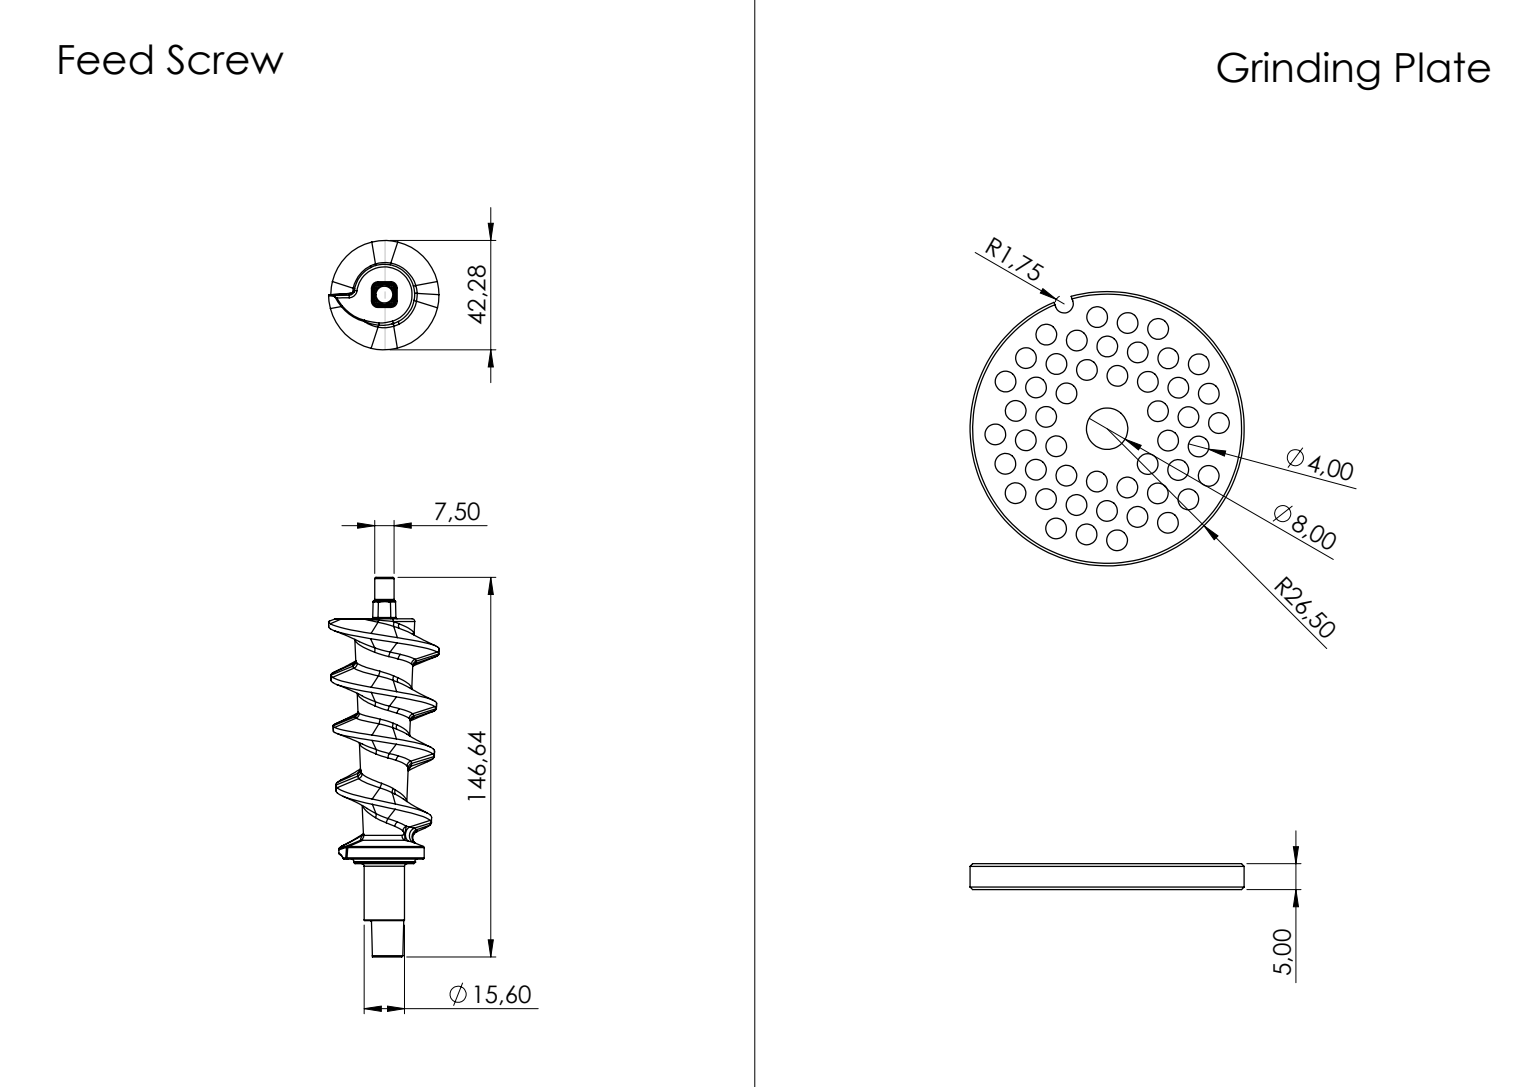
ISO-10303-21;
HEADER;
FILE_DESCRIPTION (('STEP AP214'),
    '1' );
FILE_NAME ('Grinding Plate.step',
    '2026-10-06T09:49:54',
    ( '' ),
    ( '' ),
    'SwSTEP 2.0',
    'SolidWorks 2020',
    '' );
FILE_SCHEMA (( 'AUTOMOTIVE_DESIGN' ));
ENDSEC;

DATA;
#6=DIRECTION ( 'NONE',  ( -0.6736849260863841948, 0.000000000000000000, 0.7390186874254148774 ) ) ;
#19=DIRECTION ( 'NONE',  ( 0.9858563016923833633, 0.000000000000000000, 0.1675928173085483863 ) ) ;
#20=ORIENTED_EDGE ( 'NONE', *, *, #50403, .T. ) ;
#27=ORIENTED_EDGE ( 'NONE', *, *, #23843, .F. ) ;
#32=EDGE_CURVE ( 'NONE', #37900, #21516, #96808, .T. ) ;
#63=CYLINDRICAL_SURFACE ( 'NONE', #4748, 2.000000000000003553 ) ;
#99=DIRECTION ( 'NONE',  ( 0.9858563016923833633, 0.000000000000000000, 0.1675928173085483863 ) ) ;
#119=DIRECTION ( 'NONE',  ( -5.980589973904019347E-17, 1.000000000000000000, -1.736889445713099699E-16 ) ) ;
#130=DIRECTION ( 'NONE',  ( -0.6736849260863839728, 0.000000000000000000, 0.7390186874254150995 ) ) ;
#163=CARTESIAN_POINT ( 'NONE',  ( -6.501609782144661231, 1517.151704408390060, 200.8207946853451631 ) ) ;
#210=FACE_BOUND ( 'NONE', #98928, .T. ) ;
#217=EDGE_LOOP ( 'NONE', ( #25668, #43396, #24555, #73471 ) ) ;
#228=DIRECTION ( 'NONE',  ( -0.6736849260863839728, 0.000000000000000000, 0.7390186874254150995 ) ) ;
#238=EDGE_CURVE ( 'NONE', #55027, #57510, #22026, .T. ) ;
#241=CARTESIAN_POINT ( 'NONE',  ( -9.862951377749247683, 1522.051704408389924, 228.3939896778649654 ) ) ;
#262=DIRECTION ( 'NONE',  ( 1.755985294532464991E-16, -1.000000000000000000, 1.338183447452830017E-16 ) ) ;
#294=CARTESIAN_POINT ( 'NONE',  ( -19.66678637224480397, 1519.551704408389924, 215.8936635741279986 ) ) ;
#310=CARTESIAN_POINT ( 'NONE',  ( -19.02974267272306719, 1517.051704408389924, 207.1627782414018100 ) ) ;
#365=VERTEX_POINT ( 'NONE', #20997 ) ;
#367=AXIS2_PLACEMENT_3D ( 'NONE', #81942, #5812, #24233 ) ;
#373=FACE_OUTER_BOUND ( 'NONE', #57009, .T. ) ;
#399=EDGE_CURVE ( 'NONE', #104547, #81525, #8616, .T. ) ;
#413=CARTESIAN_POINT ( 'NONE',  ( -6.954065720117950100, 1517.051704408389924, 183.5505540514350002 ) ) ;
#427=DIRECTION ( 'NONE',  ( -0.6736849260863839728, 0.000000000000000000, 0.7390186874254150995 ) ) ;
#428=DIRECTION ( 'NONE',  ( -1.755985294532469921E-16, 1.000000000000000000, -1.338183447452831989E-16 ) ) ;
#451=EDGE_LOOP ( 'NONE', ( #81291, #94235, #88373, #80457, #8593 ) ) ;
#471=AXIS2_PLACEMENT_3D ( 'NONE', #413, #34530, #58646 ) ;
#507=CARTESIAN_POINT ( 'NONE',  ( -9.786977751178733698, 1521.951704408389787, 191.2793932888540951 ) ) ;
#512=DIRECTION ( 'NONE',  ( -1.964544591288419982E-14, -1.000000000000000000, 8.043425993822650894E-15 ) ) ;
#532=DIRECTION ( 'NONE',  ( 0.9858563016923833633, 0.000000000000000000, 0.1675928173085483863 ) ) ;
#595=ORIENTED_EDGE ( 'NONE', *, *, #3501, .F. ) ;
#597=CARTESIAN_POINT ( 'NONE',  ( -7.271052316819549333, 1522.051704408389924, 225.3404165491008371 ) ) ;
#600=ORIENTED_EDGE ( 'NONE', *, *, #74040, .T. ) ;
#619=ORIENTED_EDGE ( 'NONE', *, *, #18010, .T. ) ;
#620=ADVANCED_FACE ( 'NONE', ( #78041 ), #85891, .F. ) ;
#634=SHAPE_DEFINITION_REPRESENTATION ( #5341, #72299 ) ;
#648=FACE_OUTER_BOUND ( 'NONE', #91311, .T. ) ;
#709=EDGE_CURVE ( 'NONE', #103300, #104414, #52050, .T. ) ;
#711=EDGE_CURVE ( 'NONE', #77569, #52731, #30620, .T. ) ;
#721=DIRECTION ( 'NONE',  ( 5.980589973904019347E-17, -1.000000000000000000, 1.736889445713099699E-16 ) ) ;
#743=DIRECTION ( 'NONE',  ( 1.755985294532469921E-16, -1.000000000000000000, 1.338183447452831989E-16 ) ) ;
#746=VECTOR ( 'NONE', #79973, 1000.000000000000000 ) ;
#771=ADVANCED_FACE ( 'NONE', ( #97611 ), #2481, .F. ) ;
#806=LINE ( 'NONE', #8072, #30643 ) ;
#832=EDGE_CURVE ( 'NONE', #43055, #13291, #18048, .T. ) ;
#860=AXIS2_PLACEMENT_3D ( 'NONE', #53375, #104309, #3530 ) ;
#871=VECTOR ( 'NONE', #57828, 1000.000000000000000 ) ;
#886=FACE_BOUND ( 'NONE', #41380, .T. ) ;
#910=ORIENTED_EDGE ( 'NONE', *, *, #106899, .T. ) ;
#914=CIRCLE ( 'NONE', #22271, 1.999999999999997780 ) ;
#999=ORIENTED_EDGE ( 'NONE', *, *, #53098, .T. ) ;
#1004=VERTEX_POINT ( 'NONE', #56242 ) ;
#1012=DIRECTION ( 'NONE',  ( -5.980589973904019347E-17, 1.000000000000000000, -1.736889445713099699E-16 ) ) ;
#1044=ORIENTED_EDGE ( 'NONE', *, *, #84247, .F. ) ;
#1077=VERTEX_POINT ( 'NONE', #18891 ) ;
#1134=EDGE_LOOP ( 'NONE', ( #19550, #98250, #54353, #73848 ) ) ;
#1145=EDGE_CURVE ( 'NONE', #38215, #32285, #36581, .T. ) ;
#1157=CYLINDRICAL_SURFACE ( 'NONE', #96556, 2.000000000000003553 ) ;
#1167=CARTESIAN_POINT ( 'NONE',  ( 3.897009773650441211, 1519.551704408389924, 231.0205787112126075 ) ) ;
#1269=LINE ( 'NONE', #35408, #31651 ) ;
#1351=DIRECTION ( 'NONE',  ( -1.755985294532469921E-16, 1.000000000000000000, -1.338183447452831989E-16 ) ) ;
#1368=CIRCLE ( 'NONE', #63973, 1.999999999999997780 ) ;
#1416=VECTOR ( 'NONE', #69193, 1000.000000000000000 ) ;
#1425=ORIENTED_EDGE ( 'NONE', *, *, #92483, .T. ) ;
#1443=VECTOR ( 'NONE', #3619, 1000.000000000000000 ) ;
#1447=VECTOR ( 'NONE', #59102, 1000.000000000000000 ) ;
#1455=CIRCLE ( 'NONE', #51483, 1.999999999999997780 ) ;
#1474=DIRECTION ( 'NONE',  ( -0.6736849260863841948, 0.000000000000000000, 0.7390186874254148774 ) ) ;
#1490=VERTEX_POINT ( 'NONE', #17960 ) ;
#1505=DIRECTION ( 'NONE',  ( -0.9455185755993178454, 0.000000000000000000, 0.3255681544571539243 ) ) ;
#1524=DIRECTION ( 'NONE',  ( 0.9455185755993178454, 0.000000000000000000, -0.3255681544571537578 ) ) ;
#1534=DIRECTION ( 'NONE',  ( 0.9858563016923833633, 0.000000000000000000, 0.1675928173085483863 ) ) ;
#1548=DIRECTION ( 'NONE',  ( 0.9455185755993178454, 0.000000000000000000, -0.3255681544571537578 ) ) ;
#1552=DIRECTION ( 'NONE',  ( -1.755985294532469921E-16, 1.000000000000000000, -1.338183447452831989E-16 ) ) ;
#1577=CARTESIAN_POINT ( 'NONE',  ( -11.81780673814840021, 1517.051704408389924, 222.7166774759110126 ) ) ;
#1585=VERTEX_POINT ( 'NONE', #48716 ) ;
#1595=CYLINDRICAL_SURFACE ( 'NONE', #11642, 2.000000000000003553 ) ;
#1596=DIRECTION ( 'NONE',  ( -0.6736849260863841948, 0.000000000000000000, 0.7390186874254148774 ) ) ;
#1633=DIRECTION ( 'NONE',  ( -0.6736849260863841948, 0.000000000000000000, 0.7390186874254148774 ) ) ;
#1642=DIRECTION ( 'NONE',  ( -1.755985294532469921E-16, 1.000000000000000000, -1.338183447452831989E-16 ) ) ;
#1649=EDGE_LOOP ( 'NONE', ( #99391, #52672, #101833, #73552 ) ) ;
#1650=DIRECTION ( 'NONE',  ( 1.755985294532469921E-16, -1.000000000000000000, 1.338183447452831989E-16 ) ) ;
#1667=CIRCLE ( 'NONE', #48101, 1.999999999999998668 ) ;
#1720=CARTESIAN_POINT ( 'NONE',  ( -15.69795926999090163, 1517.151704408390060, 195.4758181584410011 ) ) ;
#1747=EDGE_CURVE ( 'NONE', #43414, #35107, #74345, .T. ) ;
#1792=CARTESIAN_POINT ( 'NONE',  ( -21.63849897568203673, 1519.551704408389924, 215.5584779398195678 ) ) ;
#1822=AXIS2_PLACEMENT_3D ( 'NONE', #75535, #15573, #83352 ) ;
#1827=ORIENTED_EDGE ( 'NONE', *, *, #23117, .T. ) ;
#1848=CIRCLE ( 'NONE', #64422, 1.999999999999998668 ) ;
#1850=DIRECTION ( 'NONE',  ( -0.9455185755993178454, 0.000000000000000000, 0.3255681544571537578 ) ) ;
#1859=DIRECTION ( 'NONE',  ( -1.755985294532469921E-16, 1.000000000000000000, -1.338183447452831989E-16 ) ) ;
#1860=CONICAL_SURFACE ( 'NONE', #23233, 1.000000000000007327, 0.7853981633970000820 ) ;
#1868=AXIS2_PLACEMENT_3D ( 'NONE', #1577, #95621, #69899 ) ;
#1956=CARTESIAN_POINT ( 'NONE',  ( 21.62164173326539895, 1519.551704408389924, 208.0273405521070060 ) ) ;
#1961=CIRCLE ( 'NONE', #12873, 1.999999999999998668 ) ;
#1962=DIRECTION ( 'NONE',  ( -1.755985294532464991E-16, 1.000000000000000000, -1.338183447452830017E-16 ) ) ;
#1983=ORIENTED_EDGE ( 'NONE', *, *, #38974, .T. ) ;
#2000=ORIENTED_EDGE ( 'NONE', *, *, #5665, .F. ) ;
#2045=CIRCLE ( 'NONE', #64625, 2.000000000000003109 ) ;
#2052=ORIENTED_EDGE ( 'NONE', *, *, #13448, .F. ) ;
#2076=DIRECTION ( 'NONE',  ( 1.755985294532469921E-16, -1.000000000000000000, 1.338183447452831989E-16 ) ) ;
#2089=LINE ( 'NONE', #96684, #8615 ) ;
#2115=ORIENTED_EDGE ( 'NONE', *, *, #100899, .T. ) ;
#2153=ORIENTED_EDGE ( 'NONE', *, *, #64701, .T. ) ;
#2167=CIRCLE ( 'NONE', #36115, 1.999999999999998668 ) ;
#2172=ORIENTED_EDGE ( 'NONE', *, *, #97884, .T. ) ;
#2221=ADVANCED_FACE ( 'NONE', ( #43767 ), #11279, .F. ) ;
#2241=DIRECTION ( 'NONE',  ( -5.980589973904019347E-17, 1.000000000000000000, -1.736889445713099699E-16 ) ) ;
#2299=DIRECTION ( 'NONE',  ( -1.755985294532469921E-16, 1.000000000000000000, -1.338183447452831989E-16 ) ) ;
#2301=DIRECTION ( 'NONE',  ( -1.755985294532469921E-16, 1.000000000000000000, -1.338183447452831989E-16 ) ) ;
#2318=ADVANCED_FACE ( 'NONE', ( #87286 ), #107382, .F. ) ;
#2344=EDGE_CURVE ( 'NONE', #57510, #28393, #37987, .T. ) ;
#2356=ORIENTED_EDGE ( 'NONE', *, *, #32389, .T. ) ;
#2362=CARTESIAN_POINT ( 'NONE',  ( 10.47043688597563182, 1522.051704408389924, 197.0050518223378333 ) ) ;
#2378=DIRECTION ( 'NONE',  ( -0.6736849260863839728, 0.000000000000000000, 0.7390186874254150995 ) ) ;
#2384=EDGE_CURVE ( 'NONE', #41410, #69866, #97870, .T. ) ;
#2437=CYLINDRICAL_SURFACE ( 'NONE', #49131, 1.999999999999999556 ) ;
#2454=ORIENTED_EDGE ( 'NONE', *, *, #62551, .F. ) ;
#2468=ORIENTED_EDGE ( 'NONE', *, *, #61058, .F. ) ;
#2475=DIRECTION ( 'NONE',  ( 5.980589973904019347E-17, -1.000000000000000000, 1.736889445713099699E-16 ) ) ;
#2481=CYLINDRICAL_SURFACE ( 'NONE', #3800, 2.000000000000003109 ) ;
#2520=ORIENTED_EDGE ( 'NONE', *, *, #7279, .T. ) ;
#2526=DIRECTION ( 'NONE',  ( -0.6736849260863841948, 0.000000000000000000, 0.7390186874254148774 ) ) ;
#2578=ORIENTED_EDGE ( 'NONE', *, *, #35703, .F. ) ;
#2593=ORIENTED_EDGE ( 'NONE', *, *, #108261, .T. ) ;
#2596=CIRCLE ( 'NONE', #93734, 1.999999999999998668 ) ;
#2628=ORIENTED_EDGE ( 'NONE', *, *, #102846, .F. ) ;
#2629=DIRECTION ( 'NONE',  ( -1.755985294532469921E-16, 1.000000000000000000, -1.338183447452831989E-16 ) ) ;
#2630=DIRECTION ( 'NONE',  ( -5.980589973904019347E-17, 1.000000000000000000, -1.736889445713099699E-16 ) ) ;
#2644=ORIENTED_EDGE ( 'NONE', *, *, #20930, .T. ) ;
#2683=AXIS2_PLACEMENT_3D ( 'NONE', #72839, #63899, #54407 ) ;
#2689=DIRECTION ( 'NONE',  ( -1.755985294532469921E-16, 1.000000000000000000, -1.338183447452831989E-16 ) ) ;
#2707=FACE_OUTER_BOUND ( 'NONE', #62290, .T. ) ;
#2741=CARTESIAN_POINT ( 'NONE',  ( -5.940539704407486354, 1521.951704408389787, 229.2045057395878871 ) ) ;
#2743=ORIENTED_EDGE ( 'NONE', *, *, #15924, .T. ) ;
#2746=EDGE_CURVE ( 'NONE', #82445, #48574, #85257, .T. ) ;
#2764=VECTOR ( 'NONE', #6624, 1000.000000000000000 ) ;
#2798=ORIENTED_EDGE ( 'NONE', *, *, #52789, .T. ) ;
#2799=AXIS2_PLACEMENT_3D ( 'NONE', #81723, #3960, #12877 ) ;
#2807=CARTESIAN_POINT ( 'NONE',  ( 7.271052316819548444, 1522.051704408389924, 192.9032753742981470 ) ) ;
#2884=DIRECTION ( 'NONE',  ( 0.9858563016923833633, 0.000000000000000000, 0.1675928173085483863 ) ) ;
#2950=AXIS2_PLACEMENT_3D ( 'NONE', #40990, #76253, #75169 ) ;
#2955=CARTESIAN_POINT ( 'NONE',  ( -2.621457251404222255, 1519.551704408389924, 228.0616540033011574 ) ) ;
#2971=EDGE_CURVE ( 'NONE', #6947, #108856, #31094, .T. ) ;
#2988=EDGE_CURVE ( 'NONE', #20697, #36071, #48476, .T. ) ;
#3048=CARTESIAN_POINT ( 'NONE',  ( -21.60894078472486868, 1517.051704408389924, 199.6722430288449175 ) ) ;
#3095=CARTESIAN_POINT ( 'NONE',  ( -2.562340869413342048, 1522.051704408389924, 196.2891841806521711 ) ) ;
#3099=CIRCLE ( 'NONE', #17334, 1.999999999999999556 ) ;
#3107=VERTEX_POINT ( 'NONE', #106040 ) ;
#3128=ORIENTED_EDGE ( 'NONE', *, *, #24699, .T. ) ;
#3139=EDGE_CURVE ( 'NONE', #70769, #106306, #40471, .T. ) ;
#3155=CIRCLE ( 'NONE', #72836, 1.999999999999998668 ) ;
#3177=VECTOR ( 'NONE', #85229, 1000.000000000000000 ) ;
#3203=CIRCLE ( 'NONE', #6681, 1.999999999999999556 ) ;
#3222=ORIENTED_EDGE ( 'NONE', *, *, #102846, .T. ) ;
#3264=ORIENTED_EDGE ( 'NONE', *, *, #59650, .F. ) ;
#3450=DIRECTION ( 'NONE',  ( 1.755985294532469921E-16, -1.000000000000000000, 1.338183447452831989E-16 ) ) ;
#3455=DIRECTION ( 'NONE',  ( -0.6736849260863841948, 0.000000000000000000, 0.7390186874254148774 ) ) ;
#3468=AXIS2_PLACEMENT_3D ( 'NONE', #34859, #94767, #69046 ) ;
#3471=CYLINDRICAL_SURFACE ( 'NONE', #29822, 1.999999999999999556 ) ;
#3472=FACE_OUTER_BOUND ( 'NONE', #58106, .T. ) ;
#3501=EDGE_CURVE ( 'NONE', #90277, #63160, #6599, .T. ) ;
#3530=DIRECTION ( 'NONE',  ( -0.6736849260863841948, 0.000000000000000000, 0.7390186874254148774 ) ) ;
#3536=AXIS2_PLACEMENT_3D ( 'NONE', #106492, #105958, #29236 ) ;
#3552=ORIENTED_EDGE ( 'NONE', *, *, #50922, .F. ) ;
#3619=DIRECTION ( 'NONE',  ( -1.755985294532469921E-16, 1.000000000000000000, -1.338183447452831989E-16 ) ) ;
#3648=EDGE_CURVE ( 'NONE', #55027, #58309, #2089, .T. ) ;
#3657=EDGE_CURVE ( 'NONE', #3107, #87558, #71252, .T. ) ;
#3679=EDGE_LOOP ( 'NONE', ( #18940, #40964, #10687, #106527, #99518 ) ) ;
#3683=DIRECTION ( 'NONE',  ( -1.755985294532469921E-16, 1.000000000000000000, -1.338183447452831989E-16 ) ) ;
#3714=DIRECTION ( 'NONE',  ( -5.980589973904019347E-17, 1.000000000000000000, -1.736889445713099699E-16 ) ) ;
#3727=DIRECTION ( 'NONE',  ( -0.6736849260863839728, 0.000000000000000000, 0.7390186874254150995 ) ) ;
#3732=ORIENTED_EDGE ( 'NONE', *, *, #44116, .F. ) ;
#3738=AXIS2_PLACEMENT_3D ( 'NONE', #51329, #16589, #77104 ) ;
#3768=ADVANCED_FACE ( 'NONE', ( #87002 ), #11419, .F. ) ;
#3770=VERTEX_POINT ( 'NONE', #37164 ) ;
#3771=ORIENTED_EDGE ( 'NONE', *, *, #24131, .F. ) ;
#3777=EDGE_CURVE ( 'NONE', #20783, #98304, #62963, .T. ) ;
#3793=ORIENTED_EDGE ( 'NONE', *, *, #92766, .T. ) ;
#3794=ORIENTED_EDGE ( 'NONE', *, *, #5777, .T. ) ;
#3800=AXIS2_PLACEMENT_3D ( 'NONE', #88123, #46679, #72424 ) ;
#3804=DIRECTION ( 'NONE',  ( -0.6736849260863841948, 0.000000000000000000, 0.7390186874254148774 ) ) ;
#3812=ORIENTED_EDGE ( 'NONE', *, *, #98933, .F. ) ;
#3820=CARTESIAN_POINT ( 'NONE',  ( 11.75869035672759999, 1522.051704408389924, 227.2994842695800060 ) ) ;
#3826=ORIENTED_EDGE ( 'NONE', *, *, #68263, .F. ) ;
#3851=CARTESIAN_POINT ( 'NONE',  ( 15.69795926444620271, 1519.551704408389924, 222.7678737639049871 ) ) ;
#3893=CIRCLE ( 'NONE', #64637, 1.999999999999999556 ) ;
#3905=CARTESIAN_POINT ( 'NONE',  ( -9.803834995107230554, 1517.151704408390060, 196.6215198571080123 ) ) ;
#3914=EDGE_CURVE ( 'NONE', #42052, #70558, #6856, .T. ) ;
#3924=CARTESIAN_POINT ( 'NONE',  ( -7.878537825433329367, 1522.051704408389924, 218.1850669711710111 ) ) ;
#3955=VERTEX_POINT ( 'NONE', #1792 ) ;
#3956=AXIS2_PLACEMENT_3D ( 'NONE', #18061, #95892, #34874 ) ;
#3960=DIRECTION ( 'NONE',  ( 1.755985294532464991E-16, -1.000000000000000000, 1.338183447452830017E-16 ) ) ;
#3965=EDGE_LOOP ( 'NONE', ( #93778, #97741 ) ) ;
#3970=CIRCLE ( 'NONE', #14650, 2.000000000000003553 ) ;
#4069=EDGE_LOOP ( 'NONE', ( #72525, #55858, #37367, #105994, #72756 ) ) ;
#4131=CARTESIAN_POINT ( 'NONE',  ( 13.10606020890036838, 1522.051704408389924, 225.8214468947291493 ) ) ;
#4149=DIRECTION ( 'NONE',  ( -5.980589973904019347E-17, 1.000000000000000000, -1.736889445713099699E-16 ) ) ;
#4156=ORIENTED_EDGE ( 'NONE', *, *, #71920, .F. ) ;
#4223=DIRECTION ( 'NONE',  ( 1.755985294532469921E-16, -1.000000000000000000, 1.338183447452831989E-16 ) ) ;
#4248=FACE_OUTER_BOUND ( 'NONE', #102284, .T. ) ;
#4284=CIRCLE ( 'NONE', #32863, 1.999999999999999556 ) ;
#4287=DIRECTION ( 'NONE',  ( 5.980589973904019347E-17, -1.000000000000000000, 1.736889445713099699E-16 ) ) ;
#4305=VERTEX_POINT ( 'NONE', #28905 ) ;
#4328=ADVANCED_FACE ( 'NONE', ( #37307 ), #105058, .F. ) ;
#4340=ORIENTED_EDGE ( 'NONE', *, *, #37161, .T. ) ;
#4344=ORIENTED_EDGE ( 'NONE', *, *, #78141, .T. ) ;
#4386=CARTESIAN_POINT ( 'NONE',  ( -2.694739704345539888, 1517.151704408390060, 212.0779207114006510 ) ) ;
#4407=CARTESIAN_POINT ( 'NONE',  ( 7.271052316819548444, 1517.051704408389924, 192.9032753742981470 ) ) ;
#4486=DIRECTION ( 'NONE',  ( -1.755985294532469921E-16, 1.000000000000000000, -1.338183447452831989E-16 ) ) ;
#4521=DIRECTION ( 'NONE',  ( 5.980589973904019347E-17, -1.000000000000000000, 1.736889445713099699E-16 ) ) ;
#4577=CYLINDRICAL_SURFACE ( 'NONE', #87806, 2.000000000000003109 ) ;
#4600=ORIENTED_EDGE ( 'NONE', *, *, #107012, .F. ) ;
#4662=DIRECTION ( 'NONE',  ( 1.755985294532464991E-16, -1.000000000000000000, 1.338183447452830017E-16 ) ) ;
#4664=ORIENTED_EDGE ( 'NONE', *, *, #17540, .F. ) ;
#4694=CARTESIAN_POINT ( 'NONE',  ( 19.64992912776053657, 1517.051704408389924, 207.6921549199338983 ) ) ;
#4704=ORIENTED_EDGE ( 'NONE', *, *, #86424, .F. ) ;
#4735=DIRECTION ( 'NONE',  ( -0.9455185755993177343, 0.000000000000000000, 0.3255681544571540909 ) ) ;
#4745=CYLINDRICAL_SURFACE ( 'NONE', #5170, 2.000000000000003553 ) ;
#4748=AXIS2_PLACEMENT_3D ( 'NONE', #78412, #102486, #43707 ) ;
#4755=VERTEX_POINT ( 'NONE', #32752 ) ;
#4779=CARTESIAN_POINT ( 'NONE',  ( -9.862951377749247683, 1519.551704408389924, 228.3939896778649654 ) ) ;
#4781=CARTESIAN_POINT ( 'NONE',  ( 17.04532911661897288, 1517.151704408390060, 221.2898363890541589 ) ) ;
#4812=EDGE_CURVE ( 'NONE', #110694, #92620, #72829, .T. ) ;
#4830=ORIENTED_EDGE ( 'NONE', *, *, #2384, .F. ) ;
#4852=CYLINDRICAL_SURFACE ( 'NONE', #83731, 1.999999999999999556 ) ;
#4892=EDGE_LOOP ( 'NONE', ( #85187, #54785, #37181, #64258, #94394 ) ) ;
#4998=DIRECTION ( 'NONE',  ( -1.755985294532469921E-16, 1.000000000000000000, -1.338183447452831989E-16 ) ) ;
#5015=DIRECTION ( 'NONE',  ( 1.755985294532464991E-16, -1.000000000000000000, 1.338183447452830017E-16 ) ) ;
#5024=CARTESIAN_POINT ( 'NONE',  ( -20.98459803374076671, 1522.051704408389924, 201.4854660376508377 ) ) ;
#5026=VECTOR ( 'NONE', #83048, 1000.000000000000114 ) ;
#5071=DIRECTION ( 'NONE',  ( -5.980589973904019347E-17, 1.000000000000000000, -1.736889445713099699E-16 ) ) ;
#5075=EDGE_CURVE ( 'NONE', #8045, #31574, #41588, .T. ) ;
#5096=ORIENTED_EDGE ( 'NONE', *, *, #71920, .T. ) ;
#5103=CIRCLE ( 'NONE', #103491, 1.999999999999997780 ) ;
#5135=EDGE_CURVE ( 'NONE', #85592, #22264, #60356, .T. ) ;
#5144=EDGE_LOOP ( 'NONE', ( #76940, #42317, #64742, #2628, #47320 ) ) ;
#5162=VERTEX_POINT ( 'NONE', #106445 ) ;
#5168=DIRECTION ( 'NONE',  ( -5.980589973904019347E-17, 1.000000000000000000, -1.736889445713099699E-16 ) ) ;
#5170=AXIS2_PLACEMENT_3D ( 'NONE', #62071, #47861, #81434 ) ;
#5175=ADVANCED_FACE ( 'NONE', ( #72852 ), #46562, .F. ) ;
#5179=DIRECTION ( 'NONE',  ( -1.755985294532469921E-16, 1.000000000000000000, -1.338183447452831989E-16 ) ) ;
#5204=AXIS2_PLACEMENT_3D ( 'NONE', #24042, #8355, #68860 ) ;
#5231=DIRECTION ( 'NONE',  ( -1.755985294532469921E-16, 1.000000000000000000, -1.338183447452831989E-16 ) ) ;
#5240=CARTESIAN_POINT ( 'NONE',  ( -19.64992913029231403, 1519.551704408389924, 210.5515370058381279 ) ) ;
#5294=ORIENTED_EDGE ( 'NONE', *, *, #58517, .T. ) ;
#5341=PRODUCT_DEFINITION_SHAPE ( 'NONE', 'NONE',  #93161 ) ;
#5345=DIRECTION ( 'NONE',  ( 1.755985294532469921E-16, -1.000000000000000000, 1.338183447452831989E-16 ) ) ;
#5369=ORIENTED_EDGE ( 'NONE', *, *, #109924, .F. ) ;
#5372=DIRECTION ( 'NONE',  ( -1.755985294532469921E-16, 1.000000000000000000, -1.338183447452831989E-16 ) ) ;
#5486=EDGE_CURVE ( 'NONE', #81391, #100544, #1368, .T. ) ;
#5497=CARTESIAN_POINT ( 'NONE',  ( 5.923682464646780943, 1517.151704408390060, 194.3813127491490036 ) ) ;
#5506=DIRECTION ( 'NONE',  ( -1.755985294532469921E-16, 1.000000000000000000, -1.338183447452831989E-16 ) ) ;
#5562=CYLINDRICAL_SURFACE ( 'NONE', #30522, 2.000000000000003109 ) ;
#5599=CLOSED_SHELL ( 'NONE', ( #96938, #24061, #27007, #21181, #95044, #42222, #31748, #84990, #66105, #15986, #78832, #105611, #9693, #47464, #96441, #57134, #95527, #73378, #69362, #41149, #59645, #20154, #8989, #60806, #56963, #71224, #11391, #50751, #23310, #57672, #99363, #78459, #69555, #48000, #55987, #66999, #61806, #19362, #102319, #70587, #83469, #22197, #76059, #10075, #16727, #19263, #92537, #84237, #101278, #4328, #28941, #65806, #64116, #32565, #58366, #101310, #48745, #27494, #21540, #48765, #2318, #72324, #52788, #93107, #13462, #91394, #72125, #63168, #87992, #41597, #48623, #30912, #13186, #49423, #47605, #30257, #9196, #16734, #20439, #27756, #81449, #110377, #27011, #108348, #63755, #15866, #35213, #36382, #107664, #109982, #87124, #26759, #13816, #5175, #104836, #102164, #76276, #74830, #30311, #52793, #37664, #98830, #102964, #54643, #88843, #84779, #99574, #82543, #2221, #3768, #21272, #66596, #76262, #21664, #19989, #80982, #771, #15078, #88570, #77472, #85641, #58210, #97263, #97920, #32326, #620, #79124, #103589, #66134, #70497, #95510, #74653, #22326, #24667, #80630, #42693, #100116, #12589, #83130, #108285, #28154, #25589, #73272, #42319, #82177 ) ) ;
#5621=ORIENTED_EDGE ( 'NONE', *, *, #12480, .F. ) ;
#5646=FACE_OUTER_BOUND ( 'NONE', #74460, .T. ) ;
#5665=EDGE_CURVE ( 'NONE', #365, #93138, #21166, .T. ) ;
#5668=DIRECTION ( 'NONE',  ( -5.980589973904019347E-17, 1.000000000000000000, -1.736889445713099699E-16 ) ) ;
#5701=VECTOR ( 'NONE', #54056, 1000.000000000000000 ) ;
#5712=CARTESIAN_POINT ( 'NONE',  ( 18.31941652029302858, 1519.551704408389924, 203.8280657238408651 ) ) ;
#5718=CIRCLE ( 'NONE', #61218, 2.000000000000003553 ) ;
#5777=EDGE_CURVE ( 'NONE', #86539, #59011, #70285, .T. ) ;
#5812=DIRECTION ( 'NONE',  ( 1.755985294532469921E-16, -1.000000000000000000, 1.338183447452831989E-16 ) ) ;
#5815=AXIS2_PLACEMENT_3D ( 'NONE', #89895, #106692, #108911 ) ;
#5836=FACE_BOUND ( 'NONE', #97963, .T. ) ;
#5911=ORIENTED_EDGE ( 'NONE', *, *, #92691, .F. ) ;
#5918=( BOUNDED_CURVE ( )  B_SPLINE_CURVE ( 2, ( #99780, #55622, #89198 ),
 .UNSPECIFIED., .F., .T. ) 
 B_SPLINE_CURVE_WITH_KNOTS ( ( 3, 3 ),
 ( 0.1572692979053489926, 0.2337410564013850112 ),
 .UNSPECIFIED. ) 
 CURVE ( )  GEOMETRIC_REPRESENTATION_ITEM ( )  RATIONAL_B_SPLINE_CURVE ( ( 1.002044729868130091, 1.002448067003099963, 1.002760198777220113 ) ) 
 REPRESENTATION_ITEM ( '' )  );
#5929=CARTESIAN_POINT ( 'NONE',  ( 15.69795926444620271, 1519.551704408389924, 222.7678737639049871 ) ) ;
#5995=DIRECTION ( 'NONE',  ( -5.980589973904019347E-17, 1.000000000000000000, -1.736889445713099699E-16 ) ) ;
#5998=EDGE_LOOP ( 'NONE', ( #90814, #20701, #47201, #91238, #70087 ) ) ;
#6024=CYLINDRICAL_SURFACE ( 'NONE', #32104, 2.000000000000003553 ) ;
#6074=CARTESIAN_POINT ( 'NONE',  ( 5.864566082395450408, 1517.051704408389924, 226.1537825710409777 ) ) ;
#6086=CIRCLE ( 'NONE', #13177, 1.999999999999999556 ) ;
#6097=LINE ( 'NONE', #49227, #50092 ) ;
#6177=LINE ( 'NONE', #74511, #23361 ) ;
#6235=ORIENTED_EDGE ( 'NONE', *, *, #80260, .F. ) ;
#6266=EDGE_CURVE ( 'NONE', #64960, #108026, #19234, .T. ) ;
#6275=CIRCLE ( 'NONE', #68887, 1.999999999999999556 ) ;
#6349=LINE ( 'NONE', #90901, #52146 ) ;
#6419=VECTOR ( 'NONE', #67422, 1000.000000000000000 ) ;
#6420=ORIENTED_EDGE ( 'NONE', *, *, #107298, .T. ) ;
#6450=CARTESIAN_POINT ( 'NONE',  ( 2.562340869413348265, 1517.051704408389924, 221.9545077427458182 ) ) ;
#6458=EDGE_LOOP ( 'NONE', ( #60135, #15344, #107470, #40291, #89219, #32445 ) ) ;
#6526=AXIS2_PLACEMENT_3D ( 'NONE', #23608, #32574, #24142 ) ;
#6530=ORIENTED_EDGE ( 'NONE', *, *, #61639, .T. ) ;
#6537=DIRECTION ( 'NONE',  ( 5.980589973904019347E-17, -1.000000000000000000, 1.736889445713099699E-16 ) ) ;
#6541=ORIENTED_EDGE ( 'NONE', *, *, #93928, .F. ) ;
#6586=ORIENTED_EDGE ( 'NONE', *, *, #79455, .T. ) ;
#6592=CARTESIAN_POINT ( 'NONE',  ( 9.803834995107230554, 1517.151704408390060, 221.6221720662910002 ) ) ;
#6599=LINE ( 'NONE', #101185, #90869 ) ;
#6601=ORIENTED_EDGE ( 'NONE', *, *, #42077, .F. ) ;
#6617=EDGE_LOOP ( 'NONE', ( #84907, #22921 ) ) ;
#6624=DIRECTION ( 'NONE',  ( -1.755985294532469921E-16, 1.000000000000000000, -1.338183447452831989E-16 ) ) ;
#6671=DIRECTION ( 'NONE',  ( 0.9455185755993178454, 0.000000000000000000, -0.3255681544571539243 ) ) ;
#6681=AXIS2_PLACEMENT_3D ( 'NONE', #27841, #54173, #1548 ) ;
#6690=EDGE_CURVE ( 'NONE', #22976, #76210, #77968, .T. ) ;
#6743=ORIENTED_EDGE ( 'NONE', *, *, #107681, .F. ) ;
#6809=AXIS2_PLACEMENT_3D ( 'NONE', #15796, #75752, #109898 ) ;
#6823=LINE ( 'NONE', #40982, #25800 ) ;
#6827=CARTESIAN_POINT ( 'NONE',  ( -1.925297167936410148, 1517.051704408389924, 187.5582988455250018 ) ) ;
#6854=DIRECTION ( 'NONE',  ( 1.755985294532464991E-16, -1.000000000000000000, 1.338183447452830017E-16 ) ) ;
#6856=CIRCLE ( 'NONE', #36995, 2.000000000000003553 ) ;
#6860=CARTESIAN_POINT ( 'NONE',  ( 5.316196956075329716, 1517.151704408390060, 187.2259631713411636 ) ) ;
#6881=EDGE_CURVE ( 'NONE', #62929, #43414, #36882, .T. ) ;
#6887=CARTESIAN_POINT ( 'NONE',  ( -17.07488731192356823, 1517.051704408389924, 212.8400904445188075 ) ) ;
#6947=VERTEX_POINT ( 'NONE', #42352 ) ;
#6971=CARTESIAN_POINT ( 'NONE',  ( 19.63722818192610120, 1522.051704408389924, 218.2362632616380154 ) ) ;
#6997=DIRECTION ( 'NONE',  ( -0.9455185755993178454, 0.000000000000000000, 0.3255681544571539243 ) ) ;
#7055=CARTESIAN_POINT ( 'NONE',  ( 14.35058941227343077, 1519.551704408389924, 224.2459111387558437 ) ) ;
#7059=FACE_BOUND ( 'NONE', #66429, .T. ) ;
#7079=ORIENTED_EDGE ( 'NONE', *, *, #40772, .F. ) ;
#7092=ORIENTED_EDGE ( 'NONE', *, *, #89715, .F. ) ;
#7160=DIRECTION ( 'NONE',  ( 1.755985294532469921E-16, -1.000000000000000000, 1.338183447452831989E-16 ) ) ;
#7191=DIRECTION ( 'NONE',  ( 2.042903098301770100E-14, 1.000000000000000000, -6.143886524153290706E-15 ) ) ;
#7192=DIRECTION ( 'NONE',  ( -1.755985294532469921E-16, 1.000000000000000000, -1.338183447452831989E-16 ) ) ;
#7203=CARTESIAN_POINT ( 'NONE',  ( -13.77266209894789917, 1522.051704408389924, 217.0393652727940150 ) ) ;
#7217=FACE_OUTER_BOUND ( 'NONE', #98343, .T. ) ;
#7219=CYLINDRICAL_SURFACE ( 'NONE', #105204, 2.000000000000003109 ) ;
#7229=DIRECTION ( 'NONE',  ( -1.964544591288419982E-14, -1.000000000000000000, 8.043425993822650894E-15 ) ) ;
#7278=CARTESIAN_POINT ( 'NONE',  ( 9.833393186232889605, 1517.151704408390060, 205.7359371553449989 ) ) ;
#7279=EDGE_CURVE ( 'NONE', #79544, #79854, #42245, .T. ) ;
#7326=ORIENTED_EDGE ( 'NONE', *, *, #37919, .T. ) ;
#7360=DIRECTION ( 'NONE',  ( 0.9455185755993178454, 0.000000000000000000, -0.3255681544571539243 ) ) ;
#7380=EDGE_LOOP ( 'NONE', ( #81488, #45826 ) ) ;
#7400=CYLINDRICAL_SURFACE ( 'NONE', #95804, 2.000000000000003109 ) ;
#7417=CARTESIAN_POINT ( 'NONE',  ( 17.71193101166619854, 1517.151704408390060, 196.6727161458730109 ) ) ;
#7423=ORIENTED_EDGE ( 'NONE', *, *, #25343, .T. ) ;
#7436=EDGE_CURVE ( 'NONE', #31574, #106669, #67280, .T. ) ;
#7441=CARTESIAN_POINT ( 'NONE',  ( 3.968827104744170331, 1521.951704408389787, 188.7040005449509863 ) ) ;
#7475=FACE_BOUND ( 'NONE', #87948, .T. ) ;
#7505=DIRECTION ( 'NONE',  ( 1.755985294532464991E-16, -1.000000000000000000, 1.338183447452830017E-16 ) ) ;
#7548=CARTESIAN_POINT ( 'NONE',  ( 13.16517659032117038, 1517.151704408390060, 194.0489770726361485 ) ) ;
#7586=CARTESIAN_POINT ( 'NONE',  ( 17.66551557898246827, 1519.551704408389924, 217.9010776244259660 ) ) ;
#7603=FACE_BOUND ( 'NONE', #103983, .T. ) ;
#7626=ORIENTED_EDGE ( 'NONE', *, *, #78141, .F. ) ;
#7660=EDGE_LOOP ( 'NONE', ( #88905, #14828 ) ) ;
#7697=ORIENTED_EDGE ( 'NONE', *, *, #60037, .T. ) ;
#7746=LINE ( 'NONE', #92298, #103559 ) ;
#7766=FACE_OUTER_BOUND ( 'NONE', #19937, .T. ) ;
#7828=CARTESIAN_POINT ( 'NONE',  ( -6.790918657024139549, 1517.051704408389924, 184.0243675267330161 ) ) ;
#7845=CARTESIAN_POINT ( 'NONE',  ( 3.968827103902559550, 1519.551704408389924, 188.7040005461919918 ) ) ;
#7861=CIRCLE ( 'NONE', #36488, 1.999999999999998668 ) ;
#7886=ORIENTED_EDGE ( 'NONE', *, *, #89086, .T. ) ;
#7906=CARTESIAN_POINT ( 'NONE',  ( -1.925297170580940076, 1522.051704408389924, 187.5582988486569889 ) ) ;
#7950=DIRECTION ( 'NONE',  ( -0.6736849260863841948, 0.000000000000000000, 0.7390186874254148774 ) ) ;
#8021=FACE_BOUND ( 'NONE', #109025, .T. ) ;
#8025=VERTEX_POINT ( 'NONE', #18828 ) ;
#8045=VERTEX_POINT ( 'NONE', #59765 ) ;
#8072=CARTESIAN_POINT ( 'NONE',  ( -17.07488731192357179, 1517.151704408390060, 212.8400904445188075 ) ) ;
#8091=DIRECTION ( 'NONE',  ( 1.755985294532464991E-16, -1.000000000000000000, 1.338183447452830017E-16 ) ) ;
#8100=AXIS2_PLACEMENT_3D ( 'NONE', #32600, #85190, #109857 ) ;
#8132=CARTESIAN_POINT ( 'NONE',  ( -18.31941652021488665, 1519.551704408389924, 214.4156261991469421 ) ) ;
#8134=VERTEX_POINT ( 'NONE', #105629 ) ;
#8164=DIRECTION ( 'NONE',  ( 1.755985294532469921E-16, -1.000000000000000000, 1.338183447452831989E-16 ) ) ;
#8165=ORIENTED_EDGE ( 'NONE', *, *, #15362, .F. ) ;
#8213=EDGE_CURVE ( 'NONE', #42280, #39961, #49451, .T. ) ;
#8223=AXIS2_PLACEMENT_3D ( 'NONE', #105293, #10693, #17395 ) ;
#8283=EDGE_CURVE ( 'NONE', #54897, #71672, #24320, .T. ) ;
#8302=DIRECTION ( 'NONE',  ( 0.9858563016923833633, 0.000000000000000000, 0.1675928173085483863 ) ) ;
#8317=EDGE_LOOP ( 'NONE', ( #108206, #74502, #95926, #71184 ) ) ;
#8322=EDGE_LOOP ( 'NONE', ( #83112, #6235, #19977, #14053 ) ) ;
#8349=EDGE_CURVE ( 'NONE', #91497, #23258, #62011, .T. ) ;
#8352=DIRECTION ( 'NONE',  ( 0.9455185755993178454, 0.000000000000000000, -0.3255681544571537578 ) ) ;
#8355=DIRECTION ( 'NONE',  ( -1.755985294532469921E-16, 1.000000000000000000, -1.338183447452831989E-16 ) ) ;
#8358=DIRECTION ( 'NONE',  ( -1.755985294532469921E-16, 1.000000000000000000, -1.338183447452831989E-16 ) ) ;
#8376=AXIS2_PLACEMENT_3D ( 'NONE', #90181, #30835, #80706 ) ;
#8378=DIRECTION ( 'NONE',  ( -0.6736849260863841948, 0.000000000000000000, 0.7390186874254148774 ) ) ;
#8406=VERTEX_POINT ( 'NONE', #102384 ) ;
#8410=CARTESIAN_POINT ( 'NONE',  ( -0.04641543425164609826, 1521.951704408389787, 230.3502074417858978 ) ) ;
#8411=ORIENTED_EDGE ( 'NONE', *, *, #42579, .T. ) ;
#8434=VERTEX_POINT ( 'NONE', #59551 ) ;
#8440=DIRECTION ( 'NONE',  ( -1.755985294532469921E-16, 1.000000000000000000, -1.338183447452831989E-16 ) ) ;
#8450=CARTESIAN_POINT ( 'NONE',  ( -7.211935934568220574, 1517.151704408390060, 193.5679467272088345 ) ) ;
#8510=VECTOR ( 'NONE', #4287, 1000.000000000000000 ) ;
#8534=EDGE_CURVE ( 'NONE', #50989, #100544, #107051, .T. ) ;
#8569=DIRECTION ( 'NONE',  ( 1.755985294532469921E-16, -1.000000000000000000, 1.338183447452830017E-16 ) ) ;
#8582=DIRECTION ( 'NONE',  ( 1.755985294532464991E-16, -1.000000000000000000, 1.338183447452830017E-16 ) ) ;
#8588=DIRECTION ( 'NONE',  ( 1.755985294532469921E-16, -1.000000000000000000, 1.338183447452831989E-16 ) ) ;
#8593=ORIENTED_EDGE ( 'NONE', *, *, #44723, .F. ) ;
#8615=VECTOR ( 'NONE', #86611, 1000.000000000000000 ) ;
#8616=LINE ( 'NONE', #9733, #48463 ) ;
#8639=DIRECTION ( 'NONE',  ( -5.980589973904019347E-17, 1.000000000000000000, -1.736889445713099699E-16 ) ) ;
#8663=CARTESIAN_POINT ( 'NONE',  ( 21.62164173326539895, 1522.051704408389924, 208.0273405521070060 ) ) ;
#8669=CARTESIAN_POINT ( 'NONE',  ( 11.75869035672759999, 1517.151704408390060, 227.2994842695800060 ) ) ;
#8682=ORIENTED_EDGE ( 'NONE', *, *, #53997, .T. ) ;
#8696=AXIS2_PLACEMENT_3D ( 'NONE', #54348, #17936, #79534 ) ;
#8724=CIRCLE ( 'NONE', #26634, 1.999999999999997780 ) ;
#8741=LINE ( 'NONE', #76510, #58085 ) ;
#8756=AXIS2_PLACEMENT_3D ( 'NONE', #9855, #50756, #51874 ) ;
#8763=CARTESIAN_POINT ( 'NONE',  ( -21.62164173379369814, 1522.051704408389924, 210.2163513719069954 ) ) ;
#8775=AXIS2_PLACEMENT_3D ( 'NONE', #91608, #23832, #48525 ) ;
#8781=CARTESIAN_POINT ( 'NONE',  ( 22.96901158543816734, 1519.551704408389924, 206.5493031772561778 ) ) ;
#8794=DIRECTION ( 'NONE',  ( -0.6736849260863837507, 0.000000000000000000, 0.7390186874254154326 ) ) ;
#8804=CARTESIAN_POINT ( 'NONE',  ( -19.66678637246580053, 1521.951704408389787, 215.8936635744080093 ) ) ;
#8812=ORIENTED_EDGE ( 'NONE', *, *, #35253, .T. ) ;
#8834=DIRECTION ( 'NONE',  ( -0.9455185755993178454, 0.000000000000000000, 0.3255681544571537578 ) ) ;
#8887=CARTESIAN_POINT ( 'NONE',  ( -6.501609782144663896, 1522.051704408389924, 200.8207946853451631 ) ) ;
#8905=CARTESIAN_POINT ( 'NONE',  ( 9.833393186232889605, 1517.051704408389924, 205.7359371553449989 ) ) ;
#8945=ORIENTED_EDGE ( 'NONE', *, *, #64378, .T. ) ;
#8946=DIRECTION ( 'NONE',  ( 1.755985294532469921E-16, -1.000000000000000000, 1.338183447452831989E-16 ) ) ;
#8960=DIRECTION ( 'NONE',  ( -0.9455185755993178454, 0.000000000000000000, 0.3255681544571537578 ) ) ;
#8976=CARTESIAN_POINT ( 'NONE',  ( 10.47043688597563182, 1517.051704408389924, 197.0050518223378333 ) ) ;
#8989=ADVANCED_FACE ( 'NONE', ( #16806 ), #63, .F. ) ;
#9009=ORIENTED_EDGE ( 'NONE', *, *, #10940, .F. ) ;
#9033=VERTEX_POINT ( 'NONE', #103034 ) ;
#9044=CARTESIAN_POINT ( 'NONE',  ( -21.62164173379369814, 1522.051704408389924, 210.2163513719069954 ) ) ;
#9073=DIRECTION ( 'NONE',  ( -5.980589973904019347E-17, 1.000000000000000000, -1.736889445713099699E-16 ) ) ;
#9089=AXIS2_PLACEMENT_3D ( 'NONE', #58599, #92186, #68663 ) ;
#9118=CARTESIAN_POINT ( 'NONE',  ( 13.13561839920526886, 1517.051704408389924, 209.9352119836111683 ) ) ;
#9128=CYLINDRICAL_SURFACE ( 'NONE', #3956, 2.000000000000003109 ) ;
#9143=ORIENTED_EDGE ( 'NONE', *, *, #10415, .F. ) ;
#9158=CARTESIAN_POINT ( 'NONE',  ( -21.62164173379369814, 1519.551704408389924, 210.2163513719069954 ) ) ;
#9167=ORIENTED_EDGE ( 'NONE', *, *, #96517, .F. ) ;
#9174=AXIS2_PLACEMENT_3D ( 'NONE', #108504, #98985, #107949 ) ;
#9194=CARTESIAN_POINT ( 'NONE',  ( 19.66678637211940028, 1521.951704408389787, 202.3500283489059939 ) ) ;
#9196=ADVANCED_FACE ( 'NONE', ( #49781 ), #7219, .F. ) ;
#9200=EDGE_CURVE ( 'NONE', #42647, #23415, #12230, .T. ) ;
#9202=CARTESIAN_POINT ( 'NONE',  ( -8.456465142934458612, 1517.151704408390060, 195.1434824822571841 ) ) ;
#9206=VECTOR ( 'NONE', #65941, 1000.000000000000000 ) ;
#9250=AXIS2_PLACEMENT_3D ( 'NONE', #52199, #76835, #51089 ) ;
#9259=ORIENTED_EDGE ( 'NONE', *, *, #91873, .T. ) ;
#9269=FACE_BOUND ( 'NONE', #47033, .T. ) ;
#9274=ORIENTED_EDGE ( 'NONE', *, *, #31202, .F. ) ;
#9288=ORIENTED_EDGE ( 'NONE', *, *, #54322, .F. ) ;
#9309=( BOUNDED_CURVE ( )  B_SPLINE_CURVE ( 2, ( #96032, #68648, #62473 ),
 .UNSPECIFIED., .F., .T. ) 
 B_SPLINE_CURVE_WITH_KNOTS ( ( 3, 3 ),
 ( 0.1572692979053489926, 0.2337410564013850112 ),
 .UNSPECIFIED. ) 
 CURVE ( )  GEOMETRIC_REPRESENTATION_ITEM ( )  RATIONAL_B_SPLINE_CURVE ( ( 1.002044729868130091, 1.002448067003099963, 1.002760198777220113 ) ) 
 REPRESENTATION_ITEM ( '' )  );
#9328=AXIS2_PLACEMENT_3D ( 'NONE', #89705, #12986, #47169 ) ;
#9348=ORIENTED_EDGE ( 'NONE', *, *, #25465, .F. ) ;
#9419=ORIENTED_EDGE ( 'NONE', *, *, #81848, .F. ) ;
#9432=FACE_OUTER_BOUND ( 'NONE', #80516, .T. ) ;
#9456=ORIENTED_EDGE ( 'NONE', *, *, #45256, .T. ) ;
#9527=DIRECTION ( 'NONE',  ( -1.755985294532469921E-16, 1.000000000000000000, -1.338183447452831989E-16 ) ) ;
#9533=DIRECTION ( 'NONE',  ( -0.9455185755993178454, 0.000000000000000000, 0.3255681544571537578 ) ) ;
#9574=VERTEX_POINT ( 'NONE', #53099 ) ;
#9659=DIRECTION ( 'NONE',  ( 1.755985294532469921E-16, -1.000000000000000000, 1.338183447452831989E-16 ) ) ;
#9670=AXIS2_PLACEMENT_3D ( 'NONE', #30927, #13556, #81877 ) ;
#9676=FACE_BOUND ( 'NONE', #110772, .T. ) ;
#9693=ADVANCED_FACE ( 'NONE', ( #91641 ), #49109, .F. ) ;
#9699=EDGE_CURVE ( 'NONE', #76507, #8045, #25751, .T. ) ;
#9708=ORIENTED_EDGE ( 'NONE', *, *, #52348, .F. ) ;
#9733=CARTESIAN_POINT ( 'NONE',  ( 15.12003195112067111, 1517.151704408390060, 199.7262892757531745 ) ) ;
#9771=CARTESIAN_POINT ( 'NONE',  ( 9.862951377358559313, 1519.551704408389924, 189.8497022443989977 ) ) ;
#9787=CYLINDRICAL_SURFACE ( 'NONE', #94977, 2.000000000000002220 ) ;
#9807=EDGE_CURVE ( 'NONE', #63160, #70030, #7861, .T. ) ;
#9811=FACE_BOUND ( 'NONE', #91771, .T. ) ;
#9841=AXIS2_PLACEMENT_3D ( 'NONE', #57177, #48770, #75072 ) ;
#9851=DIRECTION ( 'NONE',  ( -1.755985294532469921E-16, 1.000000000000000000, -1.338183447452831989E-16 ) ) ;
#9855=CARTESIAN_POINT ( 'NONE',  ( 9.803834995107230554, 1522.051704408389924, 221.6221720662910002 ) ) ;
#9887=ORIENTED_EDGE ( 'NONE', *, *, #78622, .T. ) ;
#9905=DIRECTION ( 'NONE',  ( 1.755985294532464991E-16, -1.000000000000000000, 1.338183447452830017E-16 ) ) ;
#9912=CARTESIAN_POINT ( 'NONE',  ( -6.647330431358690284, 1519.551704408389924, 184.4413780136169976 ) ) ;
#9926=EDGE_CURVE ( 'NONE', #70320, #30342, #29781, .T. ) ;
#9936=CARTESIAN_POINT ( 'NONE',  ( 11.75869035456349998, 1517.051704408389924, 227.2994842691620079 ) ) ;
#9966=ORIENTED_EDGE ( 'NONE', *, *, #23721, .T. ) ;
#10020=DIRECTION ( 'NONE',  ( -0.9455185755993178454, 0.000000000000000000, 0.3255681544571537578 ) ) ;
#10028=AXIS2_PLACEMENT_3D ( 'NONE', #72051, #2630, #72576 ) ;
#10075=ADVANCED_FACE ( 'NONE', ( #98668 ), #75687, .F. ) ;
#10080=CARTESIAN_POINT ( 'NONE',  ( -13.13561839920526886, 1522.051704408389924, 208.3084799397878157 ) ) ;
#10087=CARTESIAN_POINT ( 'NONE',  ( 8.456465142934460388, 1522.051704408389924, 223.1002094411418284 ) ) ;
#10089=DIRECTION ( 'NONE',  ( -1.755985294532469921E-16, 1.000000000000000000, -1.338183447452831989E-16 ) ) ;
#10092=FACE_OUTER_BOUND ( 'NONE', #55577, .T. ) ;
#10094=DIRECTION ( 'NONE',  ( 5.980589973904019347E-17, -1.000000000000000000, 1.736889445713099699E-16 ) ) ;
#10108=EDGE_CURVE ( 'NONE', #63621, #79273, #58409, .T. ) ;
#10154=DIRECTION ( 'NONE',  ( -0.6736849260863841948, 0.000000000000000000, 0.7390186874254148774 ) ) ;
#10161=CIRCLE ( 'NONE', #60283, 1.999999999999999556 ) ;
#10167=VERTEX_POINT ( 'NONE', #100323 ) ;
#10189=CARTESIAN_POINT ( 'NONE',  ( 10.41132050455483160, 1522.051704408389924, 228.7775216444308342 ) ) ;
#10201=CIRCLE ( 'NONE', #31695, 2.000000000000003109 ) ;
#10208=DIRECTION ( 'NONE',  ( -0.6736849260863841948, 0.000000000000000000, 0.7390186874254148774 ) ) ;
#10212=DIRECTION ( 'NONE',  ( -0.6736849260863839728, 0.000000000000000000, 0.7390186874254150995 ) ) ;
#10247=CARTESIAN_POINT ( 'NONE',  ( 7.848979634317430509, 1522.051704408389924, 215.9448598632019980 ) ) ;
#10259=ORIENTED_EDGE ( 'NONE', *, *, #29592, .F. ) ;
#10262=DIRECTION ( 'NONE',  ( 1.755985294532464991E-16, -1.000000000000000000, 1.338183447452830017E-16 ) ) ;
#10303=EDGE_CURVE ( 'NONE', #48574, #82445, #54822, .T. ) ;
#10336=FACE_OUTER_BOUND ( 'NONE', #40350, .T. ) ;
#10402=FACE_OUTER_BOUND ( 'NONE', #40963, .T. ) ;
#10415=EDGE_CURVE ( 'NONE', #79870, #95724, #4284, .T. ) ;
#10427=EDGE_CURVE ( 'NONE', #77064, #46523, #89022, .T. ) ;
#10441=CARTESIAN_POINT ( 'NONE',  ( 0.02955819112566610354, 1517.051704408389924, 193.2356110507530218 ) ) ;
#10457=CARTESIAN_POINT ( 'NONE',  ( 0.02955819112566610354, 1517.051704408389924, 193.2356110507530218 ) ) ;
#10477=CIRCLE ( 'NONE', #26538, 1.999999999999998668 ) ;
#10498=AXIS2_PLACEMENT_3D ( 'NONE', #77449, #95897, #62330 ) ;
#10507=CARTESIAN_POINT ( 'NONE',  ( 5.940539707516006906, 1519.551704408389924, 189.0391861794638828 ) ) ;
#10525=EDGE_CURVE ( 'NONE', #40567, #36571, #27896, .T. ) ;
#10532=DIRECTION ( 'NONE',  ( -1.755985294532469921E-16, 1.000000000000000000, -1.338183447452831989E-16 ) ) ;
#10554=CIRCLE ( 'NONE', #30189, 26.00000000000000711 ) ;
#10555=CIRCLE ( 'NONE', #60705, 1.999999999999999556 ) ;
#10580=EDGE_CURVE ( 'NONE', #106306, #103193, #81148, .T. ) ;
#10587=LINE ( 'NONE', #44758, #108873 ) ;
#10608=AXIS2_PLACEMENT_3D ( 'NONE', #21325, #57742, #80719 ) ;
#10614=EDGE_CURVE ( 'NONE', #79550, #19461, #31191, .T. ) ;
#10621=AXIS2_PLACEMENT_3D ( 'NONE', #109777, #85660, #8960 ) ;
#10642=CARTESIAN_POINT ( 'NONE',  ( 21.62164173114529930, 1517.051704408389924, 208.0273405545509888 ) ) ;
#10655=DIRECTION ( 'NONE',  ( 1.755985294532464991E-16, -1.000000000000000000, 1.338183447452830017E-16 ) ) ;
#10675=CARTESIAN_POINT ( 'NONE',  ( -0.02955819112566620069, 1517.151704408390060, 225.0080808726450243 ) ) ;
#10687=ORIENTED_EDGE ( 'NONE', *, *, #13231, .F. ) ;
#10693=DIRECTION ( 'NONE',  ( -1.755985294532469921E-16, 1.000000000000000000, -1.338183447452831989E-16 ) ) ;
#10726=AXIS2_PLACEMENT_3D ( 'NONE', #9936, #1012, #45780 ) ;
#10758=EDGE_CURVE ( 'NONE', #65489, #99771, #71413, .T. ) ;
#10778=LINE ( 'NONE', #88050, #44800 ) ;
#10801=AXIS2_PLACEMENT_3D ( 'NONE', #92742, #101673, #66477 ) ;
#10806=ORIENTED_EDGE ( 'NONE', *, *, #90107, .T. ) ;
#10824=VERTEX_POINT ( 'NONE', #26084 ) ;
#10841=ORIENTED_EDGE ( 'NONE', *, *, #32, .F. ) ;
#10845=CIRCLE ( 'NONE', #73418, 1.999999999999998668 ) ;
#10870=CIRCLE ( 'NONE', #87680, 1.999999999999999556 ) ;
#10901=CIRCLE ( 'NONE', #57357, 1.999999999999999556 ) ;
#10903=CYLINDRICAL_SURFACE ( 'NONE', #83680, 2.000000000000003553 ) ;
#10926=FACE_BOUND ( 'NONE', #14362, .T. ) ;
#10927=CARTESIAN_POINT ( 'NONE',  ( -7.271052316819549333, 1517.051704408389924, 225.3404165491008371 ) ) ;
#10940=EDGE_CURVE ( 'NONE', #85274, #98761, #91012, .T. ) ;
#10941=DIRECTION ( 'NONE',  ( -5.980589973904019347E-17, 1.000000000000000000, -1.736889445713099699E-16 ) ) ;
#10942=DIRECTION ( 'NONE',  ( 0.9455185755993178454, 0.000000000000000000, -0.3255681544571537578 ) ) ;
#10971=CARTESIAN_POINT ( 'NONE',  ( -11.75869035857540013, 1519.551704408389924, 190.9442076533970010 ) ) ;
#10976=AXIS2_PLACEMENT_3D ( 'NONE', #84539, #86752, #6 ) ;
#11016=CARTESIAN_POINT ( 'NONE',  ( -9.862951376772540968, 1517.051704408389924, 228.3939896807019920 ) ) ;
#11028=DIRECTION ( 'NONE',  ( 1.755985294532469921E-16, -1.000000000000000000, 1.338183447452831989E-16 ) ) ;
#11057=DIRECTION ( 'NONE',  ( -1.755985294532469921E-16, 1.000000000000000000, -1.338183447452831989E-16 ) ) ;
#11074=CARTESIAN_POINT ( 'NONE',  ( -5.923682464646780943, 1517.151704408390060, 223.8623791742500089 ) ) ;
#11086=DIRECTION ( 'NONE',  ( -1.755985294532469921E-16, 1.000000000000000000, -1.338183447452831989E-16 ) ) ;
#11090=ORIENTED_EDGE ( 'NONE', *, *, #108679, .T. ) ;
#11099=DIRECTION ( 'NONE',  ( -0.6736849260863841948, 0.000000000000000000, 0.7390186874254148774 ) ) ;
#11157=AXIS2_PLACEMENT_3D ( 'NONE', #15535, #41323, #23402 ) ;
#11189=EDGE_LOOP ( 'NONE', ( #65754, #53779 ) ) ;
#11241=DIRECTION ( 'NONE',  ( -5.980589973904019347E-17, 1.000000000000000000, -1.736889445713099699E-16 ) ) ;
#11250=CARTESIAN_POINT ( 'NONE',  ( 19.63722818192610120, 1517.151704408390060, 218.2362632616380154 ) ) ;
#11259=VERTEX_POINT ( 'NONE', #21744 ) ;
#11278=FACE_OUTER_BOUND ( 'NONE', #35621, .T. ) ;
#11279=CYLINDRICAL_SURFACE ( 'NONE', #38985, 2.000000000000003553 ) ;
#11362=EDGE_LOOP ( 'NONE', ( #70091, #110735, #80095, #36403 ) ) ;
#11364=EDGE_LOOP ( 'NONE', ( #85491, #101188, #28723, #9456, #64918 ) ) ;
#11379=EDGE_LOOP ( 'NONE', ( #13415, #5294, #10806, #73899, #41511 ) ) ;
#11391=ADVANCED_FACE ( 'NONE', ( #21188 ), #51388, .F. ) ;
#11419=CYLINDRICAL_SURFACE ( 'NONE', #40830, 2.000000000000003553 ) ;
#11513=ORIENTED_EDGE ( 'NONE', *, *, #92691, .T. ) ;
#11594=EDGE_LOOP ( 'NONE', ( #49100, #71110, #74495, #9348 ) ) ;
#11607=CYLINDRICAL_SURFACE ( 'NONE', #108989, 1.999999999999999556 ) ;
#11617=FACE_OUTER_BOUND ( 'NONE', #99222, .T. ) ;
#11642=AXIS2_PLACEMENT_3D ( 'NONE', #26209, #10532, #11099 ) ;
#11643=ORIENTED_EDGE ( 'NONE', *, *, #56349, .T. ) ;
#11686=AXIS2_PLACEMENT_3D ( 'NONE', #91042, #23827, #15973 ) ;
#11691=FACE_OUTER_BOUND ( 'NONE', #3679, .T. ) ;
#11701=CYLINDRICAL_SURFACE ( 'NONE', #46238, 1.999999999999999556 ) ;
#11766=FACE_OUTER_BOUND ( 'NONE', #4069, .T. ) ;
#11770=DIRECTION ( 'NONE',  ( -1.755985294532469921E-16, 1.000000000000000000, -1.338183447452831989E-16 ) ) ;
#11773=EDGE_LOOP ( 'NONE', ( #35034, #34518, #93968, #49616, #91655 ) ) ;
#11774=ORIENTED_EDGE ( 'NONE', *, *, #64378, .F. ) ;
#11790=ORIENTED_EDGE ( 'NONE', *, *, #18010, .F. ) ;
#11802=VECTOR ( 'NONE', #76260, 1000.000000000000000 ) ;
#11825=ORIENTED_EDGE ( 'NONE', *, *, #46098, .F. ) ;
#11835=CARTESIAN_POINT ( 'NONE',  ( 21.62164173326539895, 1522.051704408389924, 208.0273405521070060 ) ) ;
#11881=DIRECTION ( 'NONE',  ( -1.755985294532469921E-16, 1.000000000000000000, -1.338183447452831989E-16 ) ) ;
#11905=EDGE_LOOP ( 'NONE', ( #87802, #63935, #72206, #10259 ) ) ;
#11961=EDGE_LOOP ( 'NONE', ( #90511, #3128 ) ) ;
#12007=EDGE_CURVE ( 'NONE', #105161, #35207, #25372, .T. ) ;
#12029=DIRECTION ( 'NONE',  ( 0.9455185755993178454, 0.000000000000000000, -0.3255681544571537578 ) ) ;
#12032=LINE ( 'NONE', #70324, #69572 ) ;
#12036=DIRECTION ( 'NONE',  ( -1.755985294532469921E-16, 1.000000000000000000, -1.338183447452831989E-16 ) ) ;
#12047=ORIENTED_EDGE ( 'NONE', *, *, #34185, .T. ) ;
#12051=AXIS2_PLACEMENT_3D ( 'NONE', #6592, #93340, #84933 ) ;
#12071=AXIS2_PLACEMENT_3D ( 'NONE', #58698, #92281, #32918 ) ;
#12117=AXIS2_PLACEMENT_3D ( 'NONE', #109765, #33045, #24619 ) ;
#12119=CARTESIAN_POINT ( 'NONE',  ( 14.38014760757802968, 1517.151704408390060, 208.3596762285818045 ) ) ;
#12133=CARTESIAN_POINT ( 'NONE',  ( 13.77266209894789917, 1517.151704408390060, 201.2043266506040027 ) ) ;
#12150=DIRECTION ( 'NONE',  ( 1.755985294532464991E-16, -1.000000000000000000, 1.338183447452830017E-16 ) ) ;
#12161=CARTESIAN_POINT ( 'NONE',  ( 21.62164173114529930, 1517.051704408389924, 208.0273405545509888 ) ) ;
#12195=VECTOR ( 'NONE', #87784, 1000.000000000000000 ) ;
#12204=CYLINDRICAL_SURFACE ( 'NONE', #81280, 2.000000000000003553 ) ;
#12206=ORIENTED_EDGE ( 'NONE', *, *, #98933, .T. ) ;
#12209=DIRECTION ( 'NONE',  ( 1.755985294532464991E-16, -1.000000000000000000, 1.338183447452830017E-16 ) ) ;
#12221=ORIENTED_EDGE ( 'NONE', *, *, #110594, .T. ) ;
#12230=CIRCLE ( 'NONE', #94466, 1.999999999999999556 ) ;
#12243=DIRECTION ( 'NONE',  ( 5.980589973904019347E-17, -1.000000000000000000, 1.736889445713099699E-16 ) ) ;
#12275=ORIENTED_EDGE ( 'NONE', *, *, #94125, .T. ) ;
#12307=EDGE_CURVE ( 'NONE', #33249, #65829, #98685, .T. ) ;
#12327=ORIENTED_EDGE ( 'NONE', *, *, #2746, .T. ) ;
#12414=CARTESIAN_POINT ( 'NONE',  ( 7.878537825433329367, 1517.151704408390060, 200.0586249522280013 ) ) ;
#12425=CYLINDRICAL_SURFACE ( 'NONE', #3536, 2.000000000000002220 ) ;
#12480=EDGE_CURVE ( 'NONE', #86431, #59011, #28998, .T. ) ;
#12493=DIRECTION ( 'NONE',  ( 1.755985294532469921E-16, -1.000000000000000000, 1.338183447452831989E-16 ) ) ;
#12521=CARTESIAN_POINT ( 'NONE',  ( -3.968827103576990201, 1522.051704408389924, 229.5396913781519856 ) ) ;
#12589=ADVANCED_FACE ( 'NONE', ( #51157 ), #39989, .F. ) ;
#12655=ORIENTED_EDGE ( 'NONE', *, *, #46120, .F. ) ;
#12665=DIRECTION ( 'NONE',  ( -0.9455185755993177343, 0.000000000000000000, 0.3255681544571540909 ) ) ;
#12673=DIRECTION ( 'NONE',  ( 1.755985294532464991E-16, -1.000000000000000000, 1.338183447452830017E-16 ) ) ;
#12722=CARTESIAN_POINT ( 'NONE',  ( -10.26338073471560008, 1517.551704408389924, 184.6900425920350131 ) ) ;
#12747=DIRECTION ( 'NONE',  ( -0.9455185755993178454, 0.000000000000000000, 0.3255681544571537578 ) ) ;
#12765=EDGE_CURVE ( 'NONE', #41410, #60554, #57630, .T. ) ;
#12810=VECTOR ( 'NONE', #34252, 1000.000000000000000 ) ;
#12830=EDGE_LOOP ( 'NONE', ( #90851, #83797 ) ) ;
#12831=ORIENTED_EDGE ( 'NONE', *, *, #48155, .F. ) ;
#12873=AXIS2_PLACEMENT_3D ( 'NONE', #3924, #10655, #88995 ) ;
#12877=DIRECTION ( 'NONE',  ( 0.9455185755993178454, 0.000000000000000000, -0.3255681544571539243 ) ) ;
#12958=LINE ( 'NONE', #45509, #69049 ) ;
#12986=DIRECTION ( 'NONE',  ( 1.755985294532469921E-16, -1.000000000000000000, 1.338183447452831989E-16 ) ) ;
#12994=DIRECTION ( 'NONE',  ( -5.980589973904019347E-17, 1.000000000000000000, -1.736889445713099699E-16 ) ) ;
#13010=ORIENTED_EDGE ( 'NONE', *, *, #90350, .T. ) ;
#13067=DIRECTION ( 'NONE',  ( 5.980589973904019347E-17, -1.000000000000000000, 1.736889445713099699E-16 ) ) ;
#13069=CARTESIAN_POINT ( 'NONE',  ( -11.78824854703250047, 1517.151704408390060, 206.8304425649369875 ) ) ;
#13079=EDGE_CURVE ( 'NONE', #87972, #65907, #2167, .T. ) ;
#13083=ORIENTED_EDGE ( 'NONE', *, *, #30416, .T. ) ;
#13086=EDGE_CURVE ( 'NONE', #8406, #90277, #30253, .T. ) ;
#13157=DIRECTION ( 'NONE',  ( -0.9455185755993178454, 0.000000000000000000, 0.3255681544571537578 ) ) ;
#13158=ORIENTED_EDGE ( 'NONE', *, *, #46603, .F. ) ;
#13172=ORIENTED_EDGE ( 'NONE', *, *, #15183, .T. ) ;
#13177=AXIS2_PLACEMENT_3D ( 'NONE', #10247, #18627, #55035 ) ;
#13186=ADVANCED_FACE ( 'NONE', ( #90393 ), #4745, .F. ) ;
#13193=ORIENTED_EDGE ( 'NONE', *, *, #32333, .T. ) ;
#13213=ORIENTED_EDGE ( 'NONE', *, *, #89073, .T. ) ;
#13217=ORIENTED_EDGE ( 'NONE', *, *, #58216, .F. ) ;
#13231=EDGE_CURVE ( 'NONE', #100346, #21912, #23053, .T. ) ;
#13253=AXIS2_PLACEMENT_3D ( 'NONE', #98689, #47199, #83529 ) ;
#13280=DIRECTION ( 'NONE',  ( -1.755985294532469921E-16, 1.000000000000000000, -1.338183447452831989E-16 ) ) ;
#13291=VERTEX_POINT ( 'NONE', #97517 ) ;
#13318=ORIENTED_EDGE ( 'NONE', *, *, #60388, .F. ) ;
#13328=VECTOR ( 'NONE', #38434, 1000.000000000000000 ) ;
#13343=ORIENTED_EDGE ( 'NONE', *, *, #10614, .T. ) ;
#13397=CARTESIAN_POINT ( 'NONE',  ( 3.968827103902559550, 1522.051704408389924, 188.7040005461919918 ) ) ;
#13415=ORIENTED_EDGE ( 'NONE', *, *, #40017, .F. ) ;
#13448=EDGE_CURVE ( 'NONE', #71672, #54897, #58889, .T. ) ;
#13451=AXIS2_PLACEMENT_3D ( 'NONE', #39023, #35043, #26069 ) ;
#13462=ADVANCED_FACE ( 'NONE', ( #74535 ), #108666, .F. ) ;
#13464=CARTESIAN_POINT ( 'NONE',  ( -0.6370436997427022519, 1522.051704408389924, 217.8527312947061603 ) ) ;
#13470=CARTESIAN_POINT ( 'NONE',  ( 13.16517659032116860, 1517.051704408389924, 194.0489770726361485 ) ) ;
#13471=EDGE_CURVE ( 'NONE', #6947, #90388, #91004, .T. ) ;
#13524=EDGE_LOOP ( 'NONE', ( #58197, #15211, #13172, #62338, #3812 ) ) ;
#13552=DIRECTION ( 'NONE',  ( 1.755985294532464991E-16, -1.000000000000000000, 1.338183447452830017E-16 ) ) ;
#13556=DIRECTION ( 'NONE',  ( -1.755985294532469921E-16, 1.000000000000000000, -1.338183447452831989E-16 ) ) ;
#13584=EDGE_LOOP ( 'NONE', ( #37137, #93284 ) ) ;
#13646=ORIENTED_EDGE ( 'NONE', *, *, #52303, .F. ) ;
#13656=CARTESIAN_POINT ( 'NONE',  ( 1.925297170580940076, 1519.551704408389924, 230.6853930747409720 ) ) ;
#13658=( NAMED_UNIT ( * ) PLANE_ANGLE_UNIT ( ) SI_UNIT ( $, .RADIAN. ) );
#13663=ORIENTED_EDGE ( 'NONE', *, *, #52242, .F. ) ;
#13666=EDGE_LOOP ( 'NONE', ( #85739, #89540 ) ) ;
#13707=EDGE_CURVE ( 'NONE', #8134, #102115, #80313, .T. ) ;
#13710=ORIENTED_EDGE ( 'NONE', *, *, #57594, .F. ) ;
#13813=ORIENTED_EDGE ( 'NONE', *, *, #20296, .T. ) ;
#13816=ADVANCED_FACE ( 'NONE', ( #28879 ), #71475, .F. ) ;
#13890=DIRECTION ( 'NONE',  ( -0.9455185755993178454, 0.000000000000000000, 0.3255681544571539243 ) ) ;
#13901=ORIENTED_EDGE ( 'NONE', *, *, #59607, .T. ) ;
#13941=ORIENTED_EDGE ( 'NONE', *, *, #53555, .F. ) ;
#13967=AXIS2_PLACEMENT_3D ( 'NONE', #31394, #65574, #82902 ) ;
#13971=AXIS2_PLACEMENT_3D ( 'NONE', #102400, #26242, #49822 ) ;
#14009=LINE ( 'NONE', #56039, #25337 ) ;
#14023=DIRECTION ( 'NONE',  ( 5.980589973904019347E-17, -1.000000000000000000, 1.736889445713099699E-16 ) ) ;
#14053=ORIENTED_EDGE ( 'NONE', *, *, #38006, .F. ) ;
#14070=DIRECTION ( 'NONE',  ( -0.6736849260863841948, 0.000000000000000000, 0.7390186874254148774 ) ) ;
#14100=ORIENTED_EDGE ( 'NONE', *, *, #45484, .F. ) ;
#14108=EDGE_CURVE ( 'NONE', #98226, #108494, #1667, .T. ) ;
#14115=DIRECTION ( 'NONE',  ( 1.755985294532464991E-16, -1.000000000000000000, 1.338183447452830017E-16 ) ) ;
#14125=CARTESIAN_POINT ( 'NONE',  ( -17.71193101166619854, 1521.951704408389787, 221.5709757775249784 ) ) ;
#14134=LINE ( 'NONE', #83008, #871 ) ;
#14140=DIRECTION ( 'NONE',  ( -1.755985294532469921E-16, 1.000000000000000000, -1.338183447452831989E-16 ) ) ;
#14142=CIRCLE ( 'NONE', #69667, 2.000000000000003553 ) ;
#14163=ORIENTED_EDGE ( 'NONE', *, *, #103365, .T. ) ;
#14186=CARTESIAN_POINT ( 'NONE',  ( -12.39573405564622988, 1517.151704408390060, 199.6750929870061668 ) ) ;
#14211=FACE_BOUND ( 'NONE', #11189, .T. ) ;
#14275=ORIENTED_EDGE ( 'NONE', *, *, #60980, .F. ) ;
#14293=VECTOR ( 'NONE', #18209, 1000.000000000000000 ) ;
#14359=CIRCLE ( 'NONE', #50123, 1.999999999999999556 ) ;
#14362=EDGE_LOOP ( 'NONE', ( #92273, #72808 ) ) ;
#14368=CIRCLE ( 'NONE', #85921, 1.999999999999999556 ) ;
#14381=ORIENTED_EDGE ( 'NONE', *, *, #32, .T. ) ;
#14401=AXIS2_PLACEMENT_3D ( 'NONE', #37861, #72047, #73117 ) ;
#14432=CARTESIAN_POINT ( 'NONE',  ( 2.694739704345540332, 1517.151704408390060, 206.1657712119973382 ) ) ;
#14475=ORIENTED_EDGE ( 'NONE', *, *, #90855, .F. ) ;
#14503=LINE ( 'NONE', #31864, #53423 ) ;
#14517=DIRECTION ( 'NONE',  ( 1.755985294532464991E-16, -1.000000000000000000, 1.338183447452830017E-16 ) ) ;
#14519=CARTESIAN_POINT ( 'NONE',  ( -10.26338073471560008, 1517.551704408389924, 184.6900425920350131 ) ) ;
#14535=VERTEX_POINT ( 'NONE', #28611 ) ;
#14554=FACE_OUTER_BOUND ( 'NONE', #92326, .T. ) ;
#14572=CARTESIAN_POINT ( 'NONE',  ( 3.968827104744170331, 1517.051704408389924, 188.7040005449509863 ) ) ;
#14625=LINE ( 'NONE', #98630, #38912 ) ;
#14650=AXIS2_PLACEMENT_3D ( 'NONE', #43659, #85087, #8378 ) ;
#14714=CARTESIAN_POINT ( 'NONE',  ( 7.211935934568220574, 1517.151704408390060, 224.6757451961901495 ) ) ;
#14779=DIRECTION ( 'NONE',  ( -0.9455185755993178454, 0.000000000000000000, 0.3255681544571537578 ) ) ;
#14789=DIRECTION ( 'NONE',  ( -5.980589973904019347E-17, 1.000000000000000000, -1.736889445713099699E-16 ) ) ;
#14828=ORIENTED_EDGE ( 'NONE', *, *, #10415, .T. ) ;
#14836=APPLICATION_CONTEXT ( 'automotive_design' ) ;
#14860=CYLINDRICAL_SURFACE ( 'NONE', #94345, 2.000000000000003109 ) ;
#14889=FACE_BOUND ( 'NONE', #40270, .T. ) ;
#14979=VERTEX_POINT ( 'NONE', #65405 ) ;
#15008=DIRECTION ( 'NONE',  ( 5.980589973904019347E-17, -1.000000000000000000, 1.736889445713099699E-16 ) ) ;
#15012=FACE_OUTER_BOUND ( 'NONE', #105412, .T. ) ;
#15030=DIRECTION ( 'NONE',  ( 5.980589973904019347E-17, -1.000000000000000000, 1.736889445713099699E-16 ) ) ;
#15078=ADVANCED_FACE ( 'NONE', ( #95421 ), #6024, .F. ) ;
#15136=CARTESIAN_POINT ( 'NONE',  ( 1.925297170580940076, 1517.151704408390060, 230.6853930747409720 ) ) ;
#15170=CIRCLE ( 'NONE', #2683, 1.999999999999998668 ) ;
#15183=EDGE_CURVE ( 'NONE', #34885, #64221, #105409, .T. ) ;
#15186=DIRECTION ( 'NONE',  ( 0.9455185755993178454, 0.000000000000000000, -0.3255681544571539243 ) ) ;
#15211=ORIENTED_EDGE ( 'NONE', *, *, #17540, .T. ) ;
#15241=ORIENTED_EDGE ( 'NONE', *, *, #19994, .T. ) ;
#15273=LINE ( 'NONE', #49466, #33008 ) ;
#15298=CARTESIAN_POINT ( 'NONE',  ( -3.968827103576990201, 1519.551704408389924, 229.5396913781519856 ) ) ;
#15329=ORIENTED_EDGE ( 'NONE', *, *, #72050, .T. ) ;
#15343=VECTOR ( 'NONE', #26649, 1000.000000000000000 ) ;
#15344=ORIENTED_EDGE ( 'NONE', *, *, #22611, .F. ) ;
#15362=EDGE_CURVE ( 'NONE', #77632, #69558, #59288, .T. ) ;
#15394=EDGE_CURVE ( 'NONE', #50989, #18256, #80691, .T. ) ;
#15426=FACE_OUTER_BOUND ( 'NONE', #36100, .T. ) ;
#15436=FACE_BOUND ( 'NONE', #32076, .T. ) ;
#15443=ORIENTED_EDGE ( 'NONE', *, *, #44217, .F. ) ;
#15456=AXIS2_PLACEMENT_3D ( 'NONE', #49929, #15728, #83508 ) ;
#15460=EDGE_LOOP ( 'NONE', ( #73341, #77496 ) ) ;
#15464=CARTESIAN_POINT ( 'NONE',  ( 17.66967187227356817, 1517.051704408389924, 223.1030594000600900 ) ) ;
#15468=DIRECTION ( 'NONE',  ( 1.755985294532469921E-16, -1.000000000000000000, 1.338183447452831989E-16 ) ) ;
#15535=CARTESIAN_POINT ( 'NONE',  ( -11.78824854703250047, 1517.051704408389924, 206.8304425649369875 ) ) ;
#15557=DIRECTION ( 'NONE',  ( -1.755985294532469921E-16, 1.000000000000000000, -1.338183447452831989E-16 ) ) ;
#15573=DIRECTION ( 'NONE',  ( -5.980589973904019347E-17, 1.000000000000000000, -1.736889445713099699E-16 ) ) ;
#15578=CIRCLE ( 'NONE', #49602, 2.000000000000003553 ) ;
#15591=EDGE_LOOP ( 'NONE', ( #42562, #44273 ) ) ;
#15600=EDGE_LOOP ( 'NONE', ( #95176, #26120, #41531, #3794, #5621 ) ) ;
#15619=EDGE_CURVE ( 'NONE', #43462, #36571, #107534, .T. ) ;
#15631=ORIENTED_EDGE ( 'NONE', *, *, #71960, .F. ) ;
#15651=CIRCLE ( 'NONE', #105060, 1.999999999999998668 ) ;
#15683=ORIENTED_EDGE ( 'NONE', *, *, #49785, .F. ) ;
#15687=EDGE_LOOP ( 'NONE', ( #11090, #28742 ) ) ;
#15722=DIRECTION ( 'NONE',  ( 1.755985294532464991E-16, -1.000000000000000000, 1.338183447452830017E-16 ) ) ;
#15728=DIRECTION ( 'NONE',  ( -1.755985294532469921E-16, 1.000000000000000000, -1.338183447452831989E-16 ) ) ;
#15729=EDGE_LOOP ( 'NONE', ( #13813, #62398, #45571, #85347, #11825 ) ) ;
#15796=CARTESIAN_POINT ( 'NONE',  ( 7.878537825433329367, 1522.051704408389924, 200.0586249522280013 ) ) ;
#15822=CARTESIAN_POINT ( 'NONE',  ( -1.317811661047102678, 1522.051704408389924, 194.7136484256038500 ) ) ;
#15852=ORIENTED_EDGE ( 'NONE', *, *, #78829, .F. ) ;
#15866=ADVANCED_FACE ( 'NONE', ( #108377 ), #15942, .F. ) ;
#15870=EDGE_LOOP ( 'NONE', ( #87541, #13318, #68405, #100643 ) ) ;
#15899=CARTESIAN_POINT ( 'NONE',  ( 21.60894078575200439, 1519.551704408389924, 218.5714488936601470 ) ) ;
#15902=AXIS2_PLACEMENT_3D ( 'NONE', #79538, #87385, #54891 ) ;
#15916=ORIENTED_EDGE ( 'NONE', *, *, #9200, .T. ) ;
#15924=EDGE_CURVE ( 'NONE', #69928, #61329, #82529, .T. ) ;
#15942=CYLINDRICAL_SURFACE ( 'NONE', #109317, 2.000000000000003553 ) ;
#15950=DIRECTION ( 'NONE',  ( -0.9455185755993178454, 0.000000000000000000, 0.3255681544571537578 ) ) ;
#15955=LINE ( 'NONE', #22144, #109014 ) ;
#15966=ORIENTED_EDGE ( 'NONE', *, *, #60370, .T. ) ;
#15970=ORIENTED_EDGE ( 'NONE', *, *, #31807, .F. ) ;
#15973=DIRECTION ( 'NONE',  ( -0.6736849260863841948, 0.000000000000000000, 0.7390186874254148774 ) ) ;
#15983=FACE_BOUND ( 'NONE', #108999, .T. ) ;
#15986=ADVANCED_FACE ( 'NONE', ( #73409 ), #28792, .F. ) ;
#15988=LINE ( 'NONE', #41761, #42570 ) ;
#15999=CARTESIAN_POINT ( 'NONE',  ( -11.83466398015730725, 1517.051704408389924, 228.0588040460849015 ) ) ;
#16011=DIRECTION ( 'NONE',  ( 0.9455185755993178454, 0.000000000000000000, -0.3255681544571537578 ) ) ;
#16033=CARTESIAN_POINT ( 'NONE',  ( -6.954065720117950100, 1521.551704408389924, 183.5505540514350002 ) ) ;
#16056=AXIS2_PLACEMENT_3D ( 'NONE', #85343, #8639, #6997 ) ;
#16137=AXIS2_PLACEMENT_3D ( 'NONE', #65159, #98187, #107142 ) ;
#16160=ORIENTED_EDGE ( 'NONE', *, *, #70554, .T. ) ;
#16194=FACE_OUTER_BOUND ( 'NONE', #86581, .T. ) ;
#16210=CIRCLE ( 'NONE', #43033, 1.999999999999999556 ) ;
#16254=CARTESIAN_POINT ( 'NONE',  ( 2.621457251729791160, 1522.051704408389924, 190.1820379210428200 ) ) ;
#16301=ORIENTED_EDGE ( 'NONE', *, *, #80260, .T. ) ;
#16313=CIRCLE ( 'NONE', #78947, 2.000000000000003553 ) ;
#16341=DIRECTION ( 'NONE',  ( -0.6736849260863841948, 0.000000000000000000, 0.7390186874254148774 ) ) ;
#16381=DIRECTION ( 'NONE',  ( 5.980589973904019347E-17, -1.000000000000000000, 1.736889445713099699E-16 ) ) ;
#16406=ORIENTED_EDGE ( 'NONE', *, *, #51819, .F. ) ;
#16452=CARTESIAN_POINT ( 'NONE',  ( 15.69795926888880189, 1517.051704408389924, 222.7678737654429995 ) ) ;
#16469=DIRECTION ( 'NONE',  ( -1.755985294532469921E-16, 1.000000000000000000, -1.338183447452831989E-16 ) ) ;
#16475=ORIENTED_EDGE ( 'NONE', *, *, #57143, .F. ) ;
#16504=EDGE_CURVE ( 'NONE', #86231, #92059, #16313, .T. ) ;
#16509=ORIENTED_EDGE ( 'NONE', *, *, #64587, .T. ) ;
#16510=CYLINDRICAL_SURFACE ( 'NONE', #85581, 2.000000000000003109 ) ;
#16512=ORIENTED_EDGE ( 'NONE', *, *, #13086, .F. ) ;
#16524=FACE_BOUND ( 'NONE', #18189, .T. ) ;
#16564=VERTEX_POINT ( 'NONE', #22832 ) ;
#16581=ORIENTED_EDGE ( 'NONE', *, *, #32467, .F. ) ;
#16589=DIRECTION ( 'NONE',  ( -5.980589973904019347E-17, 1.000000000000000000, -1.736889445713099699E-16 ) ) ;
#16604=UNCERTAINTY_MEASURE_WITH_UNIT (LENGTH_MEASURE( 1.000000000000000082E-05 ), #86941, 'distance_accuracy_value', 'NONE');
#16618=CARTESIAN_POINT ( 'NONE',  ( 11.81780673814840021, 1517.051704408389924, 195.5270144474869767 ) ) ;
#16644=DIRECTION ( 'NONE',  ( 0.9455185755993182894, 0.000000000000000000, -0.3255681544571521480 ) ) ;
#16658=EDGE_LOOP ( 'NONE', ( #19202, #82286, #24933, #70345, #95139 ) ) ;
#16680=DIRECTION ( 'NONE',  ( 5.980589973904019347E-17, -1.000000000000000000, 1.736889445713099699E-16 ) ) ;
#16692=CYLINDRICAL_SURFACE ( 'NONE', #53448, 2.000000000000003553 ) ;
#16700=LINE ( 'NONE', #95655, #54588 ) ;
#16713=CARTESIAN_POINT ( 'NONE',  ( 11.18076303840565977, 1517.151704408390060, 204.2578997804941707 ) ) ;
#16715=CARTESIAN_POINT ( 'NONE',  ( -22.96901158596647008, 1517.151704408390060, 211.6943887467578236 ) ) ;
#16727=ADVANCED_FACE ( 'NONE', ( #18504 ), #52701, .F. ) ;
#16734=ADVANCED_FACE ( 'NONE', ( #648 ), #87399, .F. ) ;
#16736=LINE ( 'NONE', #50943, #45609 ) ;
#16747=VECTOR ( 'NONE', #34632, 1000.000000000000000 ) ;
#16806=FACE_OUTER_BOUND ( 'NONE', #19261, .T. ) ;
#16812=DIRECTION ( 'NONE',  ( 1.755985294532464991E-16, -1.000000000000000000, 1.338183447452830017E-16 ) ) ;
#16832=CIRCLE ( 'NONE', #22198, 1.999999999999998668 ) ;
#16908=AXIS2_PLACEMENT_3D ( 'NONE', #70522, #1650, #96802 ) ;
#16922=LINE ( 'NONE', #103149, #50156 ) ;
#16964=CIRCLE ( 'NONE', #79604, 1.999999999999999556 ) ;
#17004=EDGE_LOOP ( 'NONE', ( #93134, #47052 ) ) ;
#17021=CIRCLE ( 'NONE', #86759, 1.999999999999998668 ) ;
#17072=ORIENTED_EDGE ( 'NONE', *, *, #50710, .F. ) ;
#17076=CIRCLE ( 'NONE', #56452, 2.000000000000003553 ) ;
#17100=CARTESIAN_POINT ( 'NONE',  ( 9.833393186232900263, 1522.051704408389924, 205.7359371553449989 ) ) ;
#17102=CARTESIAN_POINT ( 'NONE',  ( 0.02955819112566610354, 1517.151704408390060, 193.2356110507530218 ) ) ;
#17108=EDGE_CURVE ( 'NONE', #71672, #73345, #110113, .T. ) ;
#17155=CYLINDRICAL_SURFACE ( 'NONE', #12051, 2.000000000000003553 ) ;
#17169=FACE_OUTER_BOUND ( 'NONE', #83489, .T. ) ;
#17176=AXIS2_PLACEMENT_3D ( 'NONE', #66569, #50310, #23955 ) ;
#17178=CARTESIAN_POINT ( 'NONE',  ( -10.26338073471560008, 1517.051704408389924, 184.6900425920350131 ) ) ;
#17197=EDGE_CURVE ( 'NONE', #35907, #47709, #18929, .T. ) ;
#17224=FACE_OUTER_BOUND ( 'NONE', #80289, .T. ) ;
#17238=EDGE_CURVE ( 'NONE', #102140, #20317, #77943, .T. ) ;
#17241=FACE_OUTER_BOUND ( 'NONE', #45946, .T. ) ;
#17243=EDGE_CURVE ( 'NONE', #22220, #85592, #35606, .T. ) ;
#17268=ORIENTED_EDGE ( 'NONE', *, *, #85543, .T. ) ;
#17303=DIRECTION ( 'NONE',  ( -5.980589973904019347E-17, 1.000000000000000000, -1.736889445713099699E-16 ) ) ;
#17322=DIRECTION ( 'NONE',  ( 1.755985294532469921E-16, -1.000000000000000000, 1.338183447452831989E-16 ) ) ;
#17334=AXIS2_PLACEMENT_3D ( 'NONE', #9044, #85194, #66781 ) ;
#17335=CARTESIAN_POINT ( 'NONE',  ( -13.72624666664203552, 1519.551704408389924, 195.8110037932692933 ) ) ;
#17379=PRODUCT_CONTEXT ( 'NONE', #108540, 'mechanical' ) ;
#17395=DIRECTION ( 'NONE',  ( -0.6736849260863839728, 0.000000000000000000, 0.7390186874254150995 ) ) ;
#17415=DIRECTION ( 'NONE',  ( -1.755985294532469921E-16, 1.000000000000000000, -1.338183447452831989E-16 ) ) ;
#17500=FACE_BOUND ( 'NONE', #20867, .T. ) ;
#17540=EDGE_CURVE ( 'NONE', #20317, #34885, #69019, .T. ) ;
#17553=AXIS2_PLACEMENT_3D ( 'NONE', #64310, #46958, #56445 ) ;
#17579=MECHANICAL_DESIGN_GEOMETRIC_PRESENTATION_REPRESENTATION('',(#24767),#105219);
#17597=ORIENTED_EDGE ( 'NONE', *, *, #5075, .F. ) ;
#17662=ORIENTED_EDGE ( 'NONE', *, *, #63095, .F. ) ;
#17709=CONICAL_SURFACE ( 'NONE', #94631, 1.000000000000007327, 0.7853981633970000820 ) ;
#17713=CYLINDRICAL_SURFACE ( 'NONE', #69293, 2.000000000000003109 ) ;
#17741=AXIS2_PLACEMENT_3D ( 'NONE', #81668, #40235, #107985 ) ;
#17745=EDGE_LOOP ( 'NONE', ( #43209, #48383 ) ) ;
#17773=EDGE_CURVE ( 'NONE', #64279, #54634, #88930, .T. ) ;
#17789=AXIS2_PLACEMENT_3D ( 'NONE', #16618, #68199, #50284 ) ;
#17791=ORIENTED_EDGE ( 'NONE', *, *, #85108, .T. ) ;
#17849=DIRECTION ( 'NONE',  ( -0.6736849260863839728, 0.000000000000000000, 0.7390186874254150995 ) ) ;
#17867=CIRCLE ( 'NONE', #1868, 1.999999999999999556 ) ;
#17903=DIRECTION ( 'NONE',  ( -5.980589973904019347E-17, 1.000000000000000000, -1.736889445713099699E-16 ) ) ;
#17918=DIRECTION ( 'NONE',  ( -1.755985294532469921E-16, 1.000000000000000000, -1.338183447452831989E-16 ) ) ;
#17936=DIRECTION ( 'NONE',  ( 1.755985294532464991E-16, -1.000000000000000000, 1.338183447452830017E-16 ) ) ;
#17947=VERTEX_POINT ( 'NONE', #70646 ) ;
#17960=CARTESIAN_POINT ( 'NONE',  ( -4.576312612474013441, 1517.051704408389924, 222.3843417993991807 ) ) ;
#17965=EDGE_LOOP ( 'NONE', ( #12831, #26970, #14100, #2000, #80889 ) ) ;
#17973=VECTOR ( 'NONE', #1859, 1000.000000000000000 ) ;
#17997=VERTEX_POINT ( 'NONE', #69539 ) ;
#17999=AXIS2_PLACEMENT_3D ( 'NONE', #45694, #4223, #80378 ) ;
#18000=DIRECTION ( 'NONE',  ( 1.755985294532469921E-16, -1.000000000000000000, 1.338183447452831989E-16 ) ) ;
#18010=EDGE_CURVE ( 'NONE', #92059, #60698, #56019, .T. ) ;
#18041=VECTOR ( 'NONE', #35325, 1000.000000000000000 ) ;
#18048=CIRCLE ( 'NONE', #46713, 1.999999999999999556 ) ;
#18061=CARTESIAN_POINT ( 'NONE',  ( -3.968827103576990201, 1517.151704408390060, 229.5396913781519856 ) ) ;
#18065=CIRCLE ( 'NONE', #93200, 2.000000000000002220 ) ;
#18069=FACE_BOUND ( 'NONE', #40847, .T. ) ;
#18115=EDGE_LOOP ( 'NONE', ( #59069, #108185 ) ) ;
#18123=CARTESIAN_POINT ( 'NONE',  ( -1.925297170580940076, 1519.551704408389924, 187.5582988486569889 ) ) ;
#18162=LINE ( 'NONE', #92667, #46736 ) ;
#18166=DIRECTION ( 'NONE',  ( 1.755985294532464991E-16, -1.000000000000000000, 1.338183447452830017E-16 ) ) ;
#18178=VECTOR ( 'NONE', #5231, 1000.000000000000000 ) ;
#18189=EDGE_LOOP ( 'NONE', ( #24377, #39892 ) ) ;
#18201=CARTESIAN_POINT ( 'NONE',  ( -11.21032122992201785, 1519.551704408389924, 229.8720270527158220 ) ) ;
#18209=DIRECTION ( 'NONE',  ( 5.980589973904019347E-17, -1.000000000000000000, 1.736889445713099699E-16 ) ) ;
#18217=ORIENTED_EDGE ( 'NONE', *, *, #106899, .F. ) ;
#18252=VERTEX_POINT ( 'NONE', #64860 ) ;
#18256=VERTEX_POINT ( 'NONE', #39632 ) ;
#18261=EDGE_CURVE ( 'NONE', #82777, #75258, #47782, .T. ) ;
#18297=CARTESIAN_POINT ( 'NONE',  ( 11.83466398084630811, 1519.551704408389924, 190.1848878784103363 ) ) ;
#18306=CYLINDRICAL_SURFACE ( 'NONE', #83316, 1.999999999999999556 ) ;
#18332=CARTESIAN_POINT ( 'NONE',  ( -15.72751745975079984, 1517.151704408390060, 211.3620530696679793 ) ) ;
#18346=ORIENTED_EDGE ( 'NONE', *, *, #57013, .F. ) ;
#18448=ORIENTED_EDGE ( 'NONE', *, *, #55531, .T. ) ;
#18485=CARTESIAN_POINT ( 'NONE',  ( -16.36456115631863284, 1519.551704408389924, 220.0929384032941698 ) ) ;
#18490=EDGE_CURVE ( 'NONE', #76035, #33799, #76390, .T. ) ;
#18504=FACE_OUTER_BOUND ( 'NONE', #38353, .T. ) ;
#18538=CIRCLE ( 'NONE', #81132, 1.999999999999998890 ) ;
#18552=VECTOR ( 'NONE', #4486, 1000.000000000000000 ) ;
#18580=DIRECTION ( 'NONE',  ( -1.755985294532469921E-16, 1.000000000000000000, -1.338183447452831989E-16 ) ) ;
#18588=CARTESIAN_POINT ( 'NONE',  ( -4.491820960670080849E-16, 1519.551704408389924, 209.1218459616989946 ) ) ;
#18627=DIRECTION ( 'NONE',  ( 1.755985294532464991E-16, -1.000000000000000000, 1.338183447452830017E-16 ) ) ;
#18655=VERTEX_POINT ( 'NONE', #4131 ) ;
#18657=ORIENTED_EDGE ( 'NONE', *, *, #26072, .T. ) ;
#18670=CARTESIAN_POINT ( 'NONE',  ( 13.72624666093210521, 1519.551704408389924, 222.4326881300486889 ) ) ;
#18688=CIRCLE ( 'NONE', #95599, 1.999999999999998668 ) ;
#18697=CIRCLE ( 'NONE', #81285, 1.999999999999998668 ) ;
#18702=DIRECTION ( 'NONE',  ( -0.6736849260149578855, 0.000000000000000000, 0.7390186874905266823 ) ) ;
#18754=DIRECTION ( 'NONE',  ( 1.755985294532464991E-16, -1.000000000000000000, 1.338183447452830017E-16 ) ) ;
#18814=AXIS2_PLACEMENT_3D ( 'NONE', #37126, #80787, #88100 ) ;
#18828=CARTESIAN_POINT ( 'NONE',  ( -13.16517659032116860, 1522.051704408389924, 224.1947148507618408 ) ) ;
#18831=CARTESIAN_POINT ( 'NONE',  ( -0.02955819112566700213, 1522.051704408389924, 225.0080808726450243 ) ) ;
#18838=LINE ( 'NONE', #36769, #46563 ) ;
#18860=LINE ( 'NONE', #79354, #58647 ) ;
#18873=LINE ( 'NONE', #45785, #60740 ) ;
#18881=AXIS2_PLACEMENT_3D ( 'NONE', #35569, #110077, #69764 ) ;
#18891=CARTESIAN_POINT ( 'NONE',  ( -15.12003195112066933, 1517.051704408389924, 218.5174026476448432 ) ) ;
#18911=DIRECTION ( 'NONE',  ( -1.755985294532469921E-16, 1.000000000000000000, -1.338183447452831989E-16 ) ) ;
#18922=CARTESIAN_POINT ( 'NONE',  ( 13.74310390781900004, 1517.051704408389924, 217.0905615615409943 ) ) ;
#18929=CIRCLE ( 'NONE', #99422, 1.999999999999998668 ) ;
#18931=CIRCLE ( 'NONE', #31416, 1.999999999999999556 ) ;
#18940=ORIENTED_EDGE ( 'NONE', *, *, #24005, .F. ) ;
#18941=DIRECTION ( 'NONE',  ( 5.980589973904019347E-17, -1.000000000000000000, 1.736889445713099699E-16 ) ) ;
#19028=VECTOR ( 'NONE', #19737, 1000.000000000000000 ) ;
#19081=CARTESIAN_POINT ( 'NONE',  ( -15.72751745975079984, 1517.151704408390060, 211.3620530696679793 ) ) ;
#19115=CYLINDRICAL_SURFACE ( 'NONE', #69409, 4.000000000000006217 ) ;
#19116=EDGE_CURVE ( 'NONE', #10824, #50393, #10201, .T. ) ;
#19155=AXIS2_PLACEMENT_3D ( 'NONE', #14572, #73401, #107539 ) ;
#19162=CONICAL_SURFACE ( 'NONE', #81755, 1.000000000000007327, 0.7853981633970000820 ) ;
#19168=ORIENTED_EDGE ( 'NONE', *, *, #10427, .T. ) ;
#19202=ORIENTED_EDGE ( 'NONE', *, *, #92766, .F. ) ;
#19205=ORIENTED_EDGE ( 'NONE', *, *, #20010, .F. ) ;
#19227=EDGE_LOOP ( 'NONE', ( #3222, #85696 ) ) ;
#19234=CIRCLE ( 'NONE', #28216, 1.999999999999998668 ) ;
#19244=CIRCLE ( 'NONE', #101571, 2.000000000000003109 ) ;
#19261=EDGE_LOOP ( 'NONE', ( #6601, #104143, #26137, #39871 ) ) ;
#19263=ADVANCED_FACE ( 'NONE', ( #83298 ), #17155, .F. ) ;
#19295=FACE_BOUND ( 'NONE', #83749, .T. ) ;
#19300=LINE ( 'NONE', #95480, #1416 ) ;
#19338=LINE ( 'NONE', #35603, #106237 ) ;
#19362=ADVANCED_FACE ( 'NONE', ( #34545 ), #17713, .F. ) ;
#19368=DIRECTION ( 'NONE',  ( -1.755985294532469921E-16, 1.000000000000000000, -1.338183447452831989E-16 ) ) ;
#19379=EDGE_CURVE ( 'NONE', #70030, #63160, #20980, .T. ) ;
#19392=CARTESIAN_POINT ( 'NONE',  ( -15.69795926999090163, 1522.051704408389924, 195.4758181584410011 ) ) ;
#19400=CIRCLE ( 'NONE', #92703, 26.50000000000001421 ) ;
#19449=DIRECTION ( 'NONE',  ( -1.755985294532469921E-16, 1.000000000000000000, -1.338183447452831989E-16 ) ) ;
#19461=VERTEX_POINT ( 'NONE', #82628 ) ;
#19550=ORIENTED_EDGE ( 'NONE', *, *, #21692, .F. ) ;
#19559=CARTESIAN_POINT ( 'NONE',  ( 6.501609782144663896, 1517.051704408389924, 217.4228972380528262 ) ) ;
#19619=ORIENTED_EDGE ( 'NONE', *, *, #82518, .F. ) ;
#19641=AXIS2_PLACEMENT_3D ( 'NONE', #63951, #38708, #56079 ) ;
#19704=CYLINDRICAL_SURFACE ( 'NONE', #76343, 1.999999999999999556 ) ;
#19736=CIRCLE ( 'NONE', #37647, 1.999999999999999556 ) ;
#19737=DIRECTION ( 'NONE',  ( 5.980589973904019347E-17, -1.000000000000000000, 1.736889445713099699E-16 ) ) ;
#19824=CARTESIAN_POINT ( 'NONE',  ( -14.35058941781813324, 1522.051704408389924, 193.9977807835901729 ) ) ;
#19826=AXIS2_PLACEMENT_3D ( 'NONE', #88816, #52473, #87160 ) ;
#19852=LINE ( 'NONE', #56226, #5701 ) ;
#19882=ORIENTED_EDGE ( 'NONE', *, *, #103731, .T. ) ;
#19927=AXIS2_PLACEMENT_3D ( 'NONE', #20613, #86742, #96811 ) ;
#19931=LINE ( 'NONE', #36196, #96677 ) ;
#19932=DIRECTION ( 'NONE',  ( 0.3255681544571569219, 1.836970198721028948E-16, 0.9455185755993167351 ) ) ;
#19937=EDGE_LOOP ( 'NONE', ( #43118, #53004, #55304, #105844 ) ) ;
#19969=ADVANCED_BREP_SHAPE_REPRESENTATION ( '', ( #82338, #21632 ), #61094 ) ;
#19977=ORIENTED_EDGE ( 'NONE', *, *, #50557, .T. ) ;
#19989=ADVANCED_FACE ( 'NONE', ( #106719 ), #88831, .F. ) ;
#19994=EDGE_CURVE ( 'NONE', #28393, #66581, #33514, .T. ) ;
#19997=DIRECTION ( 'NONE',  ( 1.755985294532464991E-16, -1.000000000000000000, 1.338183447452830017E-16 ) ) ;
#20006=CARTESIAN_POINT ( 'NONE',  ( -7.005862043813290743E-15, 1521.551704408389924, 209.1218459616989946 ) ) ;
#20010=EDGE_CURVE ( 'NONE', #8134, #14979, #55806, .T. ) ;
#20025=ORIENTED_EDGE ( 'NONE', *, *, #26068, .T. ) ;
#20028=AXIS2_PLACEMENT_3D ( 'NONE', #27731, #18754, #85979 ) ;
#20071=CYLINDRICAL_SURFACE ( 'NONE', #96404, 2.000000000000003109 ) ;
#20095=CIRCLE ( 'NONE', #50497, 1.999999999999999556 ) ;
#20154=ADVANCED_FACE ( 'NONE', ( #84816 ), #14860, .F. ) ;
#20162=ORIENTED_EDGE ( 'NONE', *, *, #29523, .F. ) ;
#20163=ORIENTED_EDGE ( 'NONE', *, *, #75383, .T. ) ;
#20183=ORIENTED_EDGE ( 'NONE', *, *, #82984, .T. ) ;
#20193=FACE_OUTER_BOUND ( 'NONE', #30907, .T. ) ;
#20242=DIRECTION ( 'NONE',  ( 1.755985294532464991E-16, -1.000000000000000000, 1.338183447452830017E-16 ) ) ;
#20258=EDGE_LOOP ( 'NONE', ( #54509, #88871 ) ) ;
#20260=CARTESIAN_POINT ( 'NONE',  ( 20.98459803409887314, 1517.151704408390060, 216.7582258867871587 ) ) ;
#20272=DIRECTION ( 'NONE',  ( -1.755985294532469921E-16, 1.000000000000000000, -1.338183447452831989E-16 ) ) ;
#20282=EDGE_LOOP ( 'NONE', ( #29544, #20025, #97092, #11790, #66251 ) ) ;
#20296=EDGE_CURVE ( 'NONE', #8434, #76507, #24560, .T. ) ;
#20302=CARTESIAN_POINT ( 'NONE',  ( 17.71193101166619854, 1519.551704408389924, 196.6727161458730109 ) ) ;
#20317=VERTEX_POINT ( 'NONE', #25735 ) ;
#20343=EDGE_CURVE ( 'NONE', #28739, #31342, #38887, .T. ) ;
#20346=ORIENTED_EDGE ( 'NONE', *, *, #63306, .T. ) ;
#20363=LINE ( 'NONE', #107136, #18178 ) ;
#20366=DIRECTION ( 'NONE',  ( 1.755985294532469921E-16, -1.000000000000000000, 1.338183447452831989E-16 ) ) ;
#20439=ADVANCED_FACE ( 'NONE', ( #100790 ), #76163, .F. ) ;
#20461=VERTEX_POINT ( 'NONE', #58815 ) ;
#20613=CARTESIAN_POINT ( 'NONE',  ( 19.63722818192610120, 1519.551704408389924, 218.2362632616380154 ) ) ;
#20642=CYLINDRICAL_SURFACE ( 'NONE', #28639, 2.000000000000011102 ) ;
#20671=EDGE_CURVE ( 'NONE', #21086, #32612, #3203, .T. ) ;
#20681=CARTESIAN_POINT ( 'NONE',  ( -15.72751745975079984, 1517.051704408389924, 211.3620530696679793 ) ) ;
#20683=EDGE_CURVE ( 'NONE', #58053, #18655, #18860, .T. ) ;
#20690=AXIS2_PLACEMENT_3D ( 'NONE', #73884, #89564, #30199 ) ;
#20697=VERTEX_POINT ( 'NONE', #88300 ) ;
#20701=ORIENTED_EDGE ( 'NONE', *, *, #6881, .F. ) ;
#20783=VERTEX_POINT ( 'NONE', #8132 ) ;
#20808=DIRECTION ( 'NONE',  ( -0.9455185755993178454, 0.000000000000000000, 0.3255681544571537578 ) ) ;
#20848=ORIENTED_EDGE ( 'NONE', *, *, #35860, .F. ) ;
#20867=EDGE_LOOP ( 'NONE', ( #15329, #45928 ) ) ;
#20869=EDGE_LOOP ( 'NONE', ( #44121, #63841, #78174, #7626 ) ) ;
#20879=DIRECTION ( 'NONE',  ( 0.9455185755993178454, 0.000000000000000000, -0.3255681544571537578 ) ) ;
#20886=CYLINDRICAL_SURFACE ( 'NONE', #108790, 2.000000000000002220 ) ;
#20893=ORIENTED_EDGE ( 'NONE', *, *, #22823, .T. ) ;
#20930=EDGE_CURVE ( 'NONE', #25738, #63587, #55151, .T. ) ;
#20932=DIRECTION ( 'NONE',  ( -0.9455185755993178454, 0.000000000000000000, 0.3255681544571539243 ) ) ;
#20957=ORIENTED_EDGE ( 'NONE', *, *, #90539, .T. ) ;
#20980=CIRCLE ( 'NONE', #44268, 1.999999999999998668 ) ;
#20997=CARTESIAN_POINT ( 'NONE',  ( 21.63849897582232273, 1519.551704408389924, 202.6852139837732523 ) ) ;
#21008=ORIENTED_EDGE ( 'NONE', *, *, #21892, .F. ) ;
#21062=CYLINDRICAL_SURFACE ( 'NONE', #80178, 2.000000000000003553 ) ;
#21086=VERTEX_POINT ( 'NONE', #93110 ) ;
#21119=ORIENTED_EDGE ( 'NONE', *, *, #44217, .T. ) ;
#21166=LINE ( 'NONE', #55374, #40754 ) ;
#21181=ADVANCED_FACE ( 'NONE', ( #84158 ), #99849, .F. ) ;
#21188=FACE_OUTER_BOUND ( 'NONE', #41398, .T. ) ;
#21199=VERTEX_POINT ( 'NONE', #32113 ) ;
#21249=EDGE_CURVE ( 'NONE', #93813, #60698, #101541, .T. ) ;
#21272=ADVANCED_FACE ( 'NONE', ( #63961 ), #96440, .F. ) ;
#21306=VECTOR ( 'NONE', #96786, 1000.000000000000000 ) ;
#21325=CARTESIAN_POINT ( 'NONE',  ( 1.823067188510389982E-15, 1517.051704408389924, 209.1218459616989946 ) ) ;
#21329=DIRECTION ( 'NONE',  ( 1.755985294532469921E-16, -1.000000000000000000, 1.338183447452831989E-16 ) ) ;
#21332=CARTESIAN_POINT ( 'NONE',  ( -17.04532912216367180, 1517.151704408390060, 196.9538555332918293 ) ) ;
#21400=CARTESIAN_POINT ( 'NONE',  ( -9.862951377749247683, 1522.051704408389924, 228.3939896778649654 ) ) ;
#21420=LINE ( 'NONE', #84647, #11802 ) ;
#21429=CARTESIAN_POINT ( 'NONE',  ( -3.290427993577100100E-15, 1522.051704408389924, 209.1218459616989946 ) ) ;
#21433=AXIS2_PLACEMENT_3D ( 'NONE', #71448, #14789, #4735 ) ;
#21471=DIRECTION ( 'NONE',  ( -0.6736849260863841948, 0.000000000000000000, 0.7390186874254148774 ) ) ;
#21478=ORIENTED_EDGE ( 'NONE', *, *, #22780, .F. ) ;
#21487=CIRCLE ( 'NONE', #55506, 1.999999999999998668 ) ;
#21516=VERTEX_POINT ( 'NONE', #103439 ) ;
#21529=DIRECTION ( 'NONE',  ( -1.755985294532469921E-16, 1.000000000000000000, -1.338183447452831989E-16 ) ) ;
#21534=AXIS2_PLACEMENT_3D ( 'NONE', #29701, #39195, #2884 ) ;
#21536=EDGE_CURVE ( 'NONE', #68701, #97416, #36812, .T. ) ;
#21540=ADVANCED_FACE ( 'NONE', ( #79373 ), #62612, .F. ) ;
#21567=CIRCLE ( 'NONE', #35911, 1.999999999999999556 ) ;
#21601=DIRECTION ( 'NONE',  ( 0.9455185755993182894, 0.000000000000000000, -0.3255681544571521480 ) ) ;
#21612=CARTESIAN_POINT ( 'NONE',  ( 13.77266209894789917, 1522.051704408389924, 201.2043266506040027 ) ) ;
#21632=AXIS2_PLACEMENT_3D ( 'NONE', #110085, #42890, #42328 ) ;
#21664=ADVANCED_FACE ( 'NONE', ( #58032 ), #92711, .F. ) ;
#21692=EDGE_CURVE ( 'NONE', #65489, #23415, #15988, .T. ) ;
#21698=DIRECTION ( 'NONE',  ( -0.6736849260149578855, 0.000000000000000000, 0.7390186874905266823 ) ) ;
#21719=VERTEX_POINT ( 'NONE', #25494 ) ;
#21722=VECTOR ( 'NONE', #7192, 1000.000000000000000 ) ;
#21744=CARTESIAN_POINT ( 'NONE',  ( 8.515581525185790923, 1522.051704408389924, 191.3277396192498543 ) ) ;
#21750=DIRECTION ( 'NONE',  ( -0.6736849260863839728, 0.000000000000000000, 0.7390186874254150995 ) ) ;
#21798=VECTOR ( 'NONE', #8440, 1000.000000000000000 ) ;
#21832=DIRECTION ( 'NONE',  ( 0.3255681544571567554, 0.000000000000000000, 0.9455185755993167351 ) ) ;
#21892=EDGE_CURVE ( 'NONE', #27217, #37900, #19300, .T. ) ;
#21912=VERTEX_POINT ( 'NONE', #18201 ) ;
#21946=CARTESIAN_POINT ( 'NONE',  ( -1.984413551915469975, 1522.051704408389924, 219.3307686695569885 ) ) ;
#21948=ORIENTED_EDGE ( 'NONE', *, *, #34316, .T. ) ;
#21966=CARTESIAN_POINT ( 'NONE',  ( -11.78824854703250047, 1517.151704408390060, 206.8304425649369875 ) ) ;
#22004=DIRECTION ( 'NONE',  ( -0.9455185755993177343, 0.000000000000000000, 0.3255681544571540909 ) ) ;
#22026=( BOUNDED_CURVE ( )  B_SPLINE_CURVE ( 2, ( #16033, #91108, #73214 ),
 .UNSPECIFIED., .F., .T. ) 
 B_SPLINE_CURVE_WITH_KNOTS ( ( 3, 3 ),
 ( -0.2337410562555060078, -0.1572692978119380192 ),
 .UNSPECIFIED. ) 
 CURVE ( )  GEOMETRIC_REPRESENTATION_ITEM ( )  RATIONAL_B_SPLINE_CURVE ( ( 1.002760198482619991, 1.002448066741719934, 1.002044729649790078 ) ) 
 REPRESENTATION_ITEM ( '' )  );
#22084=ORIENTED_EDGE ( 'NONE', *, *, #20343, .T. ) ;
#22094=DIRECTION ( 'NONE',  ( -1.755985294532469921E-16, 1.000000000000000000, -1.338183447452831989E-16 ) ) ;
#22110=AXIS2_PLACEMENT_3D ( 'NONE', #55593, #12994, #36026 ) ;
#22144=CARTESIAN_POINT ( 'NONE',  ( -5.257080573758879716, 1517.151704408390060, 199.2452589303538275 ) ) ;
#22169=DIRECTION ( 'NONE',  ( 2.042903098301770100E-14, 1.000000000000000000, -6.143886524153290706E-15 ) ) ;
#22174=DIRECTION ( 'NONE',  ( 0.9455185755993178454, 0.000000000000000000, -0.3255681544571537578 ) ) ;
#22197=ADVANCED_FACE ( 'NONE', ( #11617 ), #52523, .F. ) ;
#22198=AXIS2_PLACEMENT_3D ( 'NONE', #23467, #49797, #91773 ) ;
#22220=VERTEX_POINT ( 'NONE', #10507 ) ;
#22262=DIRECTION ( 'NONE',  ( 0.9858563016923833633, 0.000000000000000000, 0.1675928173085483863 ) ) ;
#22264=VERTEX_POINT ( 'NONE', #62615 ) ;
#22270=DIRECTION ( 'NONE',  ( 0.9455185755993178454, 0.000000000000000000, -0.3255681544571538688 ) ) ;
#22271=AXIS2_PLACEMENT_3D ( 'NONE', #64593, #4662, #105475 ) ;
#22290=PRODUCT ( 'Grinding Plate', 'Grinding Plate', '', ( #17379 ) ) ;
#22296=CYLINDRICAL_SURFACE ( 'NONE', #67866, 2.000000000000003553 ) ;
#22326=ADVANCED_FACE ( 'NONE', ( #72630 ), #4852, .F. ) ;
#22333=CARTESIAN_POINT ( 'NONE',  ( -0.02955819112566620069, 1517.051704408389924, 225.0080808726450243 ) ) ;
#22394=CIRCLE ( 'NONE', #110034, 2.000000000000002220 ) ;
#22437=AXIS2_PLACEMENT_3D ( 'NONE', #7203, #41903, #76604 ) ;
#22467=CIRCLE ( 'NONE', #25833, 3.999999999999997335 ) ;
#22494=EDGE_LOOP ( 'NONE', ( #86825, #24464 ) ) ;
#22506=CARTESIAN_POINT ( 'NONE',  ( -13.74310390781900004, 1522.051704408389924, 201.1531303618569950 ) ) ;
#22531=CARTESIAN_POINT ( 'NONE',  ( -23.59335433665016524, 1517.051704408389924, 209.8811657366738928 ) ) ;
#22546=CARTESIAN_POINT ( 'NONE',  ( 14.38014760757803145, 1517.051704408389924, 208.3596762285818045 ) ) ;
#22551=CARTESIAN_POINT ( 'NONE',  ( -19.66678637224480397, 1519.551704408389924, 215.8936635741279986 ) ) ;
#22553=CARTESIAN_POINT ( 'NONE',  ( -6.719124544191419801, 1517.051704408389924, 184.2328727701749926 ) ) ;
#22563=CARTESIAN_POINT ( 'NONE',  ( -18.28985832939523348, 1519.551704408389924, 198.5293912879491529 ) ) ;
#22577=DIRECTION ( 'NONE',  ( 0.9455185755993178454, 0.000000000000000000, -0.3255681544571539243 ) ) ;
#22606=ORIENTED_EDGE ( 'NONE', *, *, #15619, .F. ) ;
#22611=EDGE_CURVE ( 'NONE', #9033, #14535, #9309, .T. ) ;
#22619=VERTEX_POINT ( 'NONE', #26610 ) ;
#22650=EDGE_CURVE ( 'NONE', #36071, #66446, #99212, .T. ) ;
#22716=DIRECTION ( 'NONE',  ( 1.755985294532464991E-16, -1.000000000000000000, 1.338183447452830017E-16 ) ) ;
#22721=FACE_BOUND ( 'NONE', #13666, .T. ) ;
#22772=CARTESIAN_POINT ( 'NONE',  ( 19.02974267272306719, 1517.051704408389924, 211.0809136819971741 ) ) ;
#22774=CIRCLE ( 'NONE', #51425, 1.999999999999999556 ) ;
#22780=EDGE_CURVE ( 'NONE', #60349, #9033, #59927, .T. ) ;
#22792=DIRECTION ( 'NONE',  ( -1.755985294532469921E-16, 1.000000000000000000, -1.338183447452831989E-16 ) ) ;
#22795=CYLINDRICAL_SURFACE ( 'NONE', #40408, 2.000000000000011102 ) ;
#22823=EDGE_CURVE ( 'NONE', #78966, #21516, #25780, .T. ) ;
#22829=DIRECTION ( 'NONE',  ( -0.6736849260863839728, 0.000000000000000000, 0.7390186874254150995 ) ) ;
#22832=CARTESIAN_POINT ( 'NONE',  ( 16.33500296837753041, 1522.051704408389924, 214.0369884316988305 ) ) ;
#22878=DIRECTION ( 'NONE',  ( -5.980589973904019347E-17, 1.000000000000000000, -1.736889445713099699E-16 ) ) ;
#22900=AXIS2_PLACEMENT_3D ( 'NONE', #19392, #9905, #1524 ) ;
#22906=AXIS2_PLACEMENT_3D ( 'NONE', #71275, #56641, #20808 ) ;
#22915=EDGE_LOOP ( 'NONE', ( #104652, #3793, #42988, #45792, #33384 ) ) ;
#22921=ORIENTED_EDGE ( 'NONE', *, *, #13086, .T. ) ;
#22976=VERTEX_POINT ( 'NONE', #15464 ) ;
#22995=CARTESIAN_POINT ( 'NONE',  ( 15.12003195112066933, 1522.051704408389924, 199.7262892757531745 ) ) ;
#23004=CIRCLE ( 'NONE', #107110, 1.999999999999997780 ) ;
#23022=AXIS2_PLACEMENT_3D ( 'NONE', #83367, #66609, #32963 ) ;
#23024=ORIENTED_EDGE ( 'NONE', *, *, #66667, .F. ) ;
#23037=LINE ( 'NONE', #77872, #21798 ) ;
#23053=CIRCLE ( 'NONE', #107153, 2.000000000000002220 ) ;
#23080=CARTESIAN_POINT ( 'NONE',  ( 19.66678637246580053, 1522.051704408389924, 202.3500283489900085 ) ) ;
#23089=CIRCLE ( 'NONE', #87551, 1.999999999999999556 ) ;
#23117=EDGE_CURVE ( 'NONE', #11259, #105162, #43855, .T. ) ;
#23167=ORIENTED_EDGE ( 'NONE', *, *, #107746, .T. ) ;
#23170=EDGE_LOOP ( 'NONE', ( #4830, #35681, #56906, #101887, #71680 ) ) ;
#23179=FILL_AREA_STYLE_COLOUR ( '', #37813 ) ;
#23209=ORIENTED_EDGE ( 'NONE', *, *, #107894, .F. ) ;
#23233=AXIS2_PLACEMENT_3D ( 'NONE', #93428, #512, #78294 ) ;
#23258=VERTEX_POINT ( 'NONE', #41242 ) ;
#23260=CARTESIAN_POINT ( 'NONE',  ( -3.909710721586109550, 1517.151704408390060, 197.7672215555029993 ) ) ;
#23265=DIRECTION ( 'NONE',  ( -5.980589973904019347E-17, 1.000000000000000000, -1.736889445713099699E-16 ) ) ;
#23279=VERTEX_POINT ( 'NONE', #94378 ) ;
#23287=DIRECTION ( 'NONE',  ( -0.9455185755993178454, 0.000000000000000000, 0.3255681544571537578 ) ) ;
#23291=FACE_BOUND ( 'NONE', #68585, .T. ) ;
#23310=ADVANCED_FACE ( 'NONE', ( #31045 ), #89855, .F. ) ;
#23361=VECTOR ( 'NONE', #108641, 1000.000000000000000 ) ;
#23365=CARTESIAN_POINT ( 'NONE',  ( 11.81780673814840021, 1517.051704408389924, 195.5270144474869767 ) ) ;
#23402=DIRECTION ( 'NONE',  ( -0.9455185755993178454, 0.000000000000000000, 0.3255681544571537578 ) ) ;
#23415=VERTEX_POINT ( 'NONE', #30363 ) ;
#23433=ORIENTED_EDGE ( 'NONE', *, *, #23117, .F. ) ;
#23453=VECTOR ( 'NONE', #97324, 1000.000000000000000 ) ;
#23460=CARTESIAN_POINT ( 'NONE',  ( -7.848979634317430509, 1517.151704408390060, 202.2988320601959913 ) ) ;
#23467=CARTESIAN_POINT ( 'NONE',  ( -7.848979634317430509, 1522.051704408389924, 202.2988320601959913 ) ) ;
#23477=CARTESIAN_POINT ( 'NONE',  ( -10.18103031238790024, 1517.299312825791731, 184.9292055843397975 ) ) ;
#23509=CYLINDRICAL_SURFACE ( 'NONE', #39151, 26.50000000000001421 ) ;
#23528=CIRCLE ( 'NONE', #37863, 1.999999999999998668 ) ;
#23539=EDGE_LOOP ( 'NONE', ( #91491, #12206 ) ) ;
#23588=ORIENTED_EDGE ( 'NONE', *, *, #12007, .T. ) ;
#23592=ORIENTED_EDGE ( 'NONE', *, *, #44723, .T. ) ;
#23603=DIRECTION ( 'NONE',  ( 1.755985294532464991E-16, -1.000000000000000000, 1.338183447452830017E-16 ) ) ;
#23608=CARTESIAN_POINT ( 'NONE',  ( -3.909710721586120208, 1517.051704408389924, 197.7672215555029993 ) ) ;
#23631=ORIENTED_EDGE ( 'NONE', *, *, #30416, .F. ) ;
#23668=ORIENTED_EDGE ( 'NONE', *, *, #10303, .T. ) ;
#23690=DIRECTION ( 'NONE',  ( -1.755985294532469921E-16, 1.000000000000000000, -1.338183447452831989E-16 ) ) ;
#23707=LINE ( 'NONE', #27581, #17973 ) ;
#23721=EDGE_CURVE ( 'NONE', #46101, #49402, #25921, .T. ) ;
#23746=EDGE_CURVE ( 'NONE', #1490, #26765, #16700, .T. ) ;
#23805=ORIENTED_EDGE ( 'NONE', *, *, #9200, .F. ) ;
#23827=DIRECTION ( 'NONE',  ( -1.755985294532469921E-16, 1.000000000000000000, -1.338183447452831989E-16 ) ) ;
#23832=DIRECTION ( 'NONE',  ( 5.980589973904019347E-17, -1.000000000000000000, 1.736889445713099699E-16 ) ) ;
#23836=FACE_BOUND ( 'NONE', #87008, .T. ) ;
#23843=EDGE_CURVE ( 'NONE', #32285, #81525, #6275, .T. ) ;
#23853=CARTESIAN_POINT ( 'NONE',  ( 19.66678637211940028, 1517.051704408389924, 202.3500283489059939 ) ) ;
#23858=FACE_OUTER_BOUND ( 'NONE', #8322, .T. ) ;
#23929=DIRECTION ( 'NONE',  ( 0.9455185755993178454, 0.000000000000000000, -0.3255681544571539243 ) ) ;
#23955=DIRECTION ( 'NONE',  ( -0.6736849260863841948, 0.000000000000000000, 0.7390186874254148774 ) ) ;
#23982=DIRECTION ( 'NONE',  ( 0.9858563016923833633, 0.000000000000000000, 0.1675928173085483863 ) ) ;
#23984=DIRECTION ( 'NONE',  ( -0.6736849260863839728, 0.000000000000000000, 0.7390186874254150995 ) ) ;
#23995=DIRECTION ( 'NONE',  ( 0.9455185755993178454, 0.000000000000000000, -0.3255681544571537578 ) ) ;
#24005=EDGE_CURVE ( 'NONE', #110100, #110607, #8741, .T. ) ;
#24030=CIRCLE ( 'NONE', #59888, 2.000000000000003109 ) ;
#24042=CARTESIAN_POINT ( 'NONE',  ( -1.925297170580940076, 1517.151704408390060, 187.5582988486569889 ) ) ;
#24043=CARTESIAN_POINT ( 'NONE',  ( 13.13561839920527063, 1517.151704408390060, 209.9352119836111683 ) ) ;
#24061=ADVANCED_FACE ( 'NONE', ( #64576 ), #65114, .F. ) ;
#24063=CARTESIAN_POINT ( 'NONE',  ( -1.376928043298434101, 1517.051704408389924, 226.4861182474958525 ) ) ;
#24066=EDGE_CURVE ( 'NONE', #90388, #58309, #5918, .T. ) ;
#24131=EDGE_CURVE ( 'NONE', #84814, #17947, #45710, .T. ) ;
#24142=DIRECTION ( 'NONE',  ( -0.9455185755993178454, 0.000000000000000000, 0.3255681544571539243 ) ) ;
#24144=VERTEX_POINT ( 'NONE', #84090 ) ;
#24172=EDGE_CURVE ( 'NONE', #87558, #3107, #31362, .T. ) ;
#24183=ORIENTED_EDGE ( 'NONE', *, *, #44668, .F. ) ;
#24196=EDGE_CURVE ( 'NONE', #39431, #66581, #100876, .T. ) ;
#24233=DIRECTION ( 'NONE',  ( -0.6736849260863841948, 0.000000000000000000, 0.7390186874254148774 ) ) ;
#24259=CARTESIAN_POINT ( 'NONE',  ( -11.83466398157531962, 1519.551704408389924, 228.0588040458438286 ) ) ;
#24290=EDGE_LOOP ( 'NONE', ( #60287, #108769 ) ) ;
#24312=ORIENTED_EDGE ( 'NONE', *, *, #107681, .T. ) ;
#24320=CIRCLE ( 'NONE', #24397, 1.999999999999998668 ) ;
#24343=CARTESIAN_POINT ( 'NONE',  ( -9.196349486490200675, 1522.051704408389924, 203.7768694350468195 ) ) ;
#24377=ORIENTED_EDGE ( 'NONE', *, *, #69694, .T. ) ;
#24393=FACE_BOUND ( 'NONE', #87405, .T. ) ;
#24397=AXIS2_PLACEMENT_3D ( 'NONE', #44921, #67494, #44356 ) ;
#24425=DIRECTION ( 'NONE',  ( -0.6736849260863839728, 0.000000000000000000, 0.7390186874254150995 ) ) ;
#24435=CARTESIAN_POINT ( 'NONE',  ( 13.77266209894789917, 1522.051704408389924, 201.2043266506040027 ) ) ;
#24464=ORIENTED_EDGE ( 'NONE', *, *, #57993, .T. ) ;
#24510=AXIS2_PLACEMENT_3D ( 'NONE', #59626, #103244, #49575 ) ;
#24515=CARTESIAN_POINT ( 'NONE',  ( 13.74310390781900004, 1517.151704408390060, 217.0905615615409943 ) ) ;
#24548=CARTESIAN_POINT ( 'NONE',  ( 17.04532911661896932, 1519.551704408389924, 221.2898363890541589 ) ) ;
#24555=ORIENTED_EDGE ( 'NONE', *, *, #41136, .F. ) ;
#24560=CIRCLE ( 'NONE', #87177, 2.000000000000003109 ) ;
#24576=CARTESIAN_POINT ( 'NONE',  ( -15.74021840828143404, 1517.051704408389924, 221.9061614121420973 ) ) ;
#24619=DIRECTION ( 'NONE',  ( -0.6736849260863841948, 0.000000000000000000, 0.7390186874254148774 ) ) ;
#24622=EDGE_LOOP ( 'NONE', ( #84202, #6530, #61817, #95762, #89023 ) ) ;
#24665=AXIS2_PLACEMENT_3D ( 'NONE', #42326, #78693, #76480 ) ;
#24667=ADVANCED_FACE ( 'NONE', ( #73260 ), #29589, .F. ) ;
#24699=EDGE_CURVE ( 'NONE', #92620, #110694, #17021, .T. ) ;
#24767=STYLED_ITEM ( 'NONE', ( #61234 ), #82338 ) ;
#24782=CARTESIAN_POINT ( 'NONE',  ( -3.968827103576990201, 1519.551704408389924, 229.5396913781519856 ) ) ;
#24794=CARTESIAN_POINT ( 'NONE',  ( 5.864566082395450408, 1517.151704408390060, 226.1537825710409777 ) ) ;
#24797=FACE_BOUND ( 'NONE', #56701, .T. ) ;
#24806=ORIENTED_EDGE ( 'NONE', *, *, #23721, .F. ) ;
#24827=EDGE_CURVE ( 'NONE', #21719, #8025, #90345, .T. ) ;
#24851=CARTESIAN_POINT ( 'NONE',  ( -3.897009773373953490, 1519.551704408389924, 187.2231132105589211 ) ) ;
#24874=DIRECTION ( 'NONE',  ( -1.755985294532469921E-16, 1.000000000000000000, -1.338183447452831989E-16 ) ) ;
#24895=CARTESIAN_POINT ( 'NONE',  ( 12.39573405564622988, 1517.151704408390060, 218.5685989363918225 ) ) ;
#24933=ORIENTED_EDGE ( 'NONE', *, *, #53214, .F. ) ;
#24975=CIRCLE ( 'NONE', #51797, 1.999999999999998668 ) ;
#24997=ORIENTED_EDGE ( 'NONE', *, *, #60815, .F. ) ;
#25014=DIRECTION ( 'NONE',  ( 1.755985294532469921E-16, -1.000000000000000000, 1.338183447452831989E-16 ) ) ;
#25037=DIRECTION ( 'NONE',  ( -1.755985294532469921E-16, 1.000000000000000000, -1.338183447452831989E-16 ) ) ;
#25055=LINE ( 'NONE', #83328, #2764 ) ;
#25091=AXIS2_PLACEMENT_3D ( 'NONE', #43823, #105388, #10212 ) ;
#25108=DIRECTION ( 'NONE',  ( 1.755985294532464991E-16, -1.000000000000000000, 1.338183447452830017E-16 ) ) ;
#25149=CARTESIAN_POINT ( 'NONE',  ( 5.257080573758883268, 1517.051704408389924, 218.9984329930441902 ) ) ;
#25150=DIRECTION ( 'NONE',  ( -1.755985294532469921E-16, 1.000000000000000000, -1.338183447452831989E-16 ) ) ;
#25190=DIRECTION ( 'NONE',  ( 1.755985294532469921E-16, -1.000000000000000000, 1.338183447452831989E-16 ) ) ;
#25207=DIRECTION ( 'NONE',  ( -0.6736849260863841948, 0.000000000000000000, 0.7390186874254148774 ) ) ;
#25254=DIRECTION ( 'NONE',  ( -0.9455185755993178454, 0.000000000000000000, 0.3255681544571537578 ) ) ;
#25288=ORIENTED_EDGE ( 'NONE', *, *, #47457, .F. ) ;
#25321=CARTESIAN_POINT ( 'NONE',  ( 2.562340869413361588, 1522.051704408389924, 221.9545077427458182 ) ) ;
#25323=CIRCLE ( 'NONE', #367, 2.000000000000003553 ) ;
#25337=VECTOR ( 'NONE', #47638, 1000.000000000000000 ) ;
#25343=EDGE_CURVE ( 'NONE', #61158, #47444, #92198, .T. ) ;
#25356=FACE_BOUND ( 'NONE', #91217, .T. ) ;
#25369=DIRECTION ( 'NONE',  ( 1.755985294532464991E-16, -1.000000000000000000, 1.338183447452830017E-16 ) ) ;
#25372=CIRCLE ( 'NONE', #70116, 1.999999999999999556 ) ;
#25404=DIRECTION ( 'NONE',  ( -0.6736849260863841948, 0.000000000000000000, 0.7390186874254148774 ) ) ;
#25421=EDGE_CURVE ( 'NONE', #87307, #78370, #22467, .T. ) ;
#25452=CARTESIAN_POINT ( 'NONE',  ( -9.604690719327259566E-16, 1522.051704408389924, 209.1218459616989946 ) ) ;
#25456=EDGE_CURVE ( 'NONE', #67122, #105161, #81785, .T. ) ;
#25465=EDGE_CURVE ( 'NONE', #46523, #101208, #99370, .T. ) ;
#25473=DIRECTION ( 'NONE',  ( -0.6736849260863839728, 0.000000000000000000, 0.7390186874254150995 ) ) ;
#25489=CARTESIAN_POINT ( 'NONE',  ( 3.082439592801790006E-16, 1517.051704408389924, 209.1218459616989946 ) ) ;
#25494=CARTESIAN_POINT ( 'NONE',  ( -10.47043688597563182, 1522.051704408389924, 221.2386401010601844 ) ) ;
#25507=CARTESIAN_POINT ( 'NONE',  ( 11.15120484727999894, 1522.051704408389924, 220.1441346914401720 ) ) ;
#25564=DIRECTION ( 'NONE',  ( -5.980589973904019347E-17, 1.000000000000000000, -1.736889445713099699E-16 ) ) ;
#25588=CARTESIAN_POINT ( 'NONE',  ( -19.05930086066416962, 1519.551704408389924, 223.0490131529958262 ) ) ;
#25589=ADVANCED_FACE ( 'NONE', ( #87189 ), #18306, .F. ) ;
#25600=DIRECTION ( 'NONE',  ( 0.9455185755993178454, 0.000000000000000000, -0.3255681544571537578 ) ) ;
#25604=CARTESIAN_POINT ( 'NONE',  ( 19.02974267272306719, 1522.051704408389924, 211.0809136819971741 ) ) ;
#25628=ORIENTED_EDGE ( 'NONE', *, *, #35575, .T. ) ;
#25646=VECTOR ( 'NONE', #105649, 1000.000000000000000 ) ;
#25647=ORIENTED_EDGE ( 'NONE', *, *, #13471, .T. ) ;
#25660=CARTESIAN_POINT ( 'NONE',  ( -13.74310390781900004, 1517.151704408390060, 201.1531303618569950 ) ) ;
#25661=DIRECTION ( 'NONE',  ( 0.3255681544571546460, 0.000000000000000000, 0.9455185755993176233 ) ) ;
#25668=ORIENTED_EDGE ( 'NONE', *, *, #832, .F. ) ;
#25680=VERTEX_POINT ( 'NONE', #55264 ) ;
#25683=CARTESIAN_POINT ( 'NONE',  ( 1.984413551915469975, 1517.051704408389924, 198.9129232538419956 ) ) ;
#25715=AXIS2_PLACEMENT_3D ( 'NONE', #60406, #77205, #23995 ) ;
#25735=CARTESIAN_POINT ( 'NONE',  ( -10.41132050640263174, 1519.551704408389924, 189.4661702785461728 ) ) ;
#25738=VERTEX_POINT ( 'NONE', #7586 ) ;
#25751=CIRCLE ( 'NONE', #70493, 2.000000000000003109 ) ;
#25759=EDGE_LOOP ( 'NONE', ( #64883, #27264, #85845, #47625, #32133 ) ) ;
#25774=CYLINDRICAL_SURFACE ( 'NONE', #35768, 2.000000000000003553 ) ;
#25780=LINE ( 'NONE', #94655, #95641 ) ;
#25800=VECTOR ( 'NONE', #109309, 1000.000000000000000 ) ;
#25833=AXIS2_PLACEMENT_3D ( 'NONE', #25452, #1962, #36099 ) ;
#25843=DIRECTION ( 'NONE',  ( 0.9858563016923833633, 0.000000000000000000, 0.1675928173085483863 ) ) ;
#25910=FACE_BOUND ( 'NONE', #28542, .T. ) ;
#25921=CIRCLE ( 'NONE', #88537, 1.999999999999999556 ) ;
#25963=DIRECTION ( 'NONE',  ( 1.755985294532469921E-16, -1.000000000000000000, 1.338183447452831989E-16 ) ) ;
#25985=ORIENTED_EDGE ( 'NONE', *, *, #93387, .T. ) ;
#26041=VERTEX_POINT ( 'NONE', #2955 ) ;
#26057=CARTESIAN_POINT ( 'NONE',  ( -17.71193100849139768, 1519.551704408389924, 221.5709757781449980 ) ) ;
#26068=EDGE_CURVE ( 'NONE', #75258, #93813, #12958, .T. ) ;
#26069=DIRECTION ( 'NONE',  ( -0.9455185755993178454, 0.000000000000000000, 0.3255681544571537578 ) ) ;
#26071=EDGE_CURVE ( 'NONE', #25680, #10167, #79651, .T. ) ;
#26072=EDGE_CURVE ( 'NONE', #63587, #97374, #96997, .T. ) ;
#26083=CARTESIAN_POINT ( 'NONE',  ( -13.72624666517843472, 1517.051704408389924, 195.8110037935180969 ) ) ;
#26084=CARTESIAN_POINT ( 'NONE',  ( -5.316196955749759923, 1519.551704408389924, 231.0177287530028423 ) ) ;
#26102=EDGE_LOOP ( 'NONE', ( #92320, #32591, #8411, #95647 ) ) ;
#26112=CARTESIAN_POINT ( 'NONE',  ( 12.42529224677513078, 1522.051704408389924, 202.6823640254548309 ) ) ;
#26120=ORIENTED_EDGE ( 'NONE', *, *, #109746, .T. ) ;
#26137=ORIENTED_EDGE ( 'NONE', *, *, #53997, .F. ) ;
#26162=ORIENTED_EDGE ( 'NONE', *, *, #35860, .T. ) ;
#26209=CARTESIAN_POINT ( 'NONE',  ( -11.75869035857540013, 1517.151704408390060, 190.9442076533970010 ) ) ;
#26216=FACE_OUTER_BOUND ( 'NONE', #39165, .T. ) ;
#26242=DIRECTION ( 'NONE',  ( 5.980589973904019347E-17, -1.000000000000000000, 1.736889445713099699E-16 ) ) ;
#26256=AXIS2_PLACEMENT_3D ( 'NONE', #73800, #63218, #97325 ) ;
#26293=DIRECTION ( 'NONE',  ( -0.6736849260863840838, 0.000000000000000000, 0.7390186874254150995 ) ) ;
#26531=CARTESIAN_POINT ( 'NONE',  ( -10.44087869485973030, 1517.051704408389924, 205.3524051900861593 ) ) ;
#26533=CIRCLE ( 'NONE', #22906, 1.999999999999999556 ) ;
#26538=AXIS2_PLACEMENT_3D ( 'NONE', #25683, #50377, #110808 ) ;
#26546=ORIENTED_EDGE ( 'NONE', *, *, #65359, .F. ) ;
#26583=DIRECTION ( 'NONE',  ( -5.980589973904019347E-17, 1.000000000000000000, -1.736889445713099699E-16 ) ) ;
#26603=FACE_BOUND ( 'NONE', #31733, .T. ) ;
#26610=CARTESIAN_POINT ( 'NONE',  ( 1.376928043298433657, 1522.051704408389924, 191.7575736759021936 ) ) ;
#26634=AXIS2_PLACEMENT_3D ( 'NONE', #21400, #13552, #104462 ) ;
#26649=DIRECTION ( 'NONE',  ( -1.755985294532469921E-16, 1.000000000000000000, -1.338183447452831989E-16 ) ) ;
#26665=AXIS2_PLACEMENT_3D ( 'NONE', #88024, #70690, #22270 ) ;
#26682=ORIENTED_EDGE ( 'NONE', *, *, #15394, .F. ) ;
#26685=AXIS2_PLACEMENT_3D ( 'NONE', #18588, #28115, #95327 ) ;
#26745=CARTESIAN_POINT ( 'NONE',  ( -15.69795926999090163, 1517.151704408390060, 195.4758181584410011 ) ) ;
#26754=AXIS2_PLACEMENT_3D ( 'NONE', #91162, #75490, #48634 ) ;
#26759=ADVANCED_FACE ( 'NONE', ( #34474 ), #43988, .F. ) ;
#26763=CARTESIAN_POINT ( 'NONE',  ( -19.02974267272307074, 1517.151704408390060, 207.1627782414018100 ) ) ;
#26765=VERTEX_POINT ( 'NONE', #68649 ) ;
#26770=DIRECTION ( 'NONE',  ( -0.9455185755993178454, 0.000000000000000000, 0.3255681544571539243 ) ) ;
#26803=ORIENTED_EDGE ( 'NONE', *, *, #27666, .T. ) ;
#26826=CARTESIAN_POINT ( 'NONE',  ( -10.47043688597563005, 1517.151704408390060, 221.2386401010601844 ) ) ;
#26868=ORIENTED_EDGE ( 'NONE', *, *, #91727, .T. ) ;
#26879=CARTESIAN_POINT ( 'NONE',  ( 8.456465142934458612, 1517.151704408390060, 223.1002094411418284 ) ) ;
#26925=EDGE_LOOP ( 'NONE', ( #19205, #68043, #48703, #97952, #87708 ) ) ;
#26970=ORIENTED_EDGE ( 'NONE', *, *, #89715, .T. ) ;
#26974=LINE ( 'NONE', #67341, #77004 ) ;
#26979=AXIS2_PLACEMENT_3D ( 'NONE', #107535, #54957, #3455 ) ;
#26986=CARTESIAN_POINT ( 'NONE',  ( 5.864566082395450408, 1517.051704408389924, 226.1537825710409777 ) ) ;
#27007=ADVANCED_FACE ( 'NONE', ( #29254 ), #2437, .F. ) ;
#27011=ADVANCED_FACE ( 'NONE', ( #95360 ), #97563, .F. ) ;
#27015=FACE_OUTER_BOUND ( 'NONE', #11773, .T. ) ;
#27028=AXIS2_PLACEMENT_3D ( 'NONE', #9194, #35488, #110538 ) ;
#27132=DIRECTION ( 'NONE',  ( 5.980589973904019347E-17, -1.000000000000000000, 1.736889445713099699E-16 ) ) ;
#27133=DIRECTION ( 'NONE',  ( 1.755985294532469921E-16, -1.000000000000000000, 1.338183447452831989E-16 ) ) ;
#27199=VECTOR ( 'NONE', #106077, 1000.000000000000000 ) ;
#27204=ORIENTED_EDGE ( 'NONE', *, *, #39405, .T. ) ;
#27214=DIRECTION ( 'NONE',  ( 0.9455185755993178454, 0.000000000000000000, -0.3255681544571539243 ) ) ;
#27217=VERTEX_POINT ( 'NONE', #5712 ) ;
#27223=CIRCLE ( 'NONE', #66579, 1.999999999999999556 ) ;
#27261=DIRECTION ( 'NONE',  ( 5.980589973904019347E-17, -1.000000000000000000, 1.736889445713099699E-16 ) ) ;
#27264=ORIENTED_EDGE ( 'NONE', *, *, #72631, .F. ) ;
#27274=EDGE_CURVE ( 'NONE', #8025, #21719, #16964, .T. ) ;
#27324=DIRECTION ( 'NONE',  ( 1.755985294532464991E-16, -1.000000000000000000, 1.338183447452830017E-16 ) ) ;
#27330=LINE ( 'NONE', #61516, #78343 ) ;
#27371=DIRECTION ( 'NONE',  ( -5.980589973904019347E-17, 1.000000000000000000, -1.736889445713099699E-16 ) ) ;
#27403=EDGE_LOOP ( 'NONE', ( #56434, #110182 ) ) ;
#27425=DIRECTION ( 'NONE',  ( -0.9455185755993178454, 0.000000000000000000, 0.3255681544571537578 ) ) ;
#27456=CARTESIAN_POINT ( 'NONE',  ( -13.73040296198626997, 1519.551704408389924, 190.6090220189334445 ) ) ;
#27494=ADVANCED_FACE ( 'NONE', ( #44147 ), #1595, .F. ) ;
#27511=AXIS2_PLACEMENT_3D ( 'NONE', #89930, #48506, #28940 ) ;
#27567=FACE_OUTER_BOUND ( 'NONE', #52815, .T. ) ;
#27572=CARTESIAN_POINT ( 'NONE',  ( -21.60894078505574711, 1519.551704408389924, 199.6722430287886709 ) ) ;
#27581=CARTESIAN_POINT ( 'NONE',  ( -8.515581525576477517, 1517.151704408390060, 226.9159523030141372 ) ) ;
#27593=AXIS2_PLACEMENT_3D ( 'NONE', #29494, #97801, #22577 ) ;
#27595=ORIENTED_EDGE ( 'NONE', *, *, #71913, .T. ) ;
#27666=EDGE_CURVE ( 'NONE', #88646, #53816, #106440, .T. ) ;
#27679=AXIS2_PLACEMENT_3D ( 'NONE', #103400, #78220, #86071 ) ;
#27700=CARTESIAN_POINT ( 'NONE',  ( 17.66967186770163778, 1519.551704408389924, 223.1030593992828699 ) ) ;
#27715=DIRECTION ( 'NONE',  ( -5.980589973904019347E-17, 1.000000000000000000, -1.736889445713099699E-16 ) ) ;
#27726=ORIENTED_EDGE ( 'NONE', *, *, #18261, .F. ) ;
#27731=CARTESIAN_POINT ( 'NONE',  ( 15.69795926444620271, 1522.051704408389924, 222.7678737639049871 ) ) ;
#27739=ORIENTED_EDGE ( 'NONE', *, *, #29546, .T. ) ;
#27740=CARTESIAN_POINT ( 'NONE',  ( 11.83466398051542612, 1521.951704408389787, 190.1848878783540897 ) ) ;
#27754=EDGE_CURVE ( 'NONE', #54634, #64279, #67053, .T. ) ;
#27756=ADVANCED_FACE ( 'NONE', ( #87544 ), #105998, .F. ) ;
#27801=ORIENTED_EDGE ( 'NONE', *, *, #93207, .T. ) ;
#27821=ORIENTED_EDGE ( 'NONE', *, *, #84247, .T. ) ;
#27833=CIRCLE ( 'NONE', #51017, 2.000000000000003553 ) ;
#27841=CARTESIAN_POINT ( 'NONE',  ( 11.81780673814840021, 1522.051704408389924, 195.5270144474869767 ) ) ;
#27872=CIRCLE ( 'NONE', #59848, 1.999999999999999556 ) ;
#27881=DIRECTION ( 'NONE',  ( -1.755985294532469921E-16, 1.000000000000000000, -1.338183447452831989E-16 ) ) ;
#27896=LINE ( 'NONE', #63192, #90092 ) ;
#27908=AXIS2_PLACEMENT_3D ( 'NONE', #10971, #78162, #1474 ) ;
#28010=DIRECTION ( 'NONE',  ( -0.6736849260863839728, 0.000000000000000000, 0.7390186874254150995 ) ) ;
#28028=CARTESIAN_POINT ( 'NONE',  ( -5.864566082395460178, 1522.051704408389924, 192.0899093523580063 ) ) ;
#28100=ORIENTED_EDGE ( 'NONE', *, *, #61687, .F. ) ;
#28115=DIRECTION ( 'NONE',  ( 1.755985294532469921E-16, -1.000000000000000000, 1.338183447452831989E-16 ) ) ;
#28146=EDGE_LOOP ( 'NONE', ( #33907, #600, #46102, #11774, #9708 ) ) ;
#28154=ADVANCED_FACE ( 'NONE', ( #33656 ), #77888, .F. ) ;
#28167=CARTESIAN_POINT ( 'NONE',  ( -0.02955819112566700213, 1522.051704408389924, 225.0080808726450243 ) ) ;
#28216=AXIS2_PLACEMENT_3D ( 'NONE', #95311, #53325, #37607 ) ;
#28233=EDGE_CURVE ( 'NONE', #65239, #73345, #93868, .T. ) ;
#28257=VERTEX_POINT ( 'NONE', #5024 ) ;
#28277=ORIENTED_EDGE ( 'NONE', *, *, #57993, .F. ) ;
#28302=AXIS2_PLACEMENT_3D ( 'NONE', #30037, #22716, #56917 ) ;
#28348=CARTESIAN_POINT ( 'NONE',  ( 5.923682464646780943, 1517.151704408390060, 194.3813127491490036 ) ) ;
#28393=VERTEX_POINT ( 'NONE', #58747 ) ;
#28408=DIRECTION ( 'NONE',  ( 5.980589973904019347E-17, -1.000000000000000000, 1.736889445713099699E-16 ) ) ;
#28417=DIRECTION ( 'NONE',  ( -0.6736849260863841948, 0.000000000000000000, 0.7390186874254148774 ) ) ;
#28432=DIRECTION ( 'NONE',  ( -0.6736849260863840838, 0.000000000000000000, 0.7390186874254150995 ) ) ;
#28501=ORIENTED_EDGE ( 'NONE', *, *, #10758, .T. ) ;
#28542=EDGE_LOOP ( 'NONE', ( #55198, #65654 ) ) ;
#28572=CYLINDRICAL_SURFACE ( 'NONE', #15902, 1.999999999999999556 ) ;
#28579=CARTESIAN_POINT ( 'NONE',  ( 1.317811661047104010, 1517.151704408390060, 223.5300434977941677 ) ) ;
#28595=AXIS2_PLACEMENT_3D ( 'NONE', #93680, #8588, #228 ) ;
#28610=CYLINDRICAL_SURFACE ( 'NONE', #21534, 1.999999999999999556 ) ;
#28611=CARTESIAN_POINT ( 'NONE',  ( -10.26338073471560008, 1521.551704408389924, 184.6900425920350131 ) ) ;
#28626=ORIENTED_EDGE ( 'NONE', *, *, #77582, .F. ) ;
#28639=AXIS2_PLACEMENT_3D ( 'NONE', #39678, #64347, #97910 ) ;
#28678=EDGE_LOOP ( 'NONE', ( #81324, #98670, #67744, #1425, #108996 ) ) ;
#28723=ORIENTED_EDGE ( 'NONE', *, *, #15394, .T. ) ;
#28739=VERTEX_POINT ( 'NONE', #22772 ) ;
#28742=ORIENTED_EDGE ( 'NONE', *, *, #12480, .T. ) ;
#28792=CYLINDRICAL_SURFACE ( 'NONE', #32410, 1.999999999999999556 ) ;
#28803=AXIS2_PLACEMENT_3D ( 'NONE', #92377, #56047, #108083 ) ;
#28817=ORIENTED_EDGE ( 'NONE', *, *, #43571, .T. ) ;
#28879=FACE_OUTER_BOUND ( 'NONE', #67864, .T. ) ;
#28902=EDGE_CURVE ( 'NONE', #81426, #59762, #47460, .T. ) ;
#28905=CARTESIAN_POINT ( 'NONE',  ( 1.376928043298433657, 1517.051704408389924, 191.7575736759021936 ) ) ;
#28940=DIRECTION ( 'NONE',  ( -0.6736849260149578855, 0.000000000000000000, 0.7390186874905266823 ) ) ;
#28941=ADVANCED_FACE ( 'NONE', ( #68674 ), #33936, .F. ) ;
#28994=VECTOR ( 'NONE', #19932, 1000.000000000000114 ) ;
#28998=CIRCLE ( 'NONE', #20028, 1.999999999999999556 ) ;
#29045=CARTESIAN_POINT ( 'NONE',  ( 17.07488731192356823, 1517.051704408389924, 205.4036014788801481 ) ) ;
#29046=EDGE_CURVE ( 'NONE', #44418, #9574, #102896, .T. ) ;
#29050=CYLINDRICAL_SURFACE ( 'NONE', #47828, 1.999999999999999556 ) ;
#29057=EDGE_LOOP ( 'NONE', ( #34376, #103613, #34651, #24997 ) ) ;
#29093=EDGE_LOOP ( 'NONE', ( #35926, #85297, #4340, #28626 ) ) ;
#29133=FACE_OUTER_BOUND ( 'NONE', #50682, .T. ) ;
#29136=DIRECTION ( 'NONE',  ( 1.755985294532469921E-16, -1.000000000000000000, 1.338183447452831989E-16 ) ) ;
#29201=DIRECTION ( 'NONE',  ( 0.9455185755993178454, 0.000000000000000000, -0.3255681544571539243 ) ) ;
#29209=ORIENTED_EDGE ( 'NONE', *, *, #21892, .T. ) ;
#29236=DIRECTION ( 'NONE',  ( -0.6736849260863837507, 0.000000000000000000, 0.7390186874254154326 ) ) ;
#29254=FACE_OUTER_BOUND ( 'NONE', #24622, .T. ) ;
#29302=EDGE_CURVE ( 'NONE', #59762, #81426, #38563, .T. ) ;
#29311=EDGE_CURVE ( 'NONE', #21912, #110100, #22394, .T. ) ;
#29331=CARTESIAN_POINT ( 'NONE',  ( -12.42529224677513078, 1517.051704408389924, 215.5613278979431868 ) ) ;
#29340=CARTESIAN_POINT ( 'NONE',  ( -17.69507376908103424, 1517.051704408389924, 216.2288492090250998 ) ) ;
#29412=AXIS2_PLACEMENT_3D ( 'NONE', #39125, #73863, #47012 ) ;
#29446=VECTOR ( 'NONE', #92104, 1000.000000000000000 ) ;
#29466=CARTESIAN_POINT ( 'NONE',  ( 20.27427188109263057, 1517.151704408390060, 209.5053779269578342 ) ) ;
#29494=CARTESIAN_POINT ( 'NONE',  ( 0.02955819112566530210, 1522.051704408389924, 193.2356110507530218 ) ) ;
#29523=EDGE_CURVE ( 'NONE', #48957, #53407, #31373, .T. ) ;
#29532=AXIS2_PLACEMENT_3D ( 'NONE', #71998, #3683, #38886 ) ;
#29536=CARTESIAN_POINT ( 'NONE',  ( -20.27427188162093330, 1522.051704408389924, 208.7383139970561672 ) ) ;
#29544=ORIENTED_EDGE ( 'NONE', *, *, #54299, .F. ) ;
#29546=EDGE_CURVE ( 'NONE', #4755, #58393, #68982, .T. ) ;
#29589=CYLINDRICAL_SURFACE ( 'NONE', #63618, 1.999999999999999556 ) ;
#29592=EDGE_CURVE ( 'NONE', #31342, #16564, #82294, .T. ) ;
#29670=EDGE_LOOP ( 'NONE', ( #97202, #108071, #99452, #38972 ) ) ;
#29690=ORIENTED_EDGE ( 'NONE', *, *, #19116, .T. ) ;
#29691=ORIENTED_EDGE ( 'NONE', *, *, #7279, .F. ) ;
#29701=CARTESIAN_POINT ( 'NONE',  ( -9.862951376772540968, 1521.951704408389787, 228.3939896807019920 ) ) ;
#29781=CIRCLE ( 'NONE', #69136, 2.000000000000003553 ) ;
#29798=ORIENTED_EDGE ( 'NONE', *, *, #45365, .F. ) ;
#29822=AXIS2_PLACEMENT_3D ( 'NONE', #105360, #14023, #88565 ) ;
#29850=CARTESIAN_POINT ( 'NONE',  ( -1.925297167936410148, 1521.951704408389787, 187.5582988455250018 ) ) ;
#30027=VERTEX_POINT ( 'NONE', #18670 ) ;
#30037=CARTESIAN_POINT ( 'NONE',  ( -19.63722818156799832, 1522.051704408389924, 200.0074286628000095 ) ) ;
#30090=AXIS2_PLACEMENT_3D ( 'NONE', #18332, #96167, #28417 ) ;
#30105=DIRECTION ( 'NONE',  ( -0.6736849260863841948, 0.000000000000000000, 0.7390186874254148774 ) ) ;
#30117=VERTEX_POINT ( 'NONE', #88674 ) ;
#30122=CARTESIAN_POINT ( 'NONE',  ( -12.42529224677513078, 1522.051704408389924, 215.5613278979431868 ) ) ;
#30137=LINE ( 'NONE', #14432, #105199 ) ;
#30146=EDGE_CURVE ( 'NONE', #21516, #37900, #27872, .T. ) ;
#30150=ORIENTED_EDGE ( 'NONE', *, *, #110461, .T. ) ;
#30189=AXIS2_PLACEMENT_3D ( 'NONE', #87634, #27715, #36671 ) ;
#30197=VECTOR ( 'NONE', #81623, 1000.000000000000000 ) ;
#30199=DIRECTION ( 'NONE',  ( -0.6736849260863841948, 0.000000000000000000, 0.7390186874254148774 ) ) ;
#30208=ORIENTED_EDGE ( 'NONE', *, *, #61687, .T. ) ;
#30220=DIRECTION ( 'NONE',  ( -5.980589973904019347E-17, 1.000000000000000000, -1.736889445713099699E-16 ) ) ;
#30221=EDGE_CURVE ( 'NONE', #100346, #102937, #21420, .T. ) ;
#30224=ORIENTED_EDGE ( 'NONE', *, *, #100195, .F. ) ;
#30253=CIRCLE ( 'NONE', #42742, 1.999999999999998668 ) ;
#30257=ADVANCED_FACE ( 'NONE', ( #75175 ), #7400, .F. ) ;
#30303=VECTOR ( 'NONE', #34667, 1000.000000000000000 ) ;
#30311=ADVANCED_FACE ( 'NONE', ( #61154 ), #87424, .F. ) ;
#30342=VERTEX_POINT ( 'NONE', #79041 ) ;
#30348=VECTOR ( 'NONE', #60902, 1000.000000000000000 ) ;
#30363=CARTESIAN_POINT ( 'NONE',  ( -14.38014760757803145, 1522.051704408389924, 209.8840156948171511 ) ) ;
#30368=AXIS2_PLACEMENT_3D ( 'NONE', #99017, #72745, #97379 ) ;
#30375=EDGE_LOOP ( 'NONE', ( #33524, #23592 ) ) ;
#30394=DIRECTION ( 'NONE',  ( 1.755985294532464991E-16, -1.000000000000000000, 1.338183447452830017E-16 ) ) ;
#30402=DIRECTION ( 'NONE',  ( 1.755985294532464991E-16, -1.000000000000000000, 1.338183447452830017E-16 ) ) ;
#30406=AXIS2_PLACEMENT_3D ( 'NONE', #67411, #34334, #93662 ) ;
#30416=EDGE_CURVE ( 'NONE', #65907, #66063, #65538, .T. ) ;
#30430=CIRCLE ( 'NONE', #101863, 1.999999999999998668 ) ;
#30438=DIRECTION ( 'NONE',  ( -0.6736849260863839728, 0.000000000000000000, 0.7390186874254150995 ) ) ;
#30464=AXIS2_PLACEMENT_3D ( 'NONE', #102589, #60087, #77424 ) ;
#30469=FACE_BOUND ( 'NONE', #81882, .T. ) ;
#30522=AXIS2_PLACEMENT_3D ( 'NONE', #47567, #4998, #23984 ) ;
#30534=EDGE_LOOP ( 'NONE', ( #3552, #86500, #4704, #43636 ) ) ;
#30541=LINE ( 'NONE', #105613, #105813 ) ;
#30544=FACE_OUTER_BOUND ( 'NONE', #102489, .T. ) ;
#30620=CIRCLE ( 'NONE', #93189, 2.000000000000003109 ) ;
#30643=VECTOR ( 'NONE', #1351, 1000.000000000000000 ) ;
#30651=EDGE_LOOP ( 'NONE', ( #99904, #40645 ) ) ;
#30678=DIRECTION ( 'NONE',  ( 0.3255681544571569219, 1.836970198721028948E-16, 0.9455185755993167351 ) ) ;
#30710=DIRECTION ( 'NONE',  ( -1.755985294532469921E-16, 1.000000000000000000, -1.338183447452831989E-16 ) ) ;
#30776=ORIENTED_EDGE ( 'NONE', *, *, #86894, .T. ) ;
#30780=DIRECTION ( 'NONE',  ( -1.755985294532469921E-16, 1.000000000000000000, -1.338183447452831989E-16 ) ) ;
#30832=DIRECTION ( 'NONE',  ( 0.9858563016923833633, 0.000000000000000000, 0.1675928173085483863 ) ) ;
#30835=DIRECTION ( 'NONE',  ( 5.980589973904019347E-17, -1.000000000000000000, 1.736889445713099699E-16 ) ) ;
#30863=DIRECTION ( 'NONE',  ( 1.755985294532469921E-16, -1.000000000000000000, 1.338183447452831989E-16 ) ) ;
#30907=EDGE_LOOP ( 'NONE', ( #67022, #41664, #83531, #81762, #45090 ) ) ;
#30912=ADVANCED_FACE ( 'NONE', ( #55349 ), #22795, .F. ) ;
#30927=CARTESIAN_POINT ( 'NONE',  ( 7.848979634317430509, 1517.151704408390060, 215.9448598632019980 ) ) ;
#30943=EDGE_CURVE ( 'NONE', #83569, #96293, #40169, .T. ) ;
#31008=CARTESIAN_POINT ( 'NONE',  ( -5.940539704407487243, 1517.051704408389924, 229.2045057395878871 ) ) ;
#31017=FACE_BOUND ( 'NONE', #57793, .T. ) ;
#31021=ORIENTED_EDGE ( 'NONE', *, *, #38481, .F. ) ;
#31044=DIRECTION ( 'NONE',  ( 5.980589973904019347E-17, -1.000000000000000000, 1.736889445713099699E-16 ) ) ;
#31045=FACE_OUTER_BOUND ( 'NONE', #11905, .T. ) ;
#31047=CARTESIAN_POINT ( 'NONE',  ( -9.862951377749247683, 1519.551704408389924, 228.3939896778649654 ) ) ;
#31064=ORIENTED_EDGE ( 'NONE', *, *, #35168, .F. ) ;
#31086=DIRECTION ( 'NONE',  ( 1.755985294532469921E-16, -1.000000000000000000, 1.338183447452831989E-16 ) ) ;
#31091=DIRECTION ( 'NONE',  ( -0.6736849260863841948, 0.000000000000000000, 0.7390186874254148774 ) ) ;
#31092=CONICAL_SURFACE ( 'NONE', #34615, 1.000000000000007327, 0.7853981633970000820 ) ;
#31094=LINE ( 'NONE', #66933, #88881 ) ;
#31118=LINE ( 'NONE', #56337, #82070 ) ;
#31143=CARTESIAN_POINT ( 'NONE',  ( 11.78824854703250047, 1517.051704408389924, 211.4132493584619965 ) ) ;
#31148=FACE_BOUND ( 'NONE', #64850, .T. ) ;
#31155=DIRECTION ( 'NONE',  ( 5.980589973904019347E-17, -1.000000000000000000, 1.736889445713099699E-16 ) ) ;
#31168=ORIENTED_EDGE ( 'NONE', *, *, #22650, .F. ) ;
#31191=LINE ( 'NONE', #91652, #56150 ) ;
#31194=ORIENTED_EDGE ( 'NONE', *, *, #103543, .F. ) ;
#31195=EDGE_LOOP ( 'NONE', ( #81969, #47057, #2468, #5911 ) ) ;
#31202=EDGE_CURVE ( 'NONE', #33799, #21086, #65820, .T. ) ;
#31227=DIRECTION ( 'NONE',  ( -1.755985294532469921E-16, 1.000000000000000000, -1.338183447452831989E-16 ) ) ;
#31230=ORIENTED_EDGE ( 'NONE', *, *, #24172, .F. ) ;
#31232=CARTESIAN_POINT ( 'NONE',  ( 8.486023334060119439, 1517.151704408390060, 207.2139745301958271 ) ) ;
#31276=DIRECTION ( 'NONE',  ( -5.980589973904019347E-17, 1.000000000000000000, -1.736889445713099699E-16 ) ) ;
#31342=VERTEX_POINT ( 'NONE', #56675 ) ;
#31362=CIRCLE ( 'NONE', #8100, 1.999999999999999556 ) ;
#31373=CIRCLE ( 'NONE', #2799, 1.999999999999998668 ) ;
#31385=CARTESIAN_POINT ( 'NONE',  ( 21.60894078433416610, 1517.051704408389924, 218.5714488934191309 ) ) ;
#31394=CARTESIAN_POINT ( 'NONE',  ( 17.71193101166619854, 1519.551704408389924, 196.6727161458730109 ) ) ;
#31416=AXIS2_PLACEMENT_3D ( 'NONE', #39494, #3714, #13157 ) ;
#31457=ORIENTED_EDGE ( 'NONE', *, *, #47425, .F. ) ;
#31460=ORIENTED_EDGE ( 'NONE', *, *, #50753, .F. ) ;
#31476=VERTEX_POINT ( 'NONE', #54499 ) ;
#31503=EDGE_LOOP ( 'NONE', ( #23588, #76729 ) ) ;
#31573=VERTEX_POINT ( 'NONE', #74624 ) ;
#31574=VERTEX_POINT ( 'NONE', #108203 ) ;
#31585=CARTESIAN_POINT ( 'NONE',  ( 4.576312612474012553, 1517.051704408389924, 195.8593501239998318 ) ) ;
#31621=EDGE_CURVE ( 'NONE', #30027, #76210, #14134, .T. ) ;
#31629=DIRECTION ( 'NONE',  ( -1.755985294532469921E-16, 1.000000000000000000, -1.338183447452831989E-16 ) ) ;
#31637=DIRECTION ( 'NONE',  ( 1.755985294532464991E-16, -1.000000000000000000, 1.338183447452830017E-16 ) ) ;
#31651=VECTOR ( 'NONE', #18580, 1000.000000000000000 ) ;
#31672=CARTESIAN_POINT ( 'NONE',  ( 1.317811661047101346, 1522.051704408389924, 223.5300434977941677 ) ) ;
#31695=AXIS2_PLACEMENT_3D ( 'NONE', #36886, #62685, #17849 ) ;
#31700=FACE_BOUND ( 'NONE', #72519, .T. ) ;
#31706=ORIENTED_EDGE ( 'NONE', *, *, #63184, .F. ) ;
#31723=ORIENTED_EDGE ( 'NONE', *, *, #78146, .T. ) ;
#31733=EDGE_LOOP ( 'NONE', ( #23668, #12327 ) ) ;
#31743=ORIENTED_EDGE ( 'NONE', *, *, #8213, .F. ) ;
#31746=DIRECTION ( 'NONE',  ( 1.755985294532464991E-16, -1.000000000000000000, 1.338183447452830017E-16 ) ) ;
#31748=ADVANCED_FACE ( 'NONE', ( #11278 ), #37007, .F. ) ;
#31763=ORIENTED_EDGE ( 'NONE', *, *, #77661, .T. ) ;
#31779=VERTEX_POINT ( 'NONE', #39769 ) ;
#31807=EDGE_CURVE ( 'NONE', #52731, #63621, #50930, .T. ) ;
#31831=AXIS2_PLACEMENT_3D ( 'NONE', #45502, #88046, #10208 ) ;
#31855=LINE ( 'NONE', #58179, #37730 ) ;
#31863=DIRECTION ( 'NONE',  ( -5.980589973904019347E-17, 1.000000000000000000, -1.736889445713099699E-16 ) ) ;
#31864=CARTESIAN_POINT ( 'NONE',  ( 15.74021840907683512, 1521.951704408389787, 196.3375305114159062 ) ) ;
#31869=ORIENTED_EDGE ( 'NONE', *, *, #13707, .T. ) ;
#31876=VECTOR ( 'NONE', #24874, 1000.000000000000000 ) ;
#31911=ORIENTED_EDGE ( 'NONE', *, *, #100195, .T. ) ;
#31955=DIRECTION ( 'NONE',  ( -1.755985294532469921E-16, 1.000000000000000000, -1.338183447452831989E-16 ) ) ;
#32010=CARTESIAN_POINT ( 'NONE',  ( -5.864566082395460178, 1522.051704408389924, 192.0899093523580063 ) ) ;
#32056=AXIS2_PLACEMENT_3D ( 'NONE', #52918, #37209, #63007 ) ;
#32076=EDGE_LOOP ( 'NONE', ( #68817, #999 ) ) ;
#32104=AXIS2_PLACEMENT_3D ( 'NONE', #74359, #95969, #46150 ) ;
#32113=CARTESIAN_POINT ( 'NONE',  ( 9.786977753351113307, 1519.551704408389924, 226.9642986349141722 ) ) ;
#32133=ORIENTED_EDGE ( 'NONE', *, *, #67238, .F. ) ;
#32138=ORIENTED_EDGE ( 'NONE', *, *, #13231, .T. ) ;
#32140=DIRECTION ( 'NONE',  ( -5.980589973904019347E-17, 1.000000000000000000, -1.736889445713099699E-16 ) ) ;
#32238=CARTESIAN_POINT ( 'NONE',  ( 5.257080573758897479, 1522.051704408389924, 218.9984329930441618 ) ) ;
#32245=AXIS2_PLACEMENT_3D ( 'NONE', #26057, #8164, #94370 ) ;
#32266=ORIENTED_EDGE ( 'NONE', *, *, #3648, .F. ) ;
#32285=VERTEX_POINT ( 'NONE', #26112 ) ;
#32293=DIRECTION ( 'NONE',  ( 0.9455185755993178454, 0.000000000000000000, -0.3255681544571537578 ) ) ;
#32294=ORIENTED_EDGE ( 'NONE', *, *, #63283, .T. ) ;
#32326=ADVANCED_FACE ( 'NONE', ( #77105 ), #92780, .T. ) ;
#32328=ORIENTED_EDGE ( 'NONE', *, *, #35703, .T. ) ;
#32330=CIRCLE ( 'NONE', #60888, 1.999999999999999556 ) ;
#32333=EDGE_CURVE ( 'NONE', #69866, #28257, #27223, .T. ) ;
#32385=DIRECTION ( 'NONE',  ( -0.6736849260863837507, 0.000000000000000000, 0.7390186874254154326 ) ) ;
#32389=EDGE_CURVE ( 'NONE', #42621, #39431, #97194, .T. ) ;
#32410=AXIS2_PLACEMENT_3D ( 'NONE', #39798, #105500, #30832 ) ;
#32431=EDGE_CURVE ( 'NONE', #62788, #75187, #63078, .T. ) ;
#32445=ORIENTED_EDGE ( 'NONE', *, *, #63343, .F. ) ;
#32467=EDGE_CURVE ( 'NONE', #35207, #105161, #70194, .T. ) ;
#32474=VECTOR ( 'NONE', #97523, 1000.000000000000000 ) ;
#32513=DIRECTION ( 'NONE',  ( -0.9455185755993178454, 0.000000000000000000, 0.3255681544571537578 ) ) ;
#32516=ORIENTED_EDGE ( 'NONE', *, *, #68672, .T. ) ;
#32548=AXIS2_PLACEMENT_3D ( 'NONE', #51690, #743, #51138 ) ;
#32565=ADVANCED_FACE ( 'NONE', ( #30544 ), #74771, .F. ) ;
#32572=ORIENTED_EDGE ( 'NONE', *, *, #41136, .T. ) ;
#32574=DIRECTION ( 'NONE',  ( -5.980589973904019347E-17, 1.000000000000000000, -1.736889445713099699E-16 ) ) ;
#32591=ORIENTED_EDGE ( 'NONE', *, *, #48911, .F. ) ;
#32597=ORIENTED_EDGE ( 'NONE', *, *, #93088, .T. ) ;
#32600=CARTESIAN_POINT ( 'NONE',  ( -15.69795926999090163, 1522.051704408389924, 195.4758181584410011 ) ) ;
#32610=EDGE_CURVE ( 'NONE', #48164, #51456, #20095, .T. ) ;
#32612=VERTEX_POINT ( 'NONE', #2362 ) ;
#32621=EDGE_LOOP ( 'NONE', ( #44036, #67706 ) ) ;
#32631=DIRECTION ( 'NONE',  ( -1.755985294532469921E-16, 1.000000000000000000, -1.338183447452831989E-16 ) ) ;
#32647=CYLINDRICAL_SURFACE ( 'NONE', #69482, 1.999999999999999556 ) ;
#32746=DIRECTION ( 'NONE',  ( -1.755985294532469921E-16, 1.000000000000000000, -1.338183447452831989E-16 ) ) ;
#32750=DIRECTION ( 'NONE',  ( 5.980589973904019347E-17, -1.000000000000000000, 1.736889445713099699E-16 ) ) ;
#32752=CARTESIAN_POINT ( 'NONE',  ( 3.272667022753707577, 1519.551704408389924, 229.2073556998901438 ) ) ;
#32773=CARTESIAN_POINT ( 'NONE',  ( -1.925297170580940076, 1519.551704408389924, 187.5582988486569889 ) ) ;
#32803=CARTESIAN_POINT ( 'NONE',  ( -9.833393186232900263, 1517.151704408390060, 212.5077547680540135 ) ) ;
#32836=DIRECTION ( 'NONE',  ( 0.9455185755993178454, 0.000000000000000000, -0.3255681544571539243 ) ) ;
#32863=AXIS2_PLACEMENT_3D ( 'NONE', #105847, #54896, #72254 ) ;
#32918=DIRECTION ( 'NONE',  ( -0.9455185755993178454, 0.000000000000000000, 0.3255681544571537578 ) ) ;
#32920=AXIS2_PLACEMENT_3D ( 'NONE', #54132, #45730, #38393 ) ;
#32963=DIRECTION ( 'NONE',  ( -0.9455185755993178454, 0.000000000000000000, 0.3255681544571539243 ) ) ;
#32987=DIRECTION ( 'NONE',  ( -1.755985294532469921E-16, 1.000000000000000000, -1.338183447452831989E-16 ) ) ;
#33008=VECTOR ( 'NONE', #13067, 1000.000000000000000 ) ;
#33009=CYLINDRICAL_SURFACE ( 'NONE', #99902, 2.000000000000003553 ) ;
#33045=DIRECTION ( 'NONE',  ( -1.755985294532469921E-16, 1.000000000000000000, -1.338183447452831989E-16 ) ) ;
#33050=AXIS2_PLACEMENT_3D ( 'NONE', #38625, #48709, #66068 ) ;
#33056=CARTESIAN_POINT ( 'NONE',  ( 19.68364361504686855, 1519.551704408389924, 197.0079017805142030 ) ) ;
#33067=LINE ( 'NONE', #8410, #48392 ) ;
#33080=VECTOR ( 'NONE', #107480, 1000.000000000000000 ) ;
#33087=EDGE_CURVE ( 'NONE', #55445, #56930, #105969, .T. ) ;
#33128=ORIENTED_EDGE ( 'NONE', *, *, #37848, .F. ) ;
#33129=CARTESIAN_POINT ( 'NONE',  ( 8.515581525185789147, 1519.551704408389924, 191.3277396192498543 ) ) ;
#33134=DIRECTION ( 'NONE',  ( -1.755985294532469921E-16, 1.000000000000000000, -1.338183447452830017E-16 ) ) ;
#33177=DIRECTION ( 'NONE',  ( -5.980589973904019347E-17, 1.000000000000000000, -1.736889445713099699E-16 ) ) ;
#33180=EDGE_CURVE ( 'NONE', #3770, #41248, #72020, .T. ) ;
#33189=DIRECTION ( 'NONE',  ( -5.980589973904019347E-17, 1.000000000000000000, -1.736889445713099699E-16 ) ) ;
#33192=CARTESIAN_POINT ( 'NONE',  ( -22.96901158596646653, 1522.051704408389924, 211.6943887467578236 ) ) ;
#33219=CYLINDRICAL_SURFACE ( 'NONE', #87583, 2.000000000000003109 ) ;
#33222=FACE_OUTER_BOUND ( 'NONE', #68418, .T. ) ;
#33236=DIRECTION ( 'NONE',  ( 5.980589973904019347E-17, -1.000000000000000000, 1.736889445713099699E-16 ) ) ;
#33249=VERTEX_POINT ( 'NONE', #93894 ) ;
#33312=DIRECTION ( 'NONE',  ( -0.6736849260863841948, 0.000000000000000000, 0.7390186874254148774 ) ) ;
#33319=CARTESIAN_POINT ( 'NONE',  ( -6.501609782144663896, 1517.051704408389924, 200.8207946853451631 ) ) ;
#33330=EDGE_CURVE ( 'NONE', #102937, #110607, #46756, .T. ) ;
#33344=FACE_BOUND ( 'NONE', #97058, .T. ) ;
#33371=DIRECTION ( 'NONE',  ( 1.755985294532464991E-16, -1.000000000000000000, 1.338183447452830017E-16 ) ) ;
#33374=DIRECTION ( 'NONE',  ( 1.755985294532464991E-16, -1.000000000000000000, 1.338183447452830017E-16 ) ) ;
#33384=ORIENTED_EDGE ( 'NONE', *, *, #62735, .F. ) ;
#33398=EDGE_LOOP ( 'NONE', ( #30224, #83895, #48426, #92497 ) ) ;
#33409=CARTESIAN_POINT ( 'NONE',  ( -5.940539706237879969, 1519.551704408389924, 229.2045057392767262 ) ) ;
#33416=CARTESIAN_POINT ( 'NONE',  ( 3.968827103902559550, 1519.551704408389924, 188.7040005461919918 ) ) ;
#33514=CIRCLE ( 'NONE', #96123, 1.749999999999997558 ) ;
#33524=ORIENTED_EDGE ( 'NONE', *, *, #8349, .T. ) ;
#33525=LINE ( 'NONE', #58215, #83050 ) ;
#33571=AXIS2_PLACEMENT_3D ( 'NONE', #108655, #42555, #19 ) ;
#33632=AXIS2_PLACEMENT_3D ( 'NONE', #52733, #44335, #45988 ) ;
#33656=FACE_OUTER_BOUND ( 'NONE', #64054, .T. ) ;
#33704=LINE ( 'NONE', #104235, #55775 ) ;
#33746=CARTESIAN_POINT ( 'NONE',  ( -1.997114499468346294, 1519.551704408389924, 229.8748770085109072 ) ) ;
#33769=FACE_BOUND ( 'NONE', #94302, .T. ) ;
#33782=CARTESIAN_POINT ( 'NONE',  ( 3.909710721586129534, 1522.051704408389924, 220.4764703678949900 ) ) ;
#33799=VERTEX_POINT ( 'NONE', #13470 ) ;
#33806=AXIS2_PLACEMENT_3D ( 'NONE', #78316, #18941, #532 ) ;
#33886=DIRECTION ( 'NONE',  ( -1.755985294532469921E-16, 1.000000000000000000, -1.338183447452831989E-16 ) ) ;
#33906=ORIENTED_EDGE ( 'NONE', *, *, #60370, .F. ) ;
#33907=ORIENTED_EDGE ( 'NONE', *, *, #46120, .T. ) ;
#33936=CYLINDRICAL_SURFACE ( 'NONE', #56411, 2.000000000000003109 ) ;
#33956=AXIS2_PLACEMENT_3D ( 'NONE', #3820, #27324, #97288 ) ;
#33977=AXIS2_PLACEMENT_3D ( 'NONE', #5497, #39653, #98448 ) ;
#33995=AXIS2_PLACEMENT_3D ( 'NONE', #67965, #8569, #102074 ) ;
#34021=CIRCLE ( 'NONE', #73451, 2.000000000000003109 ) ;
#34037=CYLINDRICAL_SURFACE ( 'NONE', #40610, 4.000000000000006217 ) ;
#34049=CARTESIAN_POINT ( 'NONE',  ( 15.72751745975079984, 1522.051704408389924, 206.8816388537309763 ) ) ;
#34076=CARTESIAN_POINT ( 'NONE',  ( 3.331783404088237699, 1522.051704408389924, 197.4348858789911674 ) ) ;
#34079=CARTESIAN_POINT ( 'NONE',  ( 4.939530087350459949E-13, 1547.051704408389924, 209.1218459616989946 ) ) ;
#34117=CARTESIAN_POINT ( 'NONE',  ( -7.891238773387773797, 1517.051704408389924, 228.7291753153190825 ) ) ;
#34127=AXIS2_PLACEMENT_3D ( 'NONE', #99618, #14517, #49257 ) ;
#34185=EDGE_CURVE ( 'NONE', #83271, #65641, #39615, .T. ) ;
#34193=CARTESIAN_POINT ( 'NONE',  ( 9.862951377358559313, 1517.151704408390060, 189.8497022443989977 ) ) ;
#34219=ORIENTED_EDGE ( 'NONE', *, *, #102943, .T. ) ;
#34244=AXIS2_PLACEMENT_3D ( 'NONE', #9771, #60193, #35525 ) ;
#34252=DIRECTION ( 'NONE',  ( -1.755985294532469921E-16, 1.000000000000000000, -1.338183447452831989E-16 ) ) ;
#34265=FACE_OUTER_BOUND ( 'NONE', #85279, .T. ) ;
#34296=CARTESIAN_POINT ( 'NONE',  ( 2.562340869413359812, 1517.151704408390060, 221.9545077427458182 ) ) ;
#34316=EDGE_CURVE ( 'NONE', #79273, #63621, #96858, .T. ) ;
#34334=DIRECTION ( 'NONE',  ( -5.980589973904019347E-17, 1.000000000000000000, -1.736889445713099699E-16 ) ) ;
#34347=DIRECTION ( 'NONE',  ( -1.755985294532469921E-16, 1.000000000000000000, -1.338183447452831989E-16 ) ) ;
#34354=DIRECTION ( 'NONE',  ( 1.755985294532464991E-16, -1.000000000000000000, 1.338183447452830017E-16 ) ) ;
#34376=ORIENTED_EDGE ( 'NONE', *, *, #53098, .F. ) ;
#34395=DIRECTION ( 'NONE',  ( -0.9455185755993178454, 0.000000000000000000, 0.3255681544571537578 ) ) ;
#34451=EDGE_CURVE ( 'NONE', #41248, #87307, #80538, .T. ) ;
#34461=EDGE_CURVE ( 'NONE', #79544, #96193, #37430, .T. ) ;
#34474=FACE_OUTER_BOUND ( 'NONE', #11362, .T. ) ;
#34480=CARTESIAN_POINT ( 'NONE',  ( 11.78824854703250047, 1522.051704408389924, 211.4132493584619965 ) ) ;
#34508=CARTESIAN_POINT ( 'NONE',  ( 4.576312612474010777, 1517.151704408390060, 195.8593501239998318 ) ) ;
#34518=ORIENTED_EDGE ( 'NONE', *, *, #108925, .T. ) ;
#34530=DIRECTION ( 'NONE',  ( -0.9455185755993168462, -1.224646799147349756E-16, 0.3255681544571569219 ) ) ;
#34536=ORIENTED_EDGE ( 'NONE', *, *, #21249, .T. ) ;
#34545=FACE_OUTER_BOUND ( 'NONE', #55003, .T. ) ;
#34577=VERTEX_POINT ( 'NONE', #58097 ) ;
#34605=CARTESIAN_POINT ( 'NONE',  ( -11.15120484727999894, 1522.051704408389924, 198.0995572319588405 ) ) ;
#34615=AXIS2_PLACEMENT_3D ( 'NONE', #34079, #7229, #25661 ) ;
#34616=ORIENTED_EDGE ( 'NONE', *, *, #20010, .T. ) ;
#34632=DIRECTION ( 'NONE',  ( 5.980589973904019347E-17, -1.000000000000000000, 1.736889445713099699E-16 ) ) ;
#34651=ORIENTED_EDGE ( 'NONE', *, *, #72050, .F. ) ;
#34667=DIRECTION ( 'NONE',  ( -1.755985294532469921E-16, 1.000000000000000000, -1.338183447452831989E-16 ) ) ;
#34672=FACE_OUTER_BOUND ( 'NONE', #85385, .T. ) ;
#34686=CIRCLE ( 'NONE', #66930, 1.999999999999998668 ) ;
#34702=DIRECTION ( 'NONE',  ( -1.755985294532469921E-16, 1.000000000000000000, -1.338183447452831989E-16 ) ) ;
#34727=ORIENTED_EDGE ( 'NONE', *, *, #1747, .T. ) ;
#34733=EDGE_CURVE ( 'NONE', #87972, #105626, #30541, .T. ) ;
#34821=DIRECTION ( 'NONE',  ( -0.9455185755993178454, 0.000000000000000000, 0.3255681544571539243 ) ) ;
#34859=CARTESIAN_POINT ( 'NONE',  ( 9.862951377358559313, 1522.051704408389924, 189.8497022443989977 ) ) ;
#34865=CARTESIAN_POINT ( 'NONE',  ( -15.69795926856320101, 1517.051704408389924, 195.4758181589010064 ) ) ;
#34874=DIRECTION ( 'NONE',  ( -0.6736849260863839728, 0.000000000000000000, 0.7390186874254150995 ) ) ;
#34880=FILL_AREA_STYLE ('',( #43844 ) ) ;
#34885=VERTEX_POINT ( 'NONE', #98845 ) ;
#34908=DIRECTION ( 'NONE',  ( 0.9455185755993178454, 0.000000000000000000, -0.3255681544571539243 ) ) ;
#34920=EDGE_LOOP ( 'NONE', ( #20183, #54742 ) ) ;
#34933=CARTESIAN_POINT ( 'NONE',  ( -3.968827101022720072, 1517.051704408389924, 229.5396913742049776 ) ) ;
#34939=EDGE_CURVE ( 'NONE', #72223, #86431, #38927, .T. ) ;
#34958=VERTEX_POINT ( 'NONE', #6450 ) ;
#34962=AXIS2_PLACEMENT_3D ( 'NONE', #14125, #64024, #74063 ) ;
#34965=EDGE_CURVE ( 'NONE', #56930, #65868, #50659, .T. ) ;
#35031=ORIENTED_EDGE ( 'NONE', *, *, #20683, .T. ) ;
#35034=ORIENTED_EDGE ( 'NONE', *, *, #93207, .F. ) ;
#35042=ORIENTED_EDGE ( 'NONE', *, *, #24827, .T. ) ;
#35043=DIRECTION ( 'NONE',  ( -5.980589973904019347E-17, 1.000000000000000000, -1.736889445713099699E-16 ) ) ;
#35107=VERTEX_POINT ( 'NONE', #3048 ) ;
#35168=EDGE_CURVE ( 'NONE', #26765, #88934, #95086, .T. ) ;
#35207=VERTEX_POINT ( 'NONE', #22531 ) ;
#35213=ADVANCED_FACE ( 'NONE', ( #74640 ), #41583, .F. ) ;
#35227=CARTESIAN_POINT ( 'NONE',  ( 13.74310390781900004, 1517.051704408389924, 217.0905615615409943 ) ) ;
#35253=EDGE_CURVE ( 'NONE', #34958, #48781, #43228, .T. ) ;
#35281=DIRECTION ( 'NONE',  ( -5.980589973904019347E-17, 1.000000000000000000, -1.736889445713099699E-16 ) ) ;
#35325=DIRECTION ( 'NONE',  ( -1.755985294532469921E-16, 1.000000000000000000, -1.338183447452831989E-16 ) ) ;
#35363=ORIENTED_EDGE ( 'NONE', *, *, #35846, .T. ) ;
#35408=CARTESIAN_POINT ( 'NONE',  ( -4.517196230222680242, 1517.151704408390060, 190.6118719775071781 ) ) ;
#35438=FACE_BOUND ( 'NONE', #11961, .T. ) ;
#35456=DIRECTION ( 'NONE',  ( 1.755985294532469921E-16, -1.000000000000000000, 1.338183447452831989E-16 ) ) ;
#35476=ORIENTED_EDGE ( 'NONE', *, *, #41765, .T. ) ;
#35488=DIRECTION ( 'NONE',  ( 5.980589973904019347E-17, -1.000000000000000000, 1.736889445713099699E-16 ) ) ;
#35504=ORIENTED_EDGE ( 'NONE', *, *, #29302, .T. ) ;
#35516=ORIENTED_EDGE ( 'NONE', *, *, #49464, .T. ) ;
#35525=DIRECTION ( 'NONE',  ( -0.6736849260863841948, 0.000000000000000000, 0.7390186874254148774 ) ) ;
#35569=CARTESIAN_POINT ( 'NONE',  ( 13.77266209894789917, 1517.151704408390060, 201.2043266506040027 ) ) ;
#35575=EDGE_CURVE ( 'NONE', #37122, #20697, #23528, .T. ) ;
#35590=DIRECTION ( 'NONE',  ( 1.755985294532464991E-16, -1.000000000000000000, 1.338183447452830017E-16 ) ) ;
#35603=CARTESIAN_POINT ( 'NONE',  ( -7.271052316819551109, 1517.151704408390060, 225.3404165491008371 ) ) ;
#35606=LINE ( 'NONE', #96634, #42226 ) ;
#35621=EDGE_LOOP ( 'NONE', ( #88782, #36241, #23209, #99049, #4664 ) ) ;
#35632=CARTESIAN_POINT ( 'NONE',  ( -19.63722818156799832, 1522.051704408389924, 200.0074286628000095 ) ) ;
#35643=AXIS2_PLACEMENT_3D ( 'NONE', #95567, #69845, #79329 ) ;
#35655=CARTESIAN_POINT ( 'NONE',  ( -11.78824854703250047, 1522.051704408389924, 206.8304425649369875 ) ) ;
#35665=VECTOR ( 'NONE', #66914, 1000.000000000000000 ) ;
#35666=CARTESIAN_POINT ( 'NONE',  ( -18.28985832939523348, 1522.051704408389924, 198.5293912879491529 ) ) ;
#35677=ORIENTED_EDGE ( 'NONE', *, *, #711, .T. ) ;
#35681=ORIENTED_EDGE ( 'NONE', *, *, #12765, .T. ) ;
#35703=EDGE_CURVE ( 'NONE', #77632, #95724, #84932, .T. ) ;
#35721=VERTEX_POINT ( 'NONE', #75999 ) ;
#35745=CARTESIAN_POINT ( 'NONE',  ( -9.833393186232889605, 1517.051704408389924, 212.5077547680540135 ) ) ;
#35748=EDGE_LOOP ( 'NONE', ( #87195, #31911, #17268, #50597 ) ) ;
#35768=AXIS2_PLACEMENT_3D ( 'NONE', #34193, #68933, #52117 ) ;
#35819=CARTESIAN_POINT ( 'NONE',  ( -1.925297170580940076, 1519.551704408389924, 187.5582988486569889 ) ) ;
#35842=CARTESIAN_POINT ( 'NONE',  ( 17.68237282055029880, 1522.051704408389924, 212.5589510568480023 ) ) ;
#35846=EDGE_CURVE ( 'NONE', #17997, #79550, #91488, .T. ) ;
#35860=EDGE_CURVE ( 'NONE', #26041, #48957, #20363, .T. ) ;
#35895=CIRCLE ( 'NONE', #101964, 1.999999999999997780 ) ;
#35907=VERTEX_POINT ( 'NONE', #89239 ) ;
#35911=AXIS2_PLACEMENT_3D ( 'NONE', #86242, #85686, #9533 ) ;
#35926=ORIENTED_EDGE ( 'NONE', *, *, #26071, .F. ) ;
#35999=( NAMED_UNIT ( * ) PLANE_ANGLE_UNIT ( ) SI_UNIT ( $, .RADIAN. ) );
#36005=ORIENTED_EDGE ( 'NONE', *, *, #89059, .T. ) ;
#36010=VERTEX_POINT ( 'NONE', #22546 ) ;
#36013=DIRECTION ( 'NONE',  ( 0.9455185755993178454, 0.000000000000000000, -0.3255681544571539243 ) ) ;
#36026=DIRECTION ( 'NONE',  ( -0.9455185755993178454, 0.000000000000000000, 0.3255681544571537578 ) ) ;
#36064=DIRECTION ( 'NONE',  ( -0.6736849260863837507, 0.000000000000000000, 0.7390186874254154326 ) ) ;
#36071=VERTEX_POINT ( 'NONE', #83577 ) ;
#36099=DIRECTION ( 'NONE',  ( -0.9455185755993178454, 0.000000000000000000, 0.3255681544571539243 ) ) ;
#36100=EDGE_LOOP ( 'NONE', ( #76286, #99061, #19882, #94695 ) ) ;
#36115=AXIS2_PLACEMENT_3D ( 'NONE', #91765, #48135, #100709 ) ;
#36164=AXIS2_PLACEMENT_3D ( 'NONE', #52624, #36907, #71669 ) ;
#36196=CARTESIAN_POINT ( 'NONE',  ( -15.12003195112067111, 1517.151704408390060, 218.5174026476448432 ) ) ;
#36241=ORIENTED_EDGE ( 'NONE', *, *, #98660, .T. ) ;
#36263=DIRECTION ( 'NONE',  ( -0.6736849260863841948, 0.000000000000000000, 0.7390186874254148774 ) ) ;
#36306=EDGE_LOOP ( 'NONE', ( #9288, #66009, #44678, #89397 ) ) ;
#36356=CARTESIAN_POINT ( 'NONE',  ( -7.211935934568223239, 1522.051704408389924, 193.5679467272088345 ) ) ;
#36372=AXIS2_PLACEMENT_3D ( 'NONE', #69037, #33189, #60633 ) ;
#36382=ADVANCED_FACE ( 'NONE', ( #3472 ), #105920, .F. ) ;
#36403=ORIENTED_EDGE ( 'NONE', *, *, #81129, .F. ) ;
#36417=CARTESIAN_POINT ( 'NONE',  ( -6.531167973260559201, 1517.151704408390060, 216.7070295963201829 ) ) ;
#36428=CARTESIAN_POINT ( 'NONE',  ( -9.862951377749247683, 1517.151704408390060, 228.3939896778649654 ) ) ;
#36433=ORIENTED_EDGE ( 'NONE', *, *, #10580, .T. ) ;
#36440=VERTEX_POINT ( 'NONE', #49312 ) ;
#36488=AXIS2_PLACEMENT_3D ( 'NONE', #28167, #67017, #34908 ) ;
#36571=VERTEX_POINT ( 'NONE', #54834 ) ;
#36575=DIRECTION ( 'NONE',  ( 0.9455185755993178454, 0.000000000000000000, -0.3255681544571537578 ) ) ;
#36581=LINE ( 'NONE', #70780, #66455 ) ;
#36628=AXIS2_PLACEMENT_3D ( 'NONE', #21429, #30402, #72436 ) ;
#36630=AXIS2_PLACEMENT_3D ( 'NONE', #101749, #25037, #59239 ) ;
#36671=DIRECTION ( 'NONE',  ( -0.9455185755993167351, 0.000000000000000000, 0.3255681544571568109 ) ) ;
#36742=AXIS2_PLACEMENT_3D ( 'NONE', #57265, #81317, #65099 ) ;
#36753=FACE_OUTER_BOUND ( 'NONE', #15600, .T. ) ;
#36755=DIRECTION ( 'NONE',  ( -0.6736849260863841948, 0.000000000000000000, 0.7390186874254148774 ) ) ;
#36769=CARTESIAN_POINT ( 'NONE',  ( -17.69507376908103424, 1521.951704408389787, 216.2288492090250998 ) ) ;
#36812=LINE ( 'NONE', #71003, #12195 ) ;
#36818=DIRECTION ( 'NONE',  ( 0.9455185755993166241, -1.675808339056839216E-14, -0.3255681544571569219 ) ) ;
#36846=CARTESIAN_POINT ( 'NONE',  ( 17.68237282055029880, 1517.051704408389924, 212.5589510568480023 ) ) ;
#36867=CARTESIAN_POINT ( 'NONE',  ( -13.10606021074817207, 1519.551704408389924, 192.4222450282478292 ) ) ;
#36882=CIRCLE ( 'NONE', #83384, 2.000000000000003553 ) ;
#36886=CARTESIAN_POINT ( 'NONE',  ( -3.968827103576990201, 1519.551704408389924, 229.5396913781519856 ) ) ;
#36907=DIRECTION ( 'NONE',  ( -1.755985294532469921E-16, 1.000000000000000000, -1.338183447452831989E-16 ) ) ;
#36922=CYLINDRICAL_SURFACE ( 'NONE', #89345, 1.999999999999999556 ) ;
#36967=EDGE_LOOP ( 'NONE', ( #85440, #107074 ) ) ;
#36971=ORIENTED_EDGE ( 'NONE', *, *, #43571, .F. ) ;
#36977=DIRECTION ( 'NONE',  ( -1.755985294532469921E-16, 1.000000000000000000, -1.338183447452831989E-16 ) ) ;
#36995=AXIS2_PLACEMENT_3D ( 'NONE', #75726, #100365, #7950 ) ;
#37007=CYLINDRICAL_SURFACE ( 'NONE', #86198, 1.999999999999999556 ) ;
#37021=CARTESIAN_POINT ( 'NONE',  ( -9.803834995107230554, 1522.051704408389924, 196.6215198571080123 ) ) ;
#37051=ORIENTED_EDGE ( 'NONE', *, *, #91784, .T. ) ;
#37063=EDGE_CURVE ( 'NONE', #98048, #43851, #83451, .T. ) ;
#37071=CYLINDRICAL_SURFACE ( 'NONE', #25091, 2.000000000000003109 ) ;
#37073=DIRECTION ( 'NONE',  ( 5.980589973904019347E-17, -1.000000000000000000, 1.736889445713099699E-16 ) ) ;
#37087=VECTOR ( 'NONE', #32631, 1000.000000000000000 ) ;
#37117=ORIENTED_EDGE ( 'NONE', *, *, #21249, .F. ) ;
#37122=VERTEX_POINT ( 'NONE', #19559 ) ;
#37126=CARTESIAN_POINT ( 'NONE',  ( -21.62164173379369814, 1517.151704408390060, 210.2163513719069954 ) ) ;
#37137=ORIENTED_EDGE ( 'NONE', *, *, #59893, .T. ) ;
#37150=DIRECTION ( 'NONE',  ( 1.755985294532469921E-16, -1.000000000000000000, 1.338183447452831989E-16 ) ) ;
#37161=EDGE_CURVE ( 'NONE', #5162, #31573, #25055, .T. ) ;
#37164=CARTESIAN_POINT ( 'NONE',  ( 2.694739704345535891, 1517.051704408389924, 206.1657712119973382 ) ) ;
#37181=ORIENTED_EDGE ( 'NONE', *, *, #46603, .T. ) ;
#37209=DIRECTION ( 'NONE',  ( -5.980589973904019347E-17, 1.000000000000000000, -1.736889445713099699E-16 ) ) ;
#37214=EDGE_CURVE ( 'NONE', #20317, #86983, #86636, .T. ) ;
#37299=CARTESIAN_POINT ( 'NONE',  ( 2.694739704345535447, 1522.051704408389924, 206.1657712119973382 ) ) ;
#37307=FACE_OUTER_BOUND ( 'NONE', #1649, .T. ) ;
#37333=CIRCLE ( 'NONE', #53421, 1.999999999999999556 ) ;
#37367=ORIENTED_EDGE ( 'NONE', *, *, #34939, .T. ) ;
#37400=ORIENTED_EDGE ( 'NONE', *, *, #711, .F. ) ;
#37413=VECTOR ( 'NONE', #109714, 1000.000000000000000 ) ;
#37419=DIRECTION ( 'NONE',  ( 0.9455185755993166241, -1.675808339056839216E-14, -0.3255681544571569219 ) ) ;
#37430=LINE ( 'NONE', #56998, #23453 ) ;
#37436=AXIS2_PLACEMENT_3D ( 'NONE', #39488, #22094, #41131 ) ;
#37443=DIRECTION ( 'NONE',  ( -1.755985294532469921E-16, 1.000000000000000000, -1.338183447452831989E-16 ) ) ;
#37481=CIRCLE ( 'NONE', #19641, 1.999999999999997780 ) ;
#37483=FACE_OUTER_BOUND ( 'NONE', #101686, .T. ) ;
#37529=EDGE_LOOP ( 'NONE', ( #71167, #36005, #66771, #93879, #84572 ) ) ;
#37540=VERTEX_POINT ( 'NONE', #108406 ) ;
#37544=ORIENTED_EDGE ( 'NONE', *, *, #6881, .T. ) ;
#37554=CARTESIAN_POINT ( 'NONE',  ( 10.44087869485973030, 1517.151704408390060, 212.8912867333128531 ) ) ;
#37602=VECTOR ( 'NONE', #10094, 1000.000000000000000 ) ;
#37607=DIRECTION ( 'NONE',  ( 0.9455185755993178454, 0.000000000000000000, -0.3255681544571539243 ) ) ;
#37641=CYLINDRICAL_SURFACE ( 'NONE', #93743, 2.000000000000003553 ) ;
#37647=AXIS2_PLACEMENT_3D ( 'NONE', #17100, #33374, #32293 ) ;
#37664=ADVANCED_FACE ( 'NONE', ( #15426 ), #40095, .F. ) ;
#37677=CIRCLE ( 'NONE', #59189, 2.000000000000003553 ) ;
#37727=ORIENTED_EDGE ( 'NONE', *, *, #42552, .T. ) ;
#37730=VECTOR ( 'NONE', #83356, 1000.000000000000000 ) ;
#37753=AXIS2_PLACEMENT_3D ( 'NONE', #8663, #75357, #109497 ) ;
#37809=CARTESIAN_POINT ( 'NONE',  ( 8.627556093114655766, 1517.551704408390151, 234.1780882150808907 ) ) ;
#37813=COLOUR_RGB ( '', 0.31764706, 0.68627451, 0.89019608) ;
#37848=EDGE_CURVE ( 'NONE', #53940, #24144, #27833, .T. ) ;
#37849=CYLINDRICAL_SURFACE ( 'NONE', #85301, 2.000000000000003553 ) ;
#37859=EDGE_LOOP ( 'NONE', ( #5369, #20163, #91253, #104324 ) ) ;
#37861=CARTESIAN_POINT ( 'NONE',  ( 15.72751745975079984, 1522.051704408389924, 206.8816388537309763 ) ) ;
#37863=AXIS2_PLACEMENT_3D ( 'NONE', #95290, #102554, #42677 ) ;
#37900=VERTEX_POINT ( 'NONE', #48106 ) ;
#37919=EDGE_CURVE ( 'NONE', #48060, #37972, #106565, .T. ) ;
#37972=VERTEX_POINT ( 'NONE', #65472 ) ;
#37979=DIRECTION ( 'NONE',  ( -1.755985294532469921E-16, 1.000000000000000000, -1.338183447452831989E-16 ) ) ;
#37987=LINE ( 'NONE', #63756, #101561 ) ;
#37997=CARTESIAN_POINT ( 'NONE',  ( -3.272667022753708466, 1522.051704408389924, 189.0363362235078171 ) ) ;
#38006=EDGE_CURVE ( 'NONE', #104414, #103300, #92003, .T. ) ;
#38141=FACE_OUTER_BOUND ( 'NONE', #45534, .T. ) ;
#38183=CARTESIAN_POINT ( 'NONE',  ( 20.98459803409886959, 1522.051704408389924, 216.7582258867871587 ) ) ;
#38190=ORIENTED_EDGE ( 'NONE', *, *, #28902, .T. ) ;
#38215=VERTEX_POINT ( 'NONE', #42322 ) ;
#38224=DIRECTION ( 'NONE',  ( 1.171491307323471973E-14, 1.000000000000000000, -1.371895365494980038E-14 ) ) ;
#38248=CYLINDRICAL_SURFACE ( 'NONE', #78607, 1.999999999999999556 ) ;
#38261=FACE_OUTER_BOUND ( 'NONE', #31195, .T. ) ;
#38282=ORIENTED_EDGE ( 'NONE', *, *, #49655, .T. ) ;
#38353=EDGE_LOOP ( 'NONE', ( #16512, #51704, #91551, #595 ) ) ;
#38389=CARTESIAN_POINT ( 'NONE',  ( 9.862951377358559313, 1519.551704408389924, 189.8497022443989977 ) ) ;
#38393=DIRECTION ( 'NONE',  ( 0.9455185755993178454, 0.000000000000000000, -0.3255681544571537578 ) ) ;
#38434=DIRECTION ( 'NONE',  ( 5.980589973904019347E-17, -1.000000000000000000, 1.736889445713099699E-16 ) ) ;
#38481=EDGE_CURVE ( 'NONE', #110436, #14535, #91499, .T. ) ;
#38507=ORIENTED_EDGE ( 'NONE', *, *, #94710, .F. ) ;
#38510=ORIENTED_EDGE ( 'NONE', *, *, #2746, .F. ) ;
#38512=DIRECTION ( 'NONE',  ( 1.755985294532469921E-16, -1.000000000000000000, 1.338183447452831989E-16 ) ) ;
#38533=CARTESIAN_POINT ( 'NONE',  ( -9.862951376772540968, 1521.951704408389787, 228.3939896807019920 ) ) ;
#38563=CIRCLE ( 'NONE', #51060, 1.999999999999999556 ) ;
#38569=DIRECTION ( 'NONE',  ( -1.755985294532469921E-16, 1.000000000000000000, -1.338183447452831989E-16 ) ) ;
#38623=EDGE_CURVE ( 'NONE', #42280, #64279, #71861, .T. ) ;
#38625=CARTESIAN_POINT ( 'NONE',  ( 5.923682464646780943, 1522.051704408389924, 194.3813127491490036 ) ) ;
#38708=DIRECTION ( 'NONE',  ( -5.980589973904019347E-17, 1.000000000000000000, -1.736889445713099699E-16 ) ) ;
#38712=DIRECTION ( 'NONE',  ( -1.755985294532469921E-16, 1.000000000000000000, -1.338183447452831989E-16 ) ) ;
#38734=ORIENTED_EDGE ( 'NONE', *, *, #71960, .T. ) ;
#38752=EDGE_CURVE ( 'NONE', #60554, #62929, #69022, .T. ) ;
#38775=FACE_OUTER_BOUND ( 'NONE', #109156, .T. ) ;
#38787=LINE ( 'NONE', #99784, #38792 ) ;
#38792=VECTOR ( 'NONE', #74618, 1000.000000000000000 ) ;
#38860=FACE_BOUND ( 'NONE', #15687, .T. ) ;
#38864=ORIENTED_EDGE ( 'NONE', *, *, #69224, .T. ) ;
#38884=ORIENTED_EDGE ( 'NONE', *, *, #42812, .F. ) ;
#38886=DIRECTION ( 'NONE',  ( -0.6736849260863841948, 0.000000000000000000, 0.7390186874254148774 ) ) ;
#38887=CIRCLE ( 'NONE', #71141, 1.999999999999999556 ) ;
#38912=VECTOR ( 'NONE', #57218, 1000.000000000000000 ) ;
#38925=DIRECTION ( 'NONE',  ( -0.6736849260863837507, 0.000000000000000000, 0.7390186874254154326 ) ) ;
#38927=LINE ( 'NONE', #4781, #55789 ) ;
#38958=AXIS2_PLACEMENT_3D ( 'NONE', #85958, #78664, #86503 ) ;
#38972=ORIENTED_EDGE ( 'NONE', *, *, #24827, .F. ) ;
#38973=DIRECTION ( 'NONE',  ( -0.6736849260863841948, 0.000000000000000000, 0.7390186874254148774 ) ) ;
#38974=EDGE_CURVE ( 'NONE', #99156, #42052, #17076, .T. ) ;
#38978=EDGE_CURVE ( 'NONE', #17947, #84814, #70807, .T. ) ;
#38985=AXIS2_PLACEMENT_3D ( 'NONE', #94711, #45443, #86864 ) ;
#38987=CARTESIAN_POINT ( 'NONE',  ( -5.134308048384249940E-13, 1492.051704408390151, 209.1218459616989946 ) ) ;
#39017=AXIS2_PLACEMENT_3D ( 'NONE', #86123, #11086, #96182 ) ;
#39023=CARTESIAN_POINT ( 'NONE',  ( 9.803834995107230554, 1517.051704408389924, 221.6221720662910002 ) ) ;
#39108=ORIENTED_EDGE ( 'NONE', *, *, #47457, .T. ) ;
#39123=ORIENTED_EDGE ( 'NONE', *, *, #3501, .T. ) ;
#39125=CARTESIAN_POINT ( 'NONE',  ( 13.74310390781900004, 1522.051704408389924, 217.0905615615409943 ) ) ;
#39151=AXIS2_PLACEMENT_3D ( 'NONE', #40867, #47627, #21832 ) ;
#39165=EDGE_LOOP ( 'NONE', ( #54504, #99069, #52384, #62998 ) ) ;
#39174=EDGE_CURVE ( 'NONE', #35107, #47910, #18931, .T. ) ;
#39195=DIRECTION ( 'NONE',  ( 5.980589973904019347E-17, -1.000000000000000000, 1.736889445713099699E-16 ) ) ;
#39258=CIRCLE ( 'NONE', #85690, 1.999999999999999556 ) ;
#39307=AXIS2_PLACEMENT_3D ( 'NONE', #96621, #21529, #90398 ) ;
#39405=EDGE_CURVE ( 'NONE', #57510, #60349, #68855, .T. ) ;
#39425=FACE_BOUND ( 'NONE', #70786, .T. ) ;
#39431=VERTEX_POINT ( 'NONE', #54002 ) ;
#39442=EDGE_CURVE ( 'NONE', #73345, #65239, #914, .T. ) ;
#39445=DIRECTION ( 'NONE',  ( 1.755985294532469921E-16, -1.000000000000000000, 1.338183447452831989E-16 ) ) ;
#39447=SHAPE_REPRESENTATION_RELATIONSHIP ( 'NONE' , 'NONE' ,  #72299, #19969 ) ;
#39488=CARTESIAN_POINT ( 'NONE',  ( 1.984413551915469975, 1517.151704408390060, 198.9129232538419956 ) ) ;
#39494=CARTESIAN_POINT ( 'NONE',  ( -19.63722818134010240, 1517.051704408389924, 200.0074286634620364 ) ) ;
#39512=CARTESIAN_POINT ( 'NONE',  ( 10.44087869485973030, 1517.051704408389924, 212.8912867333128531 ) ) ;
#39586=VERTEX_POINT ( 'NONE', #74632 ) ;
#39602=AXIS2_PLACEMENT_3D ( 'NONE', #97343, #87301, #61024 ) ;
#39604=DIRECTION ( 'NONE',  ( -1.755985294532469921E-16, 1.000000000000000000, -1.338183447452831989E-16 ) ) ;
#39607=ORIENTED_EDGE ( 'NONE', *, *, #23746, .F. ) ;
#39615=CIRCLE ( 'NONE', #102185, 1.999999999999998668 ) ;
#39632=CARTESIAN_POINT ( 'NONE',  ( 10.41132050455482982, 1519.551704408389924, 228.7775216444308342 ) ) ;
#39653=DIRECTION ( 'NONE',  ( -1.755985294532469921E-16, 1.000000000000000000, -1.338183447452831989E-16 ) ) ;
#39658=ORIENTED_EDGE ( 'NONE', *, *, #91727, .F. ) ;
#39664=FACE_OUTER_BOUND ( 'NONE', #110313, .T. ) ;
#39678=CARTESIAN_POINT ( 'NONE',  ( -19.66678637224480397, 1517.151704408390060, 215.8936635741279986 ) ) ;
#39718=ORIENTED_EDGE ( 'NONE', *, *, #70193, .T. ) ;
#39739=CARTESIAN_POINT ( 'NONE',  ( -17.68237282055029880, 1522.051704408389924, 205.6847408665509818 ) ) ;
#39752=AXIS2_PLACEMENT_3D ( 'NONE', #53178, #80573, #87321 ) ;
#39769=CARTESIAN_POINT ( 'NONE',  ( 8.486023334060121215, 1517.051704408389924, 207.2139745301958271 ) ) ;
#39778=CARTESIAN_POINT ( 'NONE',  ( -12.39573405564623165, 1517.051704408389924, 199.6750929870061668 ) ) ;
#39798=CARTESIAN_POINT ( 'NONE',  ( 9.862951377130659836, 1521.951704408389787, 189.8497022437369708 ) ) ;
#39815=DIRECTION ( 'NONE',  ( -0.9455185755993178454, 0.000000000000000000, 0.3255681544571539243 ) ) ;
#39862=EDGE_CURVE ( 'NONE', #65641, #83271, #15170, .T. ) ;
#39871=ORIENTED_EDGE ( 'NONE', *, *, #109651, .F. ) ;
#39892=ORIENTED_EDGE ( 'NONE', *, *, #55661, .T. ) ;
#39910=DIRECTION ( 'NONE',  ( 5.980589973904019347E-17, -1.000000000000000000, 1.736889445713099699E-16 ) ) ;
#39961=VERTEX_POINT ( 'NONE', #39778 ) ;
#39970=VECTOR ( 'NONE', #59519, 1000.000000000000000 ) ;
#39976=FACE_BOUND ( 'NONE', #59428, .T. ) ;
#39989=CYLINDRICAL_SURFACE ( 'NONE', #63011, 1.999999999999999556 ) ;
#40002=ORIENTED_EDGE ( 'NONE', *, *, #69911, .T. ) ;
#40017=EDGE_CURVE ( 'NONE', #102115, #20461, #16736, .T. ) ;
#40027=EDGE_CURVE ( 'NONE', #27217, #35721, #77786, .T. ) ;
#40095=CYLINDRICAL_SURFACE ( 'NONE', #11686, 2.000000000000003553 ) ;
#40104=FACE_BOUND ( 'NONE', #70573, .T. ) ;
#40147=DIRECTION ( 'NONE',  ( -0.9455185755993178454, 0.000000000000000000, 0.3255681544571537578 ) ) ;
#40169=CIRCLE ( 'NONE', #51133, 1.999999999999999556 ) ;
#40202=ORIENTED_EDGE ( 'NONE', *, *, #56349, .F. ) ;
#40231=FACE_OUTER_BOUND ( 'NONE', #217, .T. ) ;
#40235=DIRECTION ( 'NONE',  ( 1.755985294532469921E-16, -1.000000000000000000, 1.338183447452831989E-16 ) ) ;
#40259=CARTESIAN_POINT ( 'NONE',  ( -15.72751745975079984, 1522.051704408389924, 211.3620530696679793 ) ) ;
#40270=EDGE_LOOP ( 'NONE', ( #101257, #85104 ) ) ;
#40291=ORIENTED_EDGE ( 'NONE', *, *, #24196, .F. ) ;
#40296=ORIENTED_EDGE ( 'NONE', *, *, #83249, .F. ) ;
#40350=EDGE_LOOP ( 'NONE', ( #20957, #27801, #35031, #110648, #46789 ) ) ;
#40396=AXIS2_PLACEMENT_3D ( 'NONE', #63390, #47658, #29201 ) ;
#40408=AXIS2_PLACEMENT_3D ( 'NONE', #89483, #107931, #21698 ) ;
#40449=EDGE_LOOP ( 'NONE', ( #52859, #71504, #40828, #57233 ) ) ;
#40471=LINE ( 'NONE', #14714, #99809 ) ;
#40526=EDGE_CURVE ( 'NONE', #104582, #36010, #97441, .T. ) ;
#40540=EDGE_CURVE ( 'NONE', #64221, #53037, #47640, .T. ) ;
#40551=ORIENTED_EDGE ( 'NONE', *, *, #97914, .T. ) ;
#40567=VERTEX_POINT ( 'NONE', #57713 ) ;
#40610=AXIS2_PLACEMENT_3D ( 'NONE', #62033, #93931, #77705 ) ;
#40645=ORIENTED_EDGE ( 'NONE', *, *, #42077, .T. ) ;
#40658=DIRECTION ( 'NONE',  ( -5.980589973904019347E-17, 1.000000000000000000, -1.736889445713099699E-16 ) ) ;
#40672=LINE ( 'NONE', #70882, #14293 ) ;
#40687=EDGE_CURVE ( 'NONE', #4305, #64595, #18697, .T. ) ;
#40704=ORIENTED_EDGE ( 'NONE', *, *, #24131, .T. ) ;
#40741=DIRECTION ( 'NONE',  ( 5.980589973904019347E-17, -1.000000000000000000, 1.736889445713099699E-16 ) ) ;
#40754=VECTOR ( 'NONE', #12243, 1000.000000000000000 ) ;
#40770=ORIENTED_EDGE ( 'NONE', *, *, #68672, .F. ) ;
#40771=DIRECTION ( 'NONE',  ( -1.755985294532469921E-16, 1.000000000000000000, -1.338183447452831989E-16 ) ) ;
#40772=EDGE_CURVE ( 'NONE', #43851, #65447, #95606, .T. ) ;
#40774=EDGE_CURVE ( 'NONE', #39431, #76345, #73221, .T. ) ;
#40786=AXIS2_PLACEMENT_3D ( 'NONE', #45787, #12150, #22174 ) ;
#40806=CARTESIAN_POINT ( 'NONE',  ( 19.63722818094939981, 1521.951704408389787, 218.2362632588020119 ) ) ;
#40828=ORIENTED_EDGE ( 'NONE', *, *, #709, .F. ) ;
#40830=AXIS2_PLACEMENT_3D ( 'NONE', #96516, #88130, #44468 ) ;
#40836=CIRCLE ( 'NONE', #28302, 1.999999999999999556 ) ;
#40847=EDGE_LOOP ( 'NONE', ( #42100, #70051 ) ) ;
#40867=CARTESIAN_POINT ( 'NONE',  ( -4.491820960670080849E-16, 1519.551704408389924, 209.1218459616989946 ) ) ;
#40946=EDGE_LOOP ( 'NONE', ( #52416, #46670, #66602, #78297 ) ) ;
#40963=EDGE_LOOP ( 'NONE', ( #81293, #100187, #73795, #109232 ) ) ;
#40964=ORIENTED_EDGE ( 'NONE', *, *, #29311, .F. ) ;
#40982=CARTESIAN_POINT ( 'NONE',  ( -12.42529224677512900, 1517.151704408390060, 215.5613278979431868 ) ) ;
#40990=CARTESIAN_POINT ( 'NONE',  ( 21.62164173326539895, 1519.551704408389924, 208.0273405521070060 ) ) ;
#41019=DIRECTION ( 'NONE',  ( -1.755985294532469921E-16, 1.000000000000000000, -1.338183447452831989E-16 ) ) ;
#41058=ORIENTED_EDGE ( 'NONE', *, *, #35253, .F. ) ;
#41125=DIRECTION ( 'NONE',  ( 1.755985294532464991E-16, -1.000000000000000000, 1.338183447452830017E-16 ) ) ;
#41131=DIRECTION ( 'NONE',  ( -0.6736849260863839728, 0.000000000000000000, 0.7390186874254150995 ) ) ;
#41136=EDGE_CURVE ( 'NONE', #69131, #64021, #23089, .T. ) ;
#41144=CIRCLE ( 'NONE', #48278, 2.000000000000003553 ) ;
#41149=ADVANCED_FACE ( 'NONE', ( #45478 ), #19115, .F. ) ;
#41151=CIRCLE ( 'NONE', #59077, 1.999999999999999556 ) ;
#41186=CIRCLE ( 'NONE', #60873, 2.000000000000011102 ) ;
#41202=EDGE_LOOP ( 'NONE', ( #38510, #38864, #54094, #99451 ) ) ;
#41242=CARTESIAN_POINT ( 'NONE',  ( -21.63849897585056681, 1517.051704408389924, 215.5584779397909188 ) ) ;
#41248=VERTEX_POINT ( 'NONE', #108395 ) ;
#41259=ORIENTED_EDGE ( 'NONE', *, *, #80164, .T. ) ;
#41295=CARTESIAN_POINT ( 'NONE',  ( 11.75869035672759999, 1522.051704408389924, 227.2994842695800060 ) ) ;
#41315=EDGE_CURVE ( 'NONE', #60256, #1490, #108953, .T. ) ;
#41323=DIRECTION ( 'NONE',  ( -5.980589973904019347E-17, 1.000000000000000000, -1.736889445713099699E-16 ) ) ;
#41356=VERTEX_POINT ( 'NONE', #27700 ) ;
#41360=VECTOR ( 'NONE', #40771, 1000.000000000000000 ) ;
#41376=DIRECTION ( 'NONE',  ( -0.6736849260863839728, 0.000000000000000000, 0.7390186874254150995 ) ) ;
#41380=EDGE_LOOP ( 'NONE', ( #84769, #22084 ) ) ;
#41398=EDGE_LOOP ( 'NONE', ( #59713, #48714, #31706, #100853 ) ) ;
#41401=MECHANICAL_DESIGN_GEOMETRIC_PRESENTATION_REPRESENTATION('',(#75387),#93181);
#41410=VERTEX_POINT ( 'NONE', #22563 ) ;
#41443=FACE_OUTER_BOUND ( 'NONE', #73154, .T. ) ;
#41449=CARTESIAN_POINT ( 'NONE',  ( 11.75869035456349998, 1517.051704408389924, 227.2994842691620079 ) ) ;
#41452=EDGE_CURVE ( 'NONE', #69558, #25738, #14142, .T. ) ;
#41506=ORIENTED_EDGE ( 'NONE', *, *, #94723, .T. ) ;
#41511=ORIENTED_EDGE ( 'NONE', *, *, #59709, .F. ) ;
#41519=AXIS2_PLACEMENT_3D ( 'NONE', #60319, #94437, #51350 ) ;
#41531=ORIENTED_EDGE ( 'NONE', *, *, #78829, .T. ) ;
#41557=DIRECTION ( 'NONE',  ( -0.6736849260863840838, 0.000000000000000000, 0.7390186874254150995 ) ) ;
#41583=CYLINDRICAL_SURFACE ( 'NONE', #57539, 2.000000000000003553 ) ;
#41588=LINE ( 'NONE', #6860, #37087 ) ;
#41597=ADVANCED_FACE ( 'NONE', ( #27567 ), #61212, .T. ) ;
#41602=CARTESIAN_POINT ( 'NONE',  ( 0.04641543544835614876, 1521.951704408389787, 187.8934844801420923 ) ) ;
#41615=DIRECTION ( 'NONE',  ( 1.755985294532469921E-16, -1.000000000000000000, 1.338183447452831989E-16 ) ) ;
#41637=FACE_BOUND ( 'NONE', #72045, .T. ) ;
#41664=ORIENTED_EDGE ( 'NONE', *, *, #24005, .T. ) ;
#41700=CARTESIAN_POINT ( 'NONE',  ( 20.27427188109263057, 1519.551704408389924, 209.5053779269578342 ) ) ;
#41710=ORIENTED_EDGE ( 'NONE', *, *, #10108, .T. ) ;
#41732=CYLINDRICAL_SURFACE ( 'NONE', #45612, 2.000000000000003109 ) ;
#41733=DIRECTION ( 'NONE',  ( -0.9455185755993178454, 0.000000000000000000, 0.3255681544571537578 ) ) ;
#41757=FACE_BOUND ( 'NONE', #22494, .T. ) ;
#41761=CARTESIAN_POINT ( 'NONE',  ( -14.38014760757802968, 1517.151704408390060, 209.8840156948171511 ) ) ;
#41765=EDGE_CURVE ( 'NONE', #105162, #11259, #51742, .T. ) ;
#41790=EDGE_LOOP ( 'NONE', ( #24806, #104305, #84491, #47162 ) ) ;
#41853=CARTESIAN_POINT ( 'NONE',  ( -11.81780673814840021, 1522.051704408389924, 222.7166774759110126 ) ) ;
#41891=CARTESIAN_POINT ( 'NONE',  ( 18.28985832975333281, 1517.151704408390060, 219.7143006364888436 ) ) ;
#41903=DIRECTION ( 'NONE',  ( 1.755985294532464991E-16, -1.000000000000000000, 1.338183447452830017E-16 ) ) ;
#41905=DIRECTION ( 'NONE',  ( 1.755985294532464991E-16, -1.000000000000000000, 1.338183447452830017E-16 ) ) ;
#42052=VERTEX_POINT ( 'NONE', #106209 ) ;
#42077=EDGE_CURVE ( 'NONE', #75704, #49504, #42778, .T. ) ;
#42080=ORIENTED_EDGE ( 'NONE', *, *, #92483, .F. ) ;
#42085=EDGE_CURVE ( 'NONE', #24144, #96069, #49623, .T. ) ;
#42100=ORIENTED_EDGE ( 'NONE', *, *, #23843, .T. ) ;
#42112=LINE ( 'NONE', #86861, #12810 ) ;
#42131=LINE ( 'NONE', #57846, #57376 ) ;
#42203=DIRECTION ( 'NONE',  ( -0.6736849260863841948, 0.000000000000000000, 0.7390186874254148774 ) ) ;
#42215=ORIENTED_EDGE ( 'NONE', *, *, #109746, .F. ) ;
#42222=ADVANCED_FACE ( 'NONE', ( #83211 ), #81538, .F. ) ;
#42226=VECTOR ( 'NONE', #80383, 1000.000000000000000 ) ;
#42245=CIRCLE ( 'NONE', #2950, 2.000000000000003553 ) ;
#42277=CARTESIAN_POINT ( 'NONE',  ( -9.803834995107230554, 1522.051704408389924, 196.6215198571080123 ) ) ;
#42280=VERTEX_POINT ( 'NONE', #58024 ) ;
#42300=ORIENTED_EDGE ( 'NONE', *, *, #42552, .F. ) ;
#42317=ORIENTED_EDGE ( 'NONE', *, *, #50162, .T. ) ;
#42319=ADVANCED_FACE ( 'NONE', ( #108412 ), #17709, .T. ) ;
#42322=CARTESIAN_POINT ( 'NONE',  ( 12.42529224677513078, 1517.051704408389924, 202.6823640254548309 ) ) ;
#42326=CARTESIAN_POINT ( 'NONE',  ( -15.69795926999090163, 1519.551704408389924, 195.4758181584410011 ) ) ;
#42328=DIRECTION ( 'NONE',  ( 1.000000000000000000, 0.000000000000000000, 0.000000000000000000 ) ) ;
#42352=CARTESIAN_POINT ( 'NONE',  ( 8.464772015878761380, 1517.051704408389924, 233.7053289272598420 ) ) ;
#42389=EDGE_CURVE ( 'NONE', #28257, #69866, #40836, .T. ) ;
#42441=AXIS2_PLACEMENT_3D ( 'NONE', #55535, #21329, #32385 ) ;
#42501=ORIENTED_EDGE ( 'NONE', *, *, #57877, .F. ) ;
#42552=EDGE_CURVE ( 'NONE', #37540, #64955, #92627, .T. ) ;
#42555=DIRECTION ( 'NONE',  ( 5.980589973904019347E-17, -1.000000000000000000, 1.736889445713099699E-16 ) ) ;
#42562=ORIENTED_EDGE ( 'NONE', *, *, #33330, .T. ) ;
#42564=EDGE_CURVE ( 'NONE', #86539, #30027, #90876, .T. ) ;
#42570=VECTOR ( 'NONE', #49084, 1000.000000000000000 ) ;
#42579=EDGE_CURVE ( 'NONE', #49402, #48060, #110038, .T. ) ;
#42603=ORIENTED_EDGE ( 'NONE', *, *, #92897, .T. ) ;
#42621=VERTEX_POINT ( 'NONE', #110585 ) ;
#42647=VERTEX_POINT ( 'NONE', #69159 ) ;
#42672=DIRECTION ( 'NONE',  ( -0.6736849260863841948, 0.000000000000000000, 0.7390186874254148774 ) ) ;
#42677=DIRECTION ( 'NONE',  ( -0.9455185755993178454, 0.000000000000000000, 0.3255681544571539243 ) ) ;
#42678=DIRECTION ( 'NONE',  ( 5.980589973904019347E-17, -1.000000000000000000, 1.736889445713099699E-16 ) ) ;
#42693=ADVANCED_FACE ( 'NONE', ( #109369 ), #32647, .F. ) ;
#42712=CIRCLE ( 'NONE', #105291, 26.50000000000001421 ) ;
#42740=PLANE ( 'NONE',  #33995 ) ;
#42742=AXIS2_PLACEMENT_3D ( 'NONE', #22333, #31863, #83363 ) ;
#42752=DIRECTION ( 'NONE',  ( 0.9455185755993178454, 0.000000000000000000, -0.3255681544571537578 ) ) ;
#42774=VECTOR ( 'NONE', #25150, 1000.000000000000000 ) ;
#42778=CIRCLE ( 'NONE', #44620, 1.999999999999999556 ) ;
#42783=EDGE_CURVE ( 'NONE', #76345, #90388, #67925, .T. ) ;
#42789=ORIENTED_EDGE ( 'NONE', *, *, #67209, .F. ) ;
#42794=CARTESIAN_POINT ( 'NONE',  ( 3.968827103902559550, 1519.551704408389924, 188.7040005461919918 ) ) ;
#42805=ORIENTED_EDGE ( 'NONE', *, *, #67827, .F. ) ;
#42812=EDGE_CURVE ( 'NONE', #53037, #86983, #85497, .T. ) ;
#42826=CYLINDRICAL_SURFACE ( 'NONE', #94969, 1.999999999999999556 ) ;
#42841=DIRECTION ( 'NONE',  ( -0.6736849260863840838, 0.000000000000000000, 0.7390186874254150995 ) ) ;
#42890=DIRECTION ( 'NONE',  ( 0.000000000000000000, 0.000000000000000000, 1.000000000000000000 ) ) ;
#42900=EDGE_LOOP ( 'NONE', ( #95102, #81112 ) ) ;
#42927=CIRCLE ( 'NONE', #33956, 1.999999999999997780 ) ;
#42944=DIRECTION ( 'NONE',  ( 0.9455185755993178454, 0.000000000000000000, -0.3255681544571537578 ) ) ;
#42954=ORIENTED_EDGE ( 'NONE', *, *, #88424, .F. ) ;
#42955=FACE_OUTER_BOUND ( 'NONE', #108939, .T. ) ;
#42962=CIRCLE ( 'NONE', #21433, 1.999999999999997780 ) ;
#42983=PLANE ( 'NONE',  #57114 ) ;
#42988=ORIENTED_EDGE ( 'NONE', *, *, #5135, .F. ) ;
#43033=AXIS2_PLACEMENT_3D ( 'NONE', #35842, #44809, #78963 ) ;
#43044=AXIS2_PLACEMENT_3D ( 'NONE', #99254, #107680, #81355 ) ;
#43048=CARTESIAN_POINT ( 'NONE',  ( -15.72751745975079984, 1522.051704408389924, 211.3620530696679793 ) ) ;
#43049=ORIENTED_EDGE ( 'NONE', *, *, #51374, .F. ) ;
#43055=VERTEX_POINT ( 'NONE', #89528 ) ;
#43065=EDGE_LOOP ( 'NONE', ( #7423, #65864 ) ) ;
#43085=ORIENTED_EDGE ( 'NONE', *, *, #89086, .F. ) ;
#43118=ORIENTED_EDGE ( 'NONE', *, *, #89147, .F. ) ;
#43120=CIRCLE ( 'NONE', #26979, 2.000000000000003553 ) ;
#43143=ORIENTED_EDGE ( 'NONE', *, *, #53438, .F. ) ;
#43183=ORIENTED_EDGE ( 'NONE', *, *, #90855, .T. ) ;
#43209=ORIENTED_EDGE ( 'NONE', *, *, #40772, .T. ) ;
#43223=DIRECTION ( 'NONE',  ( -1.755985294532469921E-16, 1.000000000000000000, -1.338183447452831989E-16 ) ) ;
#43228=CIRCLE ( 'NONE', #9250, 1.999999999999998668 ) ;
#43302=VECTOR ( 'NONE', #1642, 1000.000000000000000 ) ;
#43348=VERTEX_POINT ( 'NONE', #81532 ) ;
#43396=ORIENTED_EDGE ( 'NONE', *, *, #84896, .T. ) ;
#43403=CARTESIAN_POINT ( 'NONE',  ( 0.6370436997427018078, 1517.051704408389924, 200.3909606286928238 ) ) ;
#43414=VERTEX_POINT ( 'NONE', #27572 ) ;
#43454=ORIENTED_EDGE ( 'NONE', *, *, #66582, .F. ) ;
#43462=VERTEX_POINT ( 'NONE', #63959 ) ;
#43571=EDGE_CURVE ( 'NONE', #104547, #38215, #26533, .T. ) ;
#43581=CIRCLE ( 'NONE', #106157, 1.999999999999999556 ) ;
#43596=DIRECTION ( 'NONE',  ( 0.9455185755993178454, 0.000000000000000000, -0.3255681544571537578 ) ) ;
#43601=FACE_OUTER_BOUND ( 'NONE', #36306, .T. ) ;
#43622=ORIENTED_EDGE ( 'NONE', *, *, #41452, .F. ) ;
#43636=ORIENTED_EDGE ( 'NONE', *, *, #88550, .F. ) ;
#43651=CIRCLE ( 'NONE', #77623, 1.999999999999999556 ) ;
#43659=CARTESIAN_POINT ( 'NONE',  ( -21.62164173379369814, 1519.551704408389924, 210.2163513719069954 ) ) ;
#43707=DIRECTION ( 'NONE',  ( -0.6736849260863841948, 0.000000000000000000, 0.7390186874254148774 ) ) ;
#43711=DIRECTION ( 'NONE',  ( -1.755985294532469921E-16, 1.000000000000000000, -1.338183447452831989E-16 ) ) ;
#43712=ORIENTED_EDGE ( 'NONE', *, *, #10108, .F. ) ;
#43740=AXIS2_PLACEMENT_3D ( 'NONE', #69856, #51932, #62009 ) ;
#43767=FACE_OUTER_BOUND ( 'NONE', #15870, .T. ) ;
#43793=DIRECTION ( 'NONE',  ( 5.980589973904019347E-17, -1.000000000000000000, 1.736889445713099699E-16 ) ) ;
#43814=DIRECTION ( 'NONE',  ( 0.9858563016923833633, 0.000000000000000000, 0.1675928173085483863 ) ) ;
#43815=AXIS2_PLACEMENT_3D ( 'NONE', #91285, #5071, #100241 ) ;
#43823=CARTESIAN_POINT ( 'NONE',  ( -3.909710721586109550, 1517.151704408390060, 197.7672215555029993 ) ) ;
#43844=FILL_AREA_STYLE_COLOUR ( '', #62329 ) ;
#43851=VERTEX_POINT ( 'NONE', #10080 ) ;
#43855=CIRCLE ( 'NONE', #61700, 1.999999999999999556 ) ;
#43868=AXIS2_PLACEMENT_3D ( 'NONE', #76781, #86280, #99 ) ;
#43871=ORIENTED_EDGE ( 'NONE', *, *, #1145, .F. ) ;
#43928=AXIS2_PLACEMENT_3D ( 'NONE', #68603, #18166, #60199 ) ;
#43971=LINE ( 'NONE', #41891, #21722 ) ;
#43988=CYLINDRICAL_SURFACE ( 'NONE', #18881, 2.000000000000003553 ) ;
#44005=EDGE_LOOP ( 'NONE', ( #7092, #57092, #100662, #98488, #86274 ) ) ;
#44036=ORIENTED_EDGE ( 'NONE', *, *, #98919, .T. ) ;
#44081=CARTESIAN_POINT ( 'NONE',  ( -9.956645445956299412, 1522.051704408389924, 185.5808665542169820 ) ) ;
#44085=EDGE_CURVE ( 'NONE', #101117, #96069, #108863, .T. ) ;
#44090=DIRECTION ( 'NONE',  ( -0.9455185755993168462, -1.224646799147349756E-16, 0.3255681544571569219 ) ) ;
#44112=CARTESIAN_POINT ( 'NONE',  ( 19.63722818094939981, 1517.051704408389924, 218.2362632588020119 ) ) ;
#44116=EDGE_CURVE ( 'NONE', #55027, #63956, #19400, .T. ) ;
#44121=ORIENTED_EDGE ( 'NONE', *, *, #40687, .F. ) ;
#44147=FACE_OUTER_BOUND ( 'NONE', #61674, .T. ) ;
#44171=DIRECTION ( 'NONE',  ( -1.744230429721540409E-14, -1.000000000000000000, -3.290755053036525162E-15 ) ) ;
#44217=EDGE_CURVE ( 'NONE', #68701, #48151, #5103, .T. ) ;
#44268=AXIS2_PLACEMENT_3D ( 'NONE', #18831, #68728, #87162 ) ;
#44273=ORIENTED_EDGE ( 'NONE', *, *, #75563, .T. ) ;
#44300=DIRECTION ( 'NONE',  ( -0.6736849260863841948, 0.000000000000000000, 0.7390186874254148774 ) ) ;
#44335=DIRECTION ( 'NONE',  ( 1.755985294532469921E-16, -1.000000000000000000, 1.338183447452831989E-16 ) ) ;
#44356=DIRECTION ( 'NONE',  ( -0.9455185755993178454, 0.000000000000000000, 0.3255681544571539243 ) ) ;
#44374=ORIENTED_EDGE ( 'NONE', *, *, #109651, .T. ) ;
#44391=AXIS2_PLACEMENT_3D ( 'NONE', #54475, #62900, #62326 ) ;
#44418=VERTEX_POINT ( 'NONE', #48540 ) ;
#44435=ORIENTED_EDGE ( 'NONE', *, *, #61025, .T. ) ;
#44440=CARTESIAN_POINT ( 'NONE',  ( -20.98459803374077026, 1519.551704408389924, 201.4854660376508377 ) ) ;
#44447=ORIENTED_EDGE ( 'NONE', *, *, #41315, .F. ) ;
#44465=AXIS2_PLACEMENT_3D ( 'NONE', #23460, #49241, #100711 ) ;
#44468=DIRECTION ( 'NONE',  ( -0.6736849260863841948, 0.000000000000000000, 0.7390186874254148774 ) ) ;
#44540=CIRCLE ( 'NONE', #14401, 1.999999999999999556 ) ;
#44572=CYLINDRICAL_SURFACE ( 'NONE', #57034, 2.000000000000003553 ) ;
#44617=AXIS2_PLACEMENT_3D ( 'NONE', #86051, #2629, #36755 ) ;
#44620=AXIS2_PLACEMENT_3D ( 'NONE', #31143, #47416, #23287 ) ;
#44623=UNCERTAINTY_MEASURE_WITH_UNIT (LENGTH_MEASURE( 1.000000000000000082E-05 ), #45674, 'distance_accuracy_value', 'NONE');
#44658=ORIENTED_EDGE ( 'NONE', *, *, #15924, .F. ) ;
#44668=EDGE_CURVE ( 'NONE', #4755, #54175, #12032, .T. ) ;
#44670=CARTESIAN_POINT ( 'NONE',  ( 8.515581525185789147, 1517.151704408390060, 191.3277396192498543 ) ) ;
#44678=ORIENTED_EDGE ( 'NONE', *, *, #22611, .T. ) ;
#44694=CYLINDRICAL_SURFACE ( 'NONE', #39017, 2.000000000000003109 ) ;
#44721=ORIENTED_EDGE ( 'NONE', *, *, #88500, .F. ) ;
#44723=EDGE_CURVE ( 'NONE', #23258, #91497, #37333, .T. ) ;
#44726=AXIS2_PLACEMENT_3D ( 'NONE', #86232, #64232, #87348 ) ;
#44758=CARTESIAN_POINT ( 'NONE',  ( 7.271052316819551109, 1517.151704408390060, 192.9032753742981470 ) ) ;
#44773=CARTESIAN_POINT ( 'NONE',  ( -1.925297167936410148, 1521.951704408389787, 187.5582988455250018 ) ) ;
#44800=VECTOR ( 'NONE', #52784, 1000.000000000000000 ) ;
#44809=DIRECTION ( 'NONE',  ( 1.755985294532464991E-16, -1.000000000000000000, 1.338183447452830017E-16 ) ) ;
#44834=ORIENTED_EDGE ( 'NONE', *, *, #12307, .T. ) ;
#44881=VECTOR ( 'NONE', #95578, 1000.000000000000000 ) ;
#44921=CARTESIAN_POINT ( 'NONE',  ( 5.923682464646780943, 1517.051704408389924, 194.3813127491490036 ) ) ;
#44935=ORIENTED_EDGE ( 'NONE', *, *, #103543, .T. ) ;
#45057=CARTESIAN_POINT ( 'NONE',  ( -19.64992912988063267, 1517.051704408389924, 210.5515370059081022 ) ) ;
#45090=ORIENTED_EDGE ( 'NONE', *, *, #78622, .F. ) ;
#45102=DIRECTION ( 'NONE',  ( 0.000000000000000000, -1.736889445713099699E-16, -1.000000000000000000 ) ) ;
#45125=EDGE_LOOP ( 'NONE', ( #102649, #25647, #94629, #49030 ) ) ;
#45126=EDGE_LOOP ( 'NONE', ( #50362, #73629 ) ) ;
#45127=CARTESIAN_POINT ( 'NONE',  ( 15.69795926444620271, 1522.051704408389924, 222.7678737639049871 ) ) ;
#45143=ORIENTED_EDGE ( 'NONE', *, *, #2344, .F. ) ;
#45145=CARTESIAN_POINT ( 'NONE',  ( 23.59335433618681677, 1519.551704408389924, 208.3625261894497385 ) ) ;
#45178=CYLINDRICAL_SURFACE ( 'NONE', #44617, 2.000000000000003553 ) ;
#45217=ORIENTED_EDGE ( 'NONE', *, *, #13448, .T. ) ;
#45229=DIRECTION ( 'NONE',  ( 0.9858563016923833633, 0.000000000000000000, 0.1675928173085483863 ) ) ;
#45256=EDGE_CURVE ( 'NONE', #18256, #80453, #31118, .T. ) ;
#45263=DIRECTION ( 'NONE',  ( -1.755985294532469921E-16, 1.000000000000000000, -1.338183447452831989E-16 ) ) ;
#45281=CARTESIAN_POINT ( 'NONE',  ( -0.5779273184081722414, 1522.051704408389924, 186.0802614738061607 ) ) ;
#45288=ORIENTED_EDGE ( 'NONE', *, *, #34733, .F. ) ;
#45309=DIRECTION ( 'NONE',  ( -0.6736849260863839728, 0.000000000000000000, 0.7390186874254150995 ) ) ;
#45332=EDGE_CURVE ( 'NONE', #42621, #6947, #10554, .T. ) ;
#45365=EDGE_CURVE ( 'NONE', #64002, #14979, #92783, .T. ) ;
#45405=ORIENTED_EDGE ( 'NONE', *, *, #46098, .T. ) ;
#45437=VECTOR ( 'NONE', #108456, 1000.000000000000114 ) ;
#45443=DIRECTION ( 'NONE',  ( -1.755985294532469921E-16, 1.000000000000000000, -1.338183447452831989E-16 ) ) ;
#45478=FACE_OUTER_BOUND ( 'NONE', #35748, .T. ) ;
#45482=CARTESIAN_POINT ( 'NONE',  ( -13.73040295794826626, 1517.051704408389924, 190.6090220196199141 ) ) ;
#45484=EDGE_CURVE ( 'NONE', #93138, #43348, #58826, .T. ) ;
#45502=CARTESIAN_POINT ( 'NONE',  ( -19.63722818156799832, 1517.151704408390060, 200.0074286628000095 ) ) ;
#45509=CARTESIAN_POINT ( 'NONE',  ( -17.66967187194796551, 1521.951704408389787, 195.1406325242839159 ) ) ;
#45510=( BOUNDED_CURVE ( )  B_SPLINE_CURVE ( 2, ( #14519, #23477, #57670 ),
 .UNSPECIFIED., .F., .F. ) 
 B_SPLINE_CURVE_WITH_KNOTS ( ( 3, 3 ),
 ( -0.2337410562555060078, -0.1572692978119380192 ),
 .UNSPECIFIED. ) 
 CURVE ( )  GEOMETRIC_REPRESENTATION_ITEM ( )  RATIONAL_B_SPLINE_CURVE ( ( 1.002760198482619991, 1.002448066741719934, 1.002044729649790078 ) ) 
 REPRESENTATION_ITEM ( '' )  );
#45534=EDGE_LOOP ( 'NONE', ( #3826, #30208, #40296, #4600, #70221 ) ) ;
#45566=ORIENTED_EDGE ( 'NONE', *, *, #38978, .T. ) ;
#45571=ORIENTED_EDGE ( 'NONE', *, *, #5075, .T. ) ;
#45609=VECTOR ( 'NONE', #8358, 1000.000000000000000 ) ;
#45612=AXIS2_PLACEMENT_3D ( 'NONE', #75891, #102178, #61332 ) ;
#45674=( LENGTH_UNIT ( ) NAMED_UNIT ( * ) SI_UNIT ( .MILLI., .METRE. ) );
#45694=CARTESIAN_POINT ( 'NONE',  ( -19.66678637224480397, 1519.551704408389924, 215.8936635741279986 ) ) ;
#45710=CIRCLE ( 'NONE', #72476, 1.999999999999998446 ) ;
#45730=DIRECTION ( 'NONE',  ( 1.755985294532464991E-16, -1.000000000000000000, 1.338183447452830017E-16 ) ) ;
#45769=ORIENTED_EDGE ( 'NONE', *, *, #45332, .F. ) ;
#45775=CARTESIAN_POINT ( 'NONE',  ( -17.66551557795533611, 1521.951704408389787, 200.3426142980791269 ) ) ;
#45780=DIRECTION ( 'NONE',  ( -0.9455185755993177343, 0.000000000000000000, 0.3255681544571540909 ) ) ;
#45785=CARTESIAN_POINT ( 'NONE',  ( 17.07488731192357179, 1517.151704408390060, 205.4036014788801481 ) ) ;
#45787=CARTESIAN_POINT ( 'NONE',  ( -11.78824854703250047, 1522.051704408389924, 206.8304425649369875 ) ) ;
#45792=ORIENTED_EDGE ( 'NONE', *, *, #17243, .F. ) ;
#45799=CARTESIAN_POINT ( 'NONE',  ( 13.72624666550403560, 1517.051704408389924, 222.4326881308259090 ) ) ;
#45810=CYLINDRICAL_SURFACE ( 'NONE', #71662, 2.000000000000003109 ) ;
#45826=ORIENTED_EDGE ( 'NONE', *, *, #57862, .T. ) ;
#45872=ORIENTED_EDGE ( 'NONE', *, *, #42783, .F. ) ;
#45928=ORIENTED_EDGE ( 'NONE', *, *, #35168, .T. ) ;
#45946=EDGE_LOOP ( 'NONE', ( #59303, #31869, #71599, #70118, #105213 ) ) ;
#45973=DIRECTION ( 'NONE',  ( 1.755985294532464991E-16, -1.000000000000000000, 1.338183447452830017E-16 ) ) ;
#45978=DIRECTION ( 'NONE',  ( 0.9858563016923833633, 0.000000000000000000, 0.1675928173085483863 ) ) ;
#45988=DIRECTION ( 'NONE',  ( -0.6736849260863841948, 0.000000000000000000, 0.7390186874254148774 ) ) ;
#45994=EDGE_CURVE ( 'NONE', #92059, #82777, #72999, .T. ) ;
#46014=AXIS2_PLACEMENT_3D ( 'NONE', #4779, #31086, #38925 ) ;
#46033=CARTESIAN_POINT ( 'NONE',  ( -11.75869035857540013, 1522.051704408389924, 190.9442076533970010 ) ) ;
#46086=EDGE_CURVE ( 'NONE', #66505, #103394, #1455, .T. ) ;
#46098=EDGE_CURVE ( 'NONE', #8434, #106669, #88753, .T. ) ;
#46101=VERTEX_POINT ( 'NONE', #79256 ) ;
#46102=ORIENTED_EDGE ( 'NONE', *, *, #44668, .T. ) ;
#46120=EDGE_CURVE ( 'NONE', #36440, #58638, #19244, .T. ) ;
#46150=DIRECTION ( 'NONE',  ( -0.6736849260863841948, 0.000000000000000000, 0.7390186874254148774 ) ) ;
#46207=ORIENTED_EDGE ( 'NONE', *, *, #73521, .F. ) ;
#46227=ORIENTED_EDGE ( 'NONE', *, *, #64587, .F. ) ;
#46232=EDGE_LOOP ( 'NONE', ( #40551, #80044 ) ) ;
#46238=AXIS2_PLACEMENT_3D ( 'NONE', #44773, #62701, #78923 ) ;
#46259=AXIS2_PLACEMENT_3D ( 'NONE', #91053, #40658, #48528 ) ;
#46269=ORIENTED_EDGE ( 'NONE', *, *, #50822, .F. ) ;
#46282=DIRECTION ( 'NONE',  ( 1.755985294532464991E-16, -1.000000000000000000, 1.338183447452830017E-16 ) ) ;
#46373=AXIS2_PLACEMENT_3D ( 'NONE', #58299, #68369, #60514 ) ;
#46378=ORIENTED_EDGE ( 'NONE', *, *, #84235, .T. ) ;
#46443=CYLINDRICAL_SURFACE ( 'NONE', #101508, 2.000000000000003109 ) ;
#46446=CIRCLE ( 'NONE', #26754, 1.999999999999999556 ) ;
#46521=CIRCLE ( 'NONE', #28595, 2.000000000000003109 ) ;
#46523=VERTEX_POINT ( 'NONE', #34076 ) ;
#46538=DIRECTION ( 'NONE',  ( 0.9858563016923833633, 0.000000000000000000, 0.1675928173085483863 ) ) ;
#46544=CARTESIAN_POINT ( 'NONE',  ( 19.05930086383896693, 1522.051704408389924, 195.1946787710221827 ) ) ;
#46549=ORIENTED_EDGE ( 'NONE', *, *, #25465, .T. ) ;
#46562=CYLINDRICAL_SURFACE ( 'NONE', #76407, 2.000000000000003553 ) ;
#46563=VECTOR ( 'NONE', #27261, 1000.000000000000000 ) ;
#46603=EDGE_CURVE ( 'NONE', #86231, #87558, #27330, .T. ) ;
#46616=CARTESIAN_POINT ( 'NONE',  ( -19.66678637224480397, 1522.051704408389924, 215.8936635741279986 ) ) ;
#46620=CARTESIAN_POINT ( 'NONE',  ( 17.07488731192356823, 1522.051704408389924, 205.4036014788801481 ) ) ;
#46670=ORIENTED_EDGE ( 'NONE', *, *, #108261, .F. ) ;
#46679=DIRECTION ( 'NONE',  ( -1.755985294532469921E-16, 1.000000000000000000, -1.338183447452831989E-16 ) ) ;
#46713=AXIS2_PLACEMENT_3D ( 'NONE', #95953, #88671, #63491 ) ;
#46736=VECTOR ( 'NONE', #83722, 1000.000000000000000 ) ;
#46756=CIRCLE ( 'NONE', #64657, 1.999999999999997780 ) ;
#46789=ORIENTED_EDGE ( 'NONE', *, *, #45256, .F. ) ;
#46834=AXIS2_PLACEMENT_3D ( 'NONE', #74092, #6854, #109882 ) ;
#46853=CARTESIAN_POINT ( 'NONE',  ( -19.68364361505096483, 1521.951704408389787, 221.2357901429078879 ) ) ;
#46958=DIRECTION ( 'NONE',  ( -1.755985294532469921E-16, 1.000000000000000000, -1.338183447452831989E-16 ) ) ;
#46987=DIRECTION ( 'NONE',  ( -0.6736849260863839728, 0.000000000000000000, 0.7390186874254150995 ) ) ;
#47012=DIRECTION ( 'NONE',  ( 0.9455185755993178454, 0.000000000000000000, -0.3255681544571537578 ) ) ;
#47033=EDGE_LOOP ( 'NONE', ( #2593, #87249 ) ) ;
#47052=ORIENTED_EDGE ( 'NONE', *, *, #107484, .T. ) ;
#47057=ORIENTED_EDGE ( 'NONE', *, *, #31202, .T. ) ;
#47090=ORIENTED_EDGE ( 'NONE', *, *, #63226, .T. ) ;
#47128=LINE ( 'NONE', #21332, #32474 ) ;
#47162=ORIENTED_EDGE ( 'NONE', *, *, #42579, .F. ) ;
#47163=ORIENTED_EDGE ( 'NONE', *, *, #49019, .F. ) ;
#47169=DIRECTION ( 'NONE',  ( -0.6736849260863841948, 0.000000000000000000, 0.7390186874254148774 ) ) ;
#47181=ORIENTED_EDGE ( 'NONE', *, *, #40526, .T. ) ;
#47182=ORIENTED_EDGE ( 'NONE', *, *, #107298, .F. ) ;
#47189=CIRCLE ( 'NONE', #27511, 2.000000000000011102 ) ;
#47199=DIRECTION ( 'NONE',  ( 1.171491307323471973E-14, 1.000000000000000000, -1.371895365494980038E-14 ) ) ;
#47201=ORIENTED_EDGE ( 'NONE', *, *, #38752, .F. ) ;
#47320=ORIENTED_EDGE ( 'NONE', *, *, #10614, .F. ) ;
#47328=CIRCLE ( 'NONE', #16908, 2.000000000000003553 ) ;
#47381=AXIS2_PLACEMENT_3D ( 'NONE', #241, #7505, #75824 ) ;
#47387=CARTESIAN_POINT ( 'NONE',  ( -7.878537825433329367, 1517.151704408390060, 218.1850669711710111 ) ) ;
#47413=AXIS2_PLACEMENT_3D ( 'NONE', #39739, #108595, #82291 ) ;
#47416=DIRECTION ( 'NONE',  ( -5.980589973904019347E-17, 1.000000000000000000, -1.736889445713099699E-16 ) ) ;
#47425=EDGE_CURVE ( 'NONE', #77064, #99465, #10477, .T. ) ;
#47444=VERTEX_POINT ( 'NONE', #8887 ) ;
#47457=EDGE_CURVE ( 'NONE', #63901, #54088, #75580, .T. ) ;
#47460=CIRCLE ( 'NONE', #13451, 1.999999999999999556 ) ;
#47464=ADVANCED_FACE ( 'NONE', ( #68293 ), #77228, .F. ) ;
#47492=CARTESIAN_POINT ( 'NONE',  ( -5.923682464646780943, 1517.051704408389924, 223.8623791742500089 ) ) ;
#47521=DIRECTION ( 'NONE',  ( -0.6736849260863841948, 0.000000000000000000, 0.7390186874254148774 ) ) ;
#47567=CARTESIAN_POINT ( 'NONE',  ( 0.02955819112566610354, 1517.151704408390060, 193.2356110507530218 ) ) ;
#47605=ADVANCED_FACE ( 'NONE', ( #53995 ), #20886, .F. ) ;
#47625=ORIENTED_EDGE ( 'NONE', *, *, #58460, .T. ) ;
#47627=DIRECTION ( 'NONE',  ( 1.755985294532469921E-16, -1.000000000000000000, 1.338183447452831989E-16 ) ) ;
#47638=DIRECTION ( 'NONE',  ( -1.755985294532469921E-16, 1.000000000000000000, -1.338183447452831989E-16 ) ) ;
#47640=LINE ( 'NONE', #74508, #58130 ) ;
#47657=CYLINDRICAL_SURFACE ( 'NONE', #92008, 1.999999999999999556 ) ;
#47658=DIRECTION ( 'NONE',  ( 1.755985294532464991E-16, -1.000000000000000000, 1.338183447452830017E-16 ) ) ;
#47709=VERTEX_POINT ( 'NONE', #95958 ) ;
#47747=ORIENTED_EDGE ( 'NONE', *, *, #56834, .F. ) ;
#47782=CIRCLE ( 'NONE', #26256, 2.000000000000003553 ) ;
#47804=CARTESIAN_POINT ( 'NONE',  ( 13.77266209894789917, 1517.051704408389924, 201.2043266506040027 ) ) ;
#47828=AXIS2_PLACEMENT_3D ( 'NONE', #38533, #98440, #80553 ) ;
#47831=FACE_BOUND ( 'NONE', #27403, .T. ) ;
#47835=ORIENTED_EDGE ( 'NONE', *, *, #39862, .F. ) ;
#47861=DIRECTION ( 'NONE',  ( -1.755985294532469921E-16, 1.000000000000000000, -1.338183447452831989E-16 ) ) ;
#47863=CARTESIAN_POINT ( 'NONE',  ( 3.331783404088237699, 1517.051704408389924, 197.4348858789911674 ) ) ;
#47887=CARTESIAN_POINT ( 'NONE',  ( 0.04641543544835657897, 1517.051704408389924, 187.8934844801420923 ) ) ;
#47910=VERTEX_POINT ( 'NONE', #91957 ) ;
#47958=CARTESIAN_POINT ( 'NONE',  ( 19.64992912776053657, 1521.951704408389787, 207.6921549199338983 ) ) ;
#47970=CARTESIAN_POINT ( 'NONE',  ( 21.62164173114529930, 1521.951704408389787, 208.0273405545509888 ) ) ;
#47995=DIRECTION ( 'NONE',  ( 0.9858563016923833633, 0.000000000000000000, 0.1675928173085483863 ) ) ;
#48000=ADVANCED_FACE ( 'NONE', ( #99239 ), #81342, .F. ) ;
#48060=VERTEX_POINT ( 'NONE', #51076 ) ;
#48070=CYLINDRICAL_SURFACE ( 'NONE', #75052, 2.000000000000003109 ) ;
#48101=AXIS2_PLACEMENT_3D ( 'NONE', #34933, #50644, #101563 ) ;
#48106=CARTESIAN_POINT ( 'NONE',  ( 18.31941652029303214, 1522.051704408389924, 203.8280657238408651 ) ) ;
#48135=DIRECTION ( 'NONE',  ( -5.980589973904019347E-17, 1.000000000000000000, -1.736889445713099699E-16 ) ) ;
#48151=VERTEX_POINT ( 'NONE', #59483 ) ;
#48155=EDGE_CURVE ( 'NONE', #35721, #78966, #51566, .T. ) ;
#48164=VERTEX_POINT ( 'NONE', #46544 ) ;
#48168=ORIENTED_EDGE ( 'NONE', *, *, #55884, .T. ) ;
#48214=CYLINDRICAL_SURFACE ( 'NONE', #8376, 1.999999999999999556 ) ;
#48278=AXIS2_PLACEMENT_3D ( 'NONE', #9158, #35456, #102628 ) ;
#48383=ORIENTED_EDGE ( 'NONE', *, *, #81902, .T. ) ;
#48392=VECTOR ( 'NONE', #67256, 1000.000000000000000 ) ;
#48397=FACE_BOUND ( 'NONE', #18115, .T. ) ;
#48414=DIRECTION ( 'NONE',  ( -0.6736849260863839728, 0.000000000000000000, 0.7390186874254150995 ) ) ;
#48417=PRESENTATION_STYLE_ASSIGNMENT (( #48971 ) ) ;
#48426=ORIENTED_EDGE ( 'NONE', *, *, #34451, .T. ) ;
#48434=ORIENTED_EDGE ( 'NONE', *, *, #10525, .T. ) ;
#48463=VECTOR ( 'NONE', #67460, 1000.000000000000000 ) ;
#48470=AXIS2_PLACEMENT_3D ( 'NONE', #69836, #70392, #70952 ) ;
#48476=LINE ( 'NONE', #75332, #31876 ) ;
#48506=DIRECTION ( 'NONE',  ( 1.755985294532469921E-16, -1.000000000000000000, 1.338183447452831989E-16 ) ) ;
#48525=DIRECTION ( 'NONE',  ( 0.9858563016923833633, 0.000000000000000000, 0.1675928173085483863 ) ) ;
#48528=DIRECTION ( 'NONE',  ( -0.9455185755993178454, 0.000000000000000000, 0.3255681544571539243 ) ) ;
#48540=CARTESIAN_POINT ( 'NONE',  ( 19.68364361584636768, 1517.051704408389924, 197.0079017806501156 ) ) ;
#48560=DIRECTION ( 'NONE',  ( 1.755985294532469921E-16, -1.000000000000000000, 1.338183447452831989E-16 ) ) ;
#48566=AXIS2_PLACEMENT_3D ( 'NONE', #83060, #56210, #66292 ) ;
#48574=VERTEX_POINT ( 'NONE', #55490 ) ;
#48623=ADVANCED_FACE ( 'NONE', ( #14554 ), #23509, .T. ) ;
#48627=ORIENTED_EDGE ( 'NONE', *, *, #86894, .F. ) ;
#48634=DIRECTION ( 'NONE',  ( -0.9455185755993178454, 0.000000000000000000, 0.3255681544571537578 ) ) ;
#48693=DIRECTION ( 'NONE',  ( 5.980589973904019347E-17, -1.000000000000000000, 1.736889445713099699E-16 ) ) ;
#48703=ORIENTED_EDGE ( 'NONE', *, *, #90107, .F. ) ;
#48709=DIRECTION ( 'NONE',  ( 1.755985294532464991E-16, -1.000000000000000000, 1.338183447452830017E-16 ) ) ;
#48714=ORIENTED_EDGE ( 'NONE', *, *, #26071, .T. ) ;
#48716=CARTESIAN_POINT ( 'NONE',  ( 4.517196230222682019, 1517.051704408389924, 227.6318199458918343 ) ) ;
#48745=ADVANCED_FACE ( 'NONE', ( #34672 ), #93461, .F. ) ;
#48749=EDGE_LOOP ( 'NONE', ( #65521, #6586, #44721, #96208 ) ) ;
#48765=ADVANCED_FACE ( 'NONE', ( #16194 ), #33009, .F. ) ;
#48770=DIRECTION ( 'NONE',  ( -1.755985294532469921E-16, 1.000000000000000000, -1.338183447452831989E-16 ) ) ;
#48781=VERTEX_POINT ( 'NONE', #25149 ) ;
#48875=EDGE_CURVE ( 'NONE', #54897, #65239, #10587, .T. ) ;
#48911=EDGE_CURVE ( 'NONE', #49402, #46101, #82004, .T. ) ;
#48932=DIRECTION ( 'NONE',  ( -1.755985294532469921E-16, 1.000000000000000000, -1.338183447452831989E-16 ) ) ;
#48948=AXIS2_PLACEMENT_3D ( 'NONE', #43048, #25108, #43596 ) ;
#48957=VERTEX_POINT ( 'NONE', #89489 ) ;
#48971=SURFACE_STYLE_USAGE ( .BOTH. , #49519 ) ;
#48992=ORIENTED_EDGE ( 'NONE', *, *, #50710, .T. ) ;
#49019=EDGE_CURVE ( 'NONE', #31779, #23279, #106291, .T. ) ;
#49030=ORIENTED_EDGE ( 'NONE', *, *, #84235, .F. ) ;
#49084=DIRECTION ( 'NONE',  ( -1.755985294532469921E-16, 1.000000000000000000, -1.338183447452831989E-16 ) ) ;
#49100=ORIENTED_EDGE ( 'NONE', *, *, #10427, .F. ) ;
#49109=CYLINDRICAL_SURFACE ( 'NONE', #65124, 1.999999999999999556 ) ;
#49121=CARTESIAN_POINT ( 'NONE',  ( 5.864566082395450408, 1522.051704408389924, 226.1537825710409777 ) ) ;
#49131=AXIS2_PLACEMENT_3D ( 'NONE', #80212, #53944, #52820 ) ;
#49193=ORIENTED_EDGE ( 'NONE', *, *, #49655, .F. ) ;
#49206=CARTESIAN_POINT ( 'NONE',  ( -20.27427188162093330, 1519.551704408389924, 208.7383139970561672 ) ) ;
#49207=DIRECTION ( 'NONE',  ( 0.3255681544571546460, 0.000000000000000000, 0.9455185755993176233 ) ) ;
#49227=CARTESIAN_POINT ( 'NONE',  ( -5.316196955749759923, 1517.151704408390060, 231.0177287530028423 ) ) ;
#49241=DIRECTION ( 'NONE',  ( -1.755985294532469921E-16, 1.000000000000000000, -1.338183447452831989E-16 ) ) ;
#49251=EDGE_LOOP ( 'NONE', ( #80363, #73826 ) ) ;
#49257=DIRECTION ( 'NONE',  ( 0.9455185755993178454, 0.000000000000000000, -0.3255681544571537578 ) ) ;
#49288=LINE ( 'NONE', #24043, #42774 ) ;
#49297=EDGE_CURVE ( 'NONE', #80453, #18655, #23004, .T. ) ;
#49312=CARTESIAN_POINT ( 'NONE',  ( 0.5779273184081700210, 1519.551704408389924, 232.1634304495918002 ) ) ;
#49339=DIRECTION ( 'NONE',  ( -0.6736849260863841948, 0.000000000000000000, 0.7390186874254148774 ) ) ;
#49362=EDGE_LOOP ( 'NONE', ( #55822, #74235, #20893, #10841, #21008 ) ) ;
#49402=VERTEX_POINT ( 'NONE', #87155 ) ;
#49409=CARTESIAN_POINT ( 'NONE',  ( -9.956645445956299412, 1519.551704408389924, 185.5808665542169820 ) ) ;
#49423=ADVANCED_FACE ( 'NONE', ( #36753 ), #52468, .F. ) ;
#49451=CIRCLE ( 'NONE', #10028, 1.999999999999999556 ) ;
#49464=EDGE_CURVE ( 'NONE', #65829, #33249, #44540, .T. ) ;
#49466=CARTESIAN_POINT ( 'NONE',  ( 7.891238773745893553, 1521.951704408389787, 189.5145166091198803 ) ) ;
#49486=DIRECTION ( 'NONE',  ( -0.6736849260863841948, 0.000000000000000000, 0.7390186874254148774 ) ) ;
#49504=VERTEX_POINT ( 'NONE', #39512 ) ;
#49519=SURFACE_SIDE_STYLE ('',( #57380 ) ) ;
#49541=ORIENTED_EDGE ( 'NONE', *, *, #35575, .F. ) ;
#49575=DIRECTION ( 'NONE',  ( 0.9455185755993178454, 0.000000000000000000, -0.3255681544571539243 ) ) ;
#49602=AXIS2_PLACEMENT_3D ( 'NONE', #83674, #84771, #25404 ) ;
#49616=ORIENTED_EDGE ( 'NONE', *, *, #8534, .F. ) ;
#49623=LINE ( 'NONE', #47958, #107186 ) ;
#49628=FACE_BOUND ( 'NONE', #74626, .T. ) ;
#49655=EDGE_CURVE ( 'NONE', #98249, #96193, #32330, .T. ) ;
#49717=CARTESIAN_POINT ( 'NONE',  ( -6.954065720117950100, 1521.551704408389924, 183.5505540514350002 ) ) ;
#49720=CYLINDRICAL_SURFACE ( 'NONE', #33977, 2.000000000000003109 ) ;
#49729=AXIS2_PLACEMENT_3D ( 'NONE', #59648, #57458, #15950 ) ;
#49780=CARTESIAN_POINT ( 'NONE',  ( -7.878537825433329367, 1517.051704408389924, 218.1850669711710111 ) ) ;
#49781=FACE_OUTER_BOUND ( 'NONE', #93668, .T. ) ;
#49785=EDGE_CURVE ( 'NONE', #99465, #101208, #6177, .T. ) ;
#49797=DIRECTION ( 'NONE',  ( 1.755985294532464991E-16, -1.000000000000000000, 1.338183447452830017E-16 ) ) ;
#49822=DIRECTION ( 'NONE',  ( 0.9858563016923833633, 0.000000000000000000, 0.1675928173085483863 ) ) ;
#49929=CARTESIAN_POINT ( 'NONE',  ( -5.923682464646780943, 1517.151704408390060, 223.8623791742500089 ) ) ;
#49954=DIRECTION ( 'NONE',  ( -0.9455185755993178454, 0.000000000000000000, 0.3255681544571539798 ) ) ;
#49998=LINE ( 'NONE', #163, #3177 ) ;
#50008=DIRECTION ( 'NONE',  ( 0.9858563016923833633, 0.000000000000000000, 0.1675928173085483863 ) ) ;
#50038=DIRECTION ( 'NONE',  ( 1.755985294532469921E-16, -1.000000000000000000, 1.338183447452831989E-16 ) ) ;
#50063=CARTESIAN_POINT ( 'NONE',  ( -11.75869035456349998, 1521.951704408389787, 190.9442076542370046 ) ) ;
#50092=VECTOR ( 'NONE', #109670, 1000.000000000000000 ) ;
#50123=AXIS2_PLACEMENT_3D ( 'NONE', #20681, #63838, #55429 ) ;
#50137=CARTESIAN_POINT ( 'NONE',  ( -19.66678637246580053, 1517.051704408389924, 215.8936635744080093 ) ) ;
#50156=VECTOR ( 'NONE', #109920, 1000.000000000000000 ) ;
#50162=EDGE_CURVE ( 'NONE', #3955, #20783, #64481, .T. ) ;
#50185=FACE_BOUND ( 'NONE', #7380, .T. ) ;
#50210=ORIENTED_EDGE ( 'NONE', *, *, #10940, .T. ) ;
#50273=CARTESIAN_POINT ( 'NONE',  ( -17.68237282055029880, 1522.051704408389924, 205.6847408665509818 ) ) ;
#50284=DIRECTION ( 'NONE',  ( -0.9455185755993178454, 0.000000000000000000, 0.3255681544571537578 ) ) ;
#50310=DIRECTION ( 'NONE',  ( -1.755985294532469921E-16, 1.000000000000000000, -1.338183447452831989E-16 ) ) ;
#50318=CYLINDRICAL_SURFACE ( 'NONE', #59348, 2.000000000000003553 ) ;
#50349=EDGE_LOOP ( 'NONE', ( #99468, #63416 ) ) ;
#50362=ORIENTED_EDGE ( 'NONE', *, *, #85403, .T. ) ;
#50365=EDGE_LOOP ( 'NONE', ( #9274, #74291, #11513, #73827 ) ) ;
#50377=DIRECTION ( 'NONE',  ( -5.980589973904019347E-17, 1.000000000000000000, -1.736889445713099699E-16 ) ) ;
#50390=CIRCLE ( 'NONE', #77161, 1.999999999999999556 ) ;
#50393=VERTEX_POINT ( 'NONE', #33409 ) ;
#50403=EDGE_CURVE ( 'NONE', #76210, #22976, #51996, .T. ) ;
#50428=EDGE_LOOP ( 'NONE', ( #82547, #13193 ) ) ;
#50463=CARTESIAN_POINT ( 'NONE',  ( 6.531167973260561865, 1517.051704408389924, 201.5366623270788295 ) ) ;
#50490=DIRECTION ( 'NONE',  ( 0.9455185755993178454, 0.000000000000000000, -0.3255681544571539243 ) ) ;
#50497=AXIS2_PLACEMENT_3D ( 'NONE', #101039, #8091, #92649 ) ;
#50537=DIRECTION ( 'NONE',  ( 0.2302114497549279104, -0.7071067811868634312, 0.6685825965438282337 ) ) ;
#50557=EDGE_CURVE ( 'NONE', #1077, #103300, #19931, .T. ) ;
#50585=CARTESIAN_POINT ( 'NONE',  ( -10.44087869485973030, 1522.051704408389924, 205.3524051900861593 ) ) ;
#50592=FACE_BOUND ( 'NONE', #102322, .T. ) ;
#50597=ORIENTED_EDGE ( 'NONE', *, *, #34451, .F. ) ;
#50639=ORIENTED_EDGE ( 'NONE', *, *, #80351, .F. ) ;
#50644=DIRECTION ( 'NONE',  ( -5.980589973904019347E-17, 1.000000000000000000, -1.736889445713099699E-16 ) ) ;
#50658=CARTESIAN_POINT ( 'NONE',  ( -8.515581525576479294, 1522.051704408389924, 226.9159523030141372 ) ) ;
#50659=LINE ( 'NONE', #91557, #86130 ) ;
#50682=EDGE_LOOP ( 'NONE', ( #97682, #2644, #18657, #108818, #42080 ) ) ;
#50685=CIRCLE ( 'NONE', #27679, 1.999999999999999556 ) ;
#50687=FACE_OUTER_BOUND ( 'NONE', #91326, .T. ) ;
#50710=EDGE_CURVE ( 'NONE', #53402, #65447, #101038, .T. ) ;
#50738=ORIENTED_EDGE ( 'NONE', *, *, #102468, .T. ) ;
#50743=CYLINDRICAL_SURFACE ( 'NONE', #10801, 2.000000000000003553 ) ;
#50751=ADVANCED_FACE ( 'NONE', ( #38261 ), #90312, .F. ) ;
#50753=EDGE_CURVE ( 'NONE', #53407, #48957, #10845, .T. ) ;
#50756=DIRECTION ( 'NONE',  ( 1.755985294532464991E-16, -1.000000000000000000, 1.338183447452830017E-16 ) ) ;
#50822=EDGE_CURVE ( 'NONE', #58393, #47709, #42131, .T. ) ;
#50826=DIRECTION ( 'NONE',  ( -1.295211781927295682E-16, 1.000000000000000000, 0.000000000000000000 ) ) ;
#50853=CIRCLE ( 'NONE', #27593, 1.999999999999998668 ) ;
#50922=EDGE_CURVE ( 'NONE', #70769, #1585, #100344, .T. ) ;
#50930=LINE ( 'NONE', #102413, #43302 ) ;
#50943=CARTESIAN_POINT ( 'NONE',  ( -16.36456115631862929, 1517.151704408390060, 220.0929384032941698 ) ) ;
#50976=AXIS2_PLACEMENT_3D ( 'NONE', #70773, #10262, #36575 ) ;
#50989=VERTEX_POINT ( 'NONE', #70677 ) ;
#51017=AXIS2_PLACEMENT_3D ( 'NONE', #81954, #99852, #49486 ) ;
#51056=EDGE_LOOP ( 'NONE', ( #69511, #33128, #16406, #30776, #43085 ) ) ;
#51060=AXIS2_PLACEMENT_3D ( 'NONE', #66216, #101968, #25254 ) ;
#51076=CARTESIAN_POINT ( 'NONE',  ( 12.39573405564623165, 1522.051704408389924, 218.5685989363918225 ) ) ;
#51089=DIRECTION ( 'NONE',  ( -0.9455185755993178454, 0.000000000000000000, 0.3255681544571539243 ) ) ;
#51133=AXIS2_PLACEMENT_3D ( 'NONE', #8763, #61976, #42944 ) ;
#51138=DIRECTION ( 'NONE',  ( -0.6736849260863837507, 0.000000000000000000, 0.7390186874254154326 ) ) ;
#51145=FACE_BOUND ( 'NONE', #87153, .T. ) ;
#51157=FACE_OUTER_BOUND ( 'NONE', #99246, .T. ) ;
#51232=ORIENTED_EDGE ( 'NONE', *, *, #45484, .T. ) ;
#51243=PRODUCT_DEFINITION_FORMATION_WITH_SPECIFIED_SOURCE ( 'ANY', '', #22290, .NOT_KNOWN. ) ;
#51253=ORIENTED_EDGE ( 'NONE', *, *, #29546, .F. ) ;
#51329=CARTESIAN_POINT ( 'NONE',  ( 15.69795926888880189, 1517.051704408389924, 222.7678737654429995 ) ) ;
#51345=PRODUCT_DEFINITION_CONTEXT ( 'detailed design', #14836, 'design' ) ;
#51350=DIRECTION ( 'NONE',  ( -0.6736849260863841948, 0.000000000000000000, 0.7390186874254148774 ) ) ;
#51362=LINE ( 'NONE', #12119, #25646 ) ;
#51374=EDGE_CURVE ( 'NONE', #75187, #69928, #43120, .T. ) ;
#51382=ORIENTED_EDGE ( 'NONE', *, *, #32431, .T. ) ;
#51388=CYLINDRICAL_SURFACE ( 'NONE', #17176, 2.000000000000003553 ) ;
#51402=ORIENTED_EDGE ( 'NONE', *, *, #66618, .T. ) ;
#51425=AXIS2_PLACEMENT_3D ( 'NONE', #67917, #33177, #109362 ) ;
#51443=EDGE_LOOP ( 'NONE', ( #31723, #70220 ) ) ;
#51451=ORIENTED_EDGE ( 'NONE', *, *, #52348, .T. ) ;
#51456=VERTEX_POINT ( 'NONE', #51919 ) ;
#51483=AXIS2_PLACEMENT_3D ( 'NONE', #62481, #10941, #105559 ) ;
#51537=CARTESIAN_POINT ( 'NONE',  ( 17.71193101166619854, 1519.551704408389924, 196.6727161458730109 ) ) ;
#51556=FACE_OUTER_BOUND ( 'NONE', #91673, .T. ) ;
#51566=CIRCLE ( 'NONE', #33632, 2.000000000000003553 ) ;
#51581=ORIENTED_EDGE ( 'NONE', *, *, #21692, .T. ) ;
#51594=CARTESIAN_POINT ( 'NONE',  ( -9.862951377749247683, 1519.551704408389924, 228.3939896778649654 ) ) ;
#51660=EDGE_CURVE ( 'NONE', #107071, #48164, #18162, .T. ) ;
#51690=CARTESIAN_POINT ( 'NONE',  ( 11.75869035672759999, 1519.551704408389924, 227.2994842695800060 ) ) ;
#51697=FACE_BOUND ( 'NONE', #63264, .T. ) ;
#51704=ORIENTED_EDGE ( 'NONE', *, *, #109148, .T. ) ;
#51742=CIRCLE ( 'NONE', #3468, 1.999999999999999556 ) ;
#51757=DIRECTION ( 'NONE',  ( -0.6736849260863839728, 0.000000000000000000, 0.7390186874254150995 ) ) ;
#51772=CARTESIAN_POINT ( 'NONE',  ( 3.272667022753707577, 1522.051704408389924, 229.2073556998901438 ) ) ;
#51776=CARTESIAN_POINT ( 'NONE',  ( -10.41132050640263174, 1522.051704408389924, 189.4661702785461728 ) ) ;
#51797=AXIS2_PLACEMENT_3D ( 'NONE', #13397, #5015, #6671 ) ;
#51819=EDGE_CURVE ( 'NONE', #79854, #53940, #78861, .T. ) ;
#51821=ORIENTED_EDGE ( 'NONE', *, *, #40774, .T. ) ;
#51828=CIRCLE ( 'NONE', #44726, 1.999999999999998668 ) ;
#51858=EDGE_LOOP ( 'NONE', ( #60971, #39718 ) ) ;
#51874=DIRECTION ( 'NONE',  ( 0.9455185755993178454, 0.000000000000000000, -0.3255681544571537578 ) ) ;
#51906=EDGE_LOOP ( 'NONE', ( #109338, #2172, #32597, #96357, #39658 ) ) ;
#51908=DIRECTION ( 'NONE',  ( -1.755985294532469921E-16, 1.000000000000000000, -1.338183447452831989E-16 ) ) ;
#51919=CARTESIAN_POINT ( 'NONE',  ( 16.36456115949343371, 1522.051704408389924, 198.1507535207238391 ) ) ;
#51932=DIRECTION ( 'NONE',  ( 5.980589973904019347E-17, -1.000000000000000000, 1.736889445713099699E-16 ) ) ;
#51982=FACE_OUTER_BOUND ( 'NONE', #55728, .T. ) ;
#51996=CIRCLE ( 'NONE', #3738, 1.999999999999999556 ) ;
#52021=LINE ( 'NONE', #2741, #746 ) ;
#52042=LINE ( 'NONE', #26826, #98149 ) ;
#52050=CIRCLE ( 'NONE', #77066, 1.999999999999999556 ) ;
#52058=CIRCLE ( 'NONE', #48470, 1.999999999999999556 ) ;
#52092=DIRECTION ( 'NONE',  ( -0.9455185755993178454, 0.000000000000000000, 0.3255681544571537578 ) ) ;
#52117=DIRECTION ( 'NONE',  ( -0.6736849260863841948, 0.000000000000000000, 0.7390186874254148774 ) ) ;
#52122=VERTEX_POINT ( 'NONE', #45482 ) ;
#52142=ORIENTED_EDGE ( 'NONE', *, *, #57877, .T. ) ;
#52146=VECTOR ( 'NONE', #65719, 1000.000000000000000 ) ;
#52199=CARTESIAN_POINT ( 'NONE',  ( 3.909710721586100224, 1517.051704408389924, 220.4764703678949900 ) ) ;
#52213=FACE_OUTER_BOUND ( 'NONE', #17965, .T. ) ;
#52242=EDGE_CURVE ( 'NONE', #75187, #105162, #96838, .T. ) ;
#52303=EDGE_CURVE ( 'NONE', #109826, #77569, #62830, .T. ) ;
#52319=DIRECTION ( 'NONE',  ( 1.755985294532469921E-16, -1.000000000000000000, 1.338183447452831989E-16 ) ) ;
#52348=EDGE_CURVE ( 'NONE', #36440, #18252, #100663, .T. ) ;
#52384=ORIENTED_EDGE ( 'NONE', *, *, #17773, .F. ) ;
#52416=ORIENTED_EDGE ( 'NONE', *, *, #110594, .F. ) ;
#52448=ORIENTED_EDGE ( 'NONE', *, *, #3914, .T. ) ;
#52468=CYLINDRICAL_SURFACE ( 'NONE', #64212, 2.000000000000003553 ) ;
#52470=DIRECTION ( 'NONE',  ( -0.6736849260863837507, 0.000000000000000000, 0.7390186874254154326 ) ) ;
#52473=DIRECTION ( 'NONE',  ( -5.980589973904019347E-17, 1.000000000000000000, -1.736889445713099699E-16 ) ) ;
#52491=CARTESIAN_POINT ( 'NONE',  ( 6.501609782144661231, 1517.151704408390060, 217.4228972380528262 ) ) ;
#52504=VERTEX_POINT ( 'NONE', #25604 ) ;
#52523=CYLINDRICAL_SURFACE ( 'NONE', #30090, 2.000000000000003553 ) ;
#52528=CARTESIAN_POINT ( 'NONE',  ( 11.81780673814840021, 1517.151704408390060, 195.5270144474869767 ) ) ;
#52556=EDGE_LOOP ( 'NONE', ( #17791, #69781 ) ) ;
#52624=CARTESIAN_POINT ( 'NONE',  ( 1.984413551915469975, 1517.151704408390060, 198.9129232538419956 ) ) ;
#52627=ORIENTED_EDGE ( 'NONE', *, *, #53214, .T. ) ;
#52672=ORIENTED_EDGE ( 'NONE', *, *, #48875, .T. ) ;
#52701=CYLINDRICAL_SURFACE ( 'NONE', #8223, 2.000000000000003109 ) ;
#52731=VERTEX_POINT ( 'NONE', #90904 ) ;
#52733=CARTESIAN_POINT ( 'NONE',  ( 19.66678637246580053, 1519.551704408389924, 202.3500283489900085 ) ) ;
#52784=DIRECTION ( 'NONE',  ( -1.755985294532469921E-16, 1.000000000000000000, -1.338183447452831989E-16 ) ) ;
#52788=ADVANCED_FACE ( 'NONE', ( #98200 ), #65723, .F. ) ;
#52789=EDGE_CURVE ( 'NONE', #14979, #64002, #95071, .T. ) ;
#52793=ADVANCED_FACE ( 'NONE', ( #57340 ), #98753, .F. ) ;
#52815=EDGE_LOOP ( 'NONE', ( #96801, #32294, #46378, #32266 ) ) ;
#52820=DIRECTION ( 'NONE',  ( 0.9858563016923833633, 0.000000000000000000, 0.1675928173085483863 ) ) ;
#52859=ORIENTED_EDGE ( 'NONE', *, *, #70047, .F. ) ;
#52918=CARTESIAN_POINT ( 'NONE',  ( -5.923682464646780943, 1517.051704408389924, 223.8623791742500089 ) ) ;
#52938=PLANE ( 'NONE',  #108806 ) ;
#52963=LINE ( 'NONE', #27740, #107248 ) ;
#52987=CARTESIAN_POINT ( 'NONE',  ( 1.925297169133120212, 1517.051704408389924, 230.6853930764029883 ) ) ;
#53004=ORIENTED_EDGE ( 'NONE', *, *, #80268, .T. ) ;
#53037=VERTEX_POINT ( 'NONE', #57558 ) ;
#53042=LINE ( 'NONE', #9912, #30348 ) ;
#53098=EDGE_CURVE ( 'NONE', #1490, #60256, #61138, .T. ) ;
#53099=CARTESIAN_POINT ( 'NONE',  ( 15.74021840907683512, 1517.051704408389924, 196.3375305114159062 ) ) ;
#53124=CIRCLE ( 'NONE', #46014, 2.000000000000002220 ) ;
#53152=ORIENTED_EDGE ( 'NONE', *, *, #75456, .T. ) ;
#53178=CARTESIAN_POINT ( 'NONE',  ( 21.62164173326539895, 1519.551704408389924, 208.0273405521070060 ) ) ;
#53187=ORIENTED_EDGE ( 'NONE', *, *, #94125, .F. ) ;
#53203=EDGE_LOOP ( 'NONE', ( #95379, #42300, #96185, #76965 ) ) ;
#53208=CARTESIAN_POINT ( 'NONE',  ( 17.04532911661896932, 1522.051704408389924, 221.2898363890541589 ) ) ;
#53214=EDGE_CURVE ( 'NONE', #22220, #8434, #53949, .T. ) ;
#53219=CARTESIAN_POINT ( 'NONE',  ( -9.225907677606096868, 1522.051704408389924, 219.6631043460218393 ) ) ;
#53240=CYLINDRICAL_SURFACE ( 'NONE', #108867, 2.000000000000003109 ) ;
#53259=CIRCLE ( 'NONE', #78253, 1.999999999999999556 ) ;
#53325=DIRECTION ( 'NONE',  ( 1.755985294532464991E-16, -1.000000000000000000, 1.338183447452830017E-16 ) ) ;
#53375=CARTESIAN_POINT ( 'NONE',  ( -11.75869035857540013, 1517.151704408390060, 190.9442076533970010 ) ) ;
#53402=VERTEX_POINT ( 'NONE', #26531 ) ;
#53407=VERTEX_POINT ( 'NONE', #60727 ) ;
#53421=AXIS2_PLACEMENT_3D ( 'NONE', #81975, #32140, #14779 ) ;
#53423=VECTOR ( 'NONE', #48693, 1000.000000000000000 ) ;
#53438=EDGE_CURVE ( 'NONE', #99771, #42647, #806, .T. ) ;
#53448=AXIS2_PLACEMENT_3D ( 'NONE', #25660, #69926, #110229 ) ;
#53483=EDGE_LOOP ( 'NONE', ( #79297, #105148 ) ) ;
#53546=DIRECTION ( 'NONE',  ( -1.755985294532469921E-16, 1.000000000000000000, -1.338183447452831989E-16 ) ) ;
#53555=EDGE_CURVE ( 'NONE', #62929, #28257, #42112, .T. ) ;
#53588=CARTESIAN_POINT ( 'NONE',  ( -21.01415622427472485, 1519.551704408389924, 217.3717009491090835 ) ) ;
#53628=CARTESIAN_POINT ( 'NONE',  ( -13.13561839920526886, 1517.051704408389924, 208.3084799397878157 ) ) ;
#53635=CARTESIAN_POINT ( 'NONE',  ( 1.925297169133120212, 1521.951704408389787, 230.6853930764029883 ) ) ;
#53747=AXIS2_PLACEMENT_3D ( 'NONE', #69353, #103463, #26770 ) ;
#53779=ORIENTED_EDGE ( 'NONE', *, *, #29523, .T. ) ;
#53794=CARTESIAN_POINT ( 'NONE',  ( 19.68364361584636768, 1521.951704408389787, 197.0079017806501156 ) ) ;
#53812=ORIENTED_EDGE ( 'NONE', *, *, #88500, .T. ) ;
#53816=VERTEX_POINT ( 'NONE', #50658 ) ;
#53854=AXIS2_PLACEMENT_3D ( 'NONE', #10642, #35281, #96296 ) ;
#53868=AXIS2_PLACEMENT_3D ( 'NONE', #35819, #8946, #26293 ) ;
#53911=CYLINDRICAL_SURFACE ( 'NONE', #31831, 2.000000000000003553 ) ;
#53926=DIRECTION ( 'NONE',  ( 0.9455185755993178454, 0.000000000000000000, -0.3255681544571537578 ) ) ;
#53933=CIRCLE ( 'NONE', #10976, 2.000000000000003553 ) ;
#53940=VERTEX_POINT ( 'NONE', #41700 ) ;
#53944=DIRECTION ( 'NONE',  ( 5.980589973904019347E-17, -1.000000000000000000, 1.736889445713099699E-16 ) ) ;
#53949=CIRCLE ( 'NONE', #78939, 2.000000000000003109 ) ;
#53987=DIRECTION ( 'NONE',  ( -0.6736849260863841948, 0.000000000000000000, 0.7390186874254148774 ) ) ;
#53995=FACE_OUTER_BOUND ( 'NONE', #11364, .T. ) ;
#53997=EDGE_CURVE ( 'NONE', #67084, #71877, #3893, .T. ) ;
#54002=CARTESIAN_POINT ( 'NONE',  ( -9.956645445956299412, 1517.051704408389924, 185.5808665542169820 ) ) ;
#54056=DIRECTION ( 'NONE',  ( -1.755985294532469921E-16, 1.000000000000000000, -1.338183447452831989E-16 ) ) ;
#54076=CARTESIAN_POINT ( 'NONE',  ( 2.621457251729789384, 1517.151704408390060, 190.1820379210428200 ) ) ;
#54085=ORIENTED_EDGE ( 'NONE', *, *, #90745, .T. ) ;
#54088=VERTEX_POINT ( 'NONE', #60743 ) ;
#54094=ORIENTED_EDGE ( 'NONE', *, *, #4812, .F. ) ;
#54105=DIRECTION ( 'NONE',  ( -5.980589973904019347E-17, 1.000000000000000000, -1.736889445713099699E-16 ) ) ;
#54126=DIRECTION ( 'NONE',  ( -1.755985294532469921E-16, 1.000000000000000000, -1.338183447452831989E-16 ) ) ;
#54132=CARTESIAN_POINT ( 'NONE',  ( 11.81780673814840021, 1522.051704408389924, 195.5270144474869767 ) ) ;
#54142=CARTESIAN_POINT ( 'NONE',  ( 11.15120484728000072, 1517.151704408390060, 220.1441346914401720 ) ) ;
#54171=ORIENTED_EDGE ( 'NONE', *, *, #93511, .T. ) ;
#54173=DIRECTION ( 'NONE',  ( 1.755985294532464991E-16, -1.000000000000000000, 1.338183447452830017E-16 ) ) ;
#54175=VERTEX_POINT ( 'NONE', #51772 ) ;
#54263=CARTESIAN_POINT ( 'NONE',  ( -1.984413551915469975, 1517.151704408390060, 219.3307686695569885 ) ) ;
#54269=EDGE_CURVE ( 'NONE', #101208, #46523, #95146, .T. ) ;
#54280=CARTESIAN_POINT ( 'NONE',  ( 17.71193101246160140, 1521.951704408389787, 196.6727161460330251 ) ) ;
#54283=FACE_OUTER_BOUND ( 'NONE', #60276, .T. ) ;
#54299=EDGE_CURVE ( 'NONE', #75258, #86231, #5718, .T. ) ;
#54320=ORIENTED_EDGE ( 'NONE', *, *, #60815, .T. ) ;
#54322=EDGE_CURVE ( 'NONE', #60349, #63956, #33704, .T. ) ;
#54348=CARTESIAN_POINT ( 'NONE',  ( -1.984413551915469975, 1522.051704408389924, 219.3307686695569885 ) ) ;
#54353=ORIENTED_EDGE ( 'NONE', *, *, #53438, .T. ) ;
#54407=DIRECTION ( 'NONE',  ( -0.9455185755993178454, 0.000000000000000000, 0.3255681544571539243 ) ) ;
#54475=CARTESIAN_POINT ( 'NONE',  ( 19.66678637211940028, 1517.051704408389924, 202.3500283489059939 ) ) ;
#54499=CARTESIAN_POINT ( 'NONE',  ( -4.517196230222687348, 1522.051704408389924, 190.6118719775071781 ) ) ;
#54504=ORIENTED_EDGE ( 'NONE', *, *, #70193, .F. ) ;
#54506=DIRECTION ( 'NONE',  ( 1.755985294532469921E-16, -1.000000000000000000, 1.338183447452831989E-16 ) ) ;
#54509=ORIENTED_EDGE ( 'NONE', *, *, #60980, .T. ) ;
#54588=VECTOR ( 'NONE', #97305, 1000.000000000000000 ) ;
#54600=LINE ( 'NONE', #107170, #27199 ) ;
#54625=CARTESIAN_POINT ( 'NONE',  ( -17.04532912216367180, 1519.551704408389924, 196.9538555332918293 ) ) ;
#54634=VERTEX_POINT ( 'NONE', #109204 ) ;
#54643=ADVANCED_FACE ( 'NONE', ( #41443 ), #98573, .F. ) ;
#54681=DIRECTION ( 'NONE',  ( -1.755985294532469921E-16, 1.000000000000000000, -1.338183447452831989E-16 ) ) ;
#54742=ORIENTED_EDGE ( 'NONE', *, *, #63095, .T. ) ;
#54748=CYLINDRICAL_SURFACE ( 'NONE', #103740, 2.000000000000003553 ) ;
#54773=ORIENTED_EDGE ( 'NONE', *, *, #51374, .T. ) ;
#54785=ORIENTED_EDGE ( 'NONE', *, *, #54299, .T. ) ;
#54791=CARTESIAN_POINT ( 'NONE',  ( -15.09047375999176843, 1522.051704408389924, 202.6311677367078232 ) ) ;
#54805=CARTESIAN_POINT ( 'NONE',  ( 15.12003195112066933, 1517.051704408389924, 199.7262892757531745 ) ) ;
#54807=EDGE_CURVE ( 'NONE', #4305, #22619, #14009, .T. ) ;
#54822=CIRCLE ( 'NONE', #6526, 1.999999999999998668 ) ;
#54823=DIRECTION ( 'NONE',  ( 5.980589973904019347E-17, -1.000000000000000000, 1.736889445713099699E-16 ) ) ;
#54834=CARTESIAN_POINT ( 'NONE',  ( -16.33500296837753041, 1522.051704408389924, 204.2067034917001536 ) ) ;
#54863=ORIENTED_EDGE ( 'NONE', *, *, #20930, .F. ) ;
#54891=DIRECTION ( 'NONE',  ( 0.9858563016923833633, 0.000000000000000000, 0.1675928173085483863 ) ) ;
#54896=DIRECTION ( 'NONE',  ( -5.980589973904019347E-17, 1.000000000000000000, -1.736889445713099699E-16 ) ) ;
#54897=VERTEX_POINT ( 'NONE', #4407 ) ;
#54949=EDGE_CURVE ( 'NONE', #43414, #41410, #107614, .T. ) ;
#54957=DIRECTION ( 'NONE',  ( 1.755985294532469921E-16, -1.000000000000000000, 1.338183447452831989E-16 ) ) ;
#55003=EDGE_LOOP ( 'NONE', ( #57532, #12221, #14275, #81119 ) ) ;
#55027=VERTEX_POINT ( 'NONE', #49717 ) ;
#55035=DIRECTION ( 'NONE',  ( 0.9455185755993178454, 0.000000000000000000, -0.3255681544571537578 ) ) ;
#55091=ORIENTED_EDGE ( 'NONE', *, *, #8283, .T. ) ;
#55151=CIRCLE ( 'NONE', #38958, 2.000000000000003553 ) ;
#55189=CARTESIAN_POINT ( 'NONE',  ( 0.02955819112566530210, 1522.051704408389924, 193.2356110507530218 ) ) ;
#55198=ORIENTED_EDGE ( 'NONE', *, *, #25421, .F. ) ;
#55222=DIRECTION ( 'NONE',  ( -0.6736849260863841948, 0.000000000000000000, 0.7390186874254148774 ) ) ;
#55262=AXIS2_PLACEMENT_3D ( 'NONE', #35227, #69414, #103525 ) ;
#55264=CARTESIAN_POINT ( 'NONE',  ( -8.486023334060126544, 1517.051704408389924, 211.0297173932031569 ) ) ;
#55304=ORIENTED_EDGE ( 'NONE', *, *, #25343, .F. ) ;
#55349=FACE_OUTER_BOUND ( 'NONE', #98963, .T. ) ;
#55374=CARTESIAN_POINT ( 'NONE',  ( 21.63849897547177292, 1521.951704408389787, 202.6852139837136804 ) ) ;
#55429=DIRECTION ( 'NONE',  ( -0.9455185755993178454, 0.000000000000000000, 0.3255681544571537578 ) ) ;
#55445=VERTEX_POINT ( 'NONE', #108089 ) ;
#55471=DIRECTION ( 'NONE',  ( -1.755985294532469921E-16, 1.000000000000000000, -1.338183447452831989E-16 ) ) ;
#55490=CARTESIAN_POINT ( 'NONE',  ( -5.257080573758882380, 1517.051704408389924, 199.2452589303538275 ) ) ;
#55506=AXIS2_PLACEMENT_3D ( 'NONE', #61340, #95460, #20932 ) ;
#55531=EDGE_CURVE ( 'NONE', #67122, #99156, #3970, .T. ) ;
#55535=CARTESIAN_POINT ( 'NONE',  ( -9.862951377749247683, 1519.551704408389924, 228.3939896778649654 ) ) ;
#55546=DIRECTION ( 'NONE',  ( -0.6736849260863841948, 0.000000000000000000, 0.7390186874254148774 ) ) ;
#55577=EDGE_LOOP ( 'NONE', ( #13158, #95397, #76100, #9259, #31230 ) ) ;
#55593=CARTESIAN_POINT ( 'NONE',  ( -17.68237282055029880, 1517.051704408389924, 205.6847408665509818 ) ) ;
#55598=ORIENTED_EDGE ( 'NONE', *, *, #75383, .F. ) ;
#55622=CARTESIAN_POINT ( 'NONE',  ( -6.871715297787709176, 1517.299312825780135, 183.7897170437481407 ) ) ;
#55636=DIRECTION ( 'NONE',  ( 0.9858563016923833633, 0.000000000000000000, 0.1675928173085483863 ) ) ;
#55643=EDGE_LOOP ( 'NONE', ( #70556, #27726, #109102, #619, #37117 ) ) ;
#55661=EDGE_CURVE ( 'NONE', #53402, #98048, #59436, .T. ) ;
#55728=EDGE_LOOP ( 'NONE', ( #9167, #64146, #15966, #17662 ) ) ;
#55775=VECTOR ( 'NONE', #50537, 1000.000000000000000 ) ;
#55789=VECTOR ( 'NONE', #73107, 1000.000000000000000 ) ;
#55806=LINE ( 'NONE', #46853, #8510 ) ;
#55822=ORIENTED_EDGE ( 'NONE', *, *, #40027, .T. ) ;
#55858=ORIENTED_EDGE ( 'NONE', *, *, #57013, .T. ) ;
#55884=EDGE_CURVE ( 'NONE', #24144, #79544, #88054, .T. ) ;
#55893=EDGE_LOOP ( 'NONE', ( #56698, #60508, #15852, #109078, #85311 ) ) ;
#55911=LINE ( 'NONE', #90029, #100060 ) ;
#55927=CARTESIAN_POINT ( 'NONE',  ( -15.69795926999090163, 1519.551704408389924, 195.4758181584410011 ) ) ;
#55987=ADVANCED_FACE ( 'NONE', ( #72199 ), #78367, .F. ) ;
#56003=ORIENTED_EDGE ( 'NONE', *, *, #98574, .F. ) ;
#56006=CARTESIAN_POINT ( 'NONE',  ( 19.63722818192610120, 1522.051704408389924, 218.2362632616380154 ) ) ;
#56011=ORIENTED_EDGE ( 'NONE', *, *, #104717, .F. ) ;
#56019=LINE ( 'NONE', #89055, #97799 ) ;
#56039=CARTESIAN_POINT ( 'NONE',  ( 1.376928043298436322, 1517.151704408390060, 191.7575736759021936 ) ) ;
#56047=DIRECTION ( 'NONE',  ( 1.755985294532469921E-16, -1.000000000000000000, 1.338183447452831989E-16 ) ) ;
#56079=DIRECTION ( 'NONE',  ( -0.9455185755993177343, 0.000000000000000000, 0.3255681544571540909 ) ) ;
#56110=VERTEX_POINT ( 'NONE', #36356 ) ;
#56135=CARTESIAN_POINT ( 'NONE',  ( 15.72751745975079984, 1517.151704408390060, 206.8816388537309763 ) ) ;
#56141=EDGE_LOOP ( 'NONE', ( #36971, #68718, #27, #43871 ) ) ;
#56150=VECTOR ( 'NONE', #39604, 1000.000000000000000 ) ;
#56210=DIRECTION ( 'NONE',  ( -1.755985294532469921E-16, 1.000000000000000000, -1.338183447452831989E-16 ) ) ;
#56226=CARTESIAN_POINT ( 'NONE',  ( 10.47043688597563005, 1517.151704408390060, 197.0050518223378333 ) ) ;
#56242=CARTESIAN_POINT ( 'NONE',  ( 0.04641543339558022729, 1519.551704408389924, 187.8934844797931305 ) ) ;
#56251=FILL_AREA_STYLE ('',( #23179 ) ) ;
#56291=VECTOR ( 'NONE', #88283, 1000.000000000000000 ) ;
#56337=CARTESIAN_POINT ( 'NONE',  ( 10.41132050455482982, 1517.151704408390060, 228.7775216444308342 ) ) ;
#56349=EDGE_CURVE ( 'NONE', #52504, #16564, #101839, .T. ) ;
#56380=DIRECTION ( 'NONE',  ( 0.9858563016923833633, 0.000000000000000000, 0.1675928173085483863 ) ) ;
#56411=AXIS2_PLACEMENT_3D ( 'NONE', #17102, #67023, #24425 ) ;
#56413=CARTESIAN_POINT ( 'NONE',  ( -17.66551557828621455, 1519.551704408389924, 200.3426142980228519 ) ) ;
#56434=ORIENTED_EDGE ( 'NONE', *, *, #106265, .T. ) ;
#56445=DIRECTION ( 'NONE',  ( -0.6736849260863841948, 0.000000000000000000, 0.7390186874254148774 ) ) ;
#56452=AXIS2_PLACEMENT_3D ( 'NONE', #62006, #11028, #96126 ) ;
#56524=DIRECTION ( 'NONE',  ( -0.9455185755993177343, 0.000000000000000000, 0.3255681544571540909 ) ) ;
#56572=DIRECTION ( 'NONE',  ( 5.980589973904019347E-17, -1.000000000000000000, 1.736889445713099699E-16 ) ) ;
#56591=DIRECTION ( 'NONE',  ( -1.755985294532469921E-16, 1.000000000000000000, -1.338183447452831989E-16 ) ) ;
#56641=DIRECTION ( 'NONE',  ( -5.980589973904019347E-17, 1.000000000000000000, -1.736889445713099699E-16 ) ) ;
#56663=ORIENTED_EDGE ( 'NONE', *, *, #94287, .F. ) ;
#56664=ORIENTED_EDGE ( 'NONE', *, *, #6690, .T. ) ;
#56675=CARTESIAN_POINT ( 'NONE',  ( 16.33500296837753041, 1517.051704408389924, 214.0369884316988305 ) ) ;
#56681=ORIENTED_EDGE ( 'NONE', *, *, #63863, .F. ) ;
#56692=CARTESIAN_POINT ( 'NONE',  ( 7.509485228916700454E-15, 1517.551704408389924, 209.1218459616989946 ) ) ;
#56698=ORIENTED_EDGE ( 'NONE', *, *, #31621, .F. ) ;
#56701=EDGE_LOOP ( 'NONE', ( #107384, #91364 ) ) ;
#56729=DIRECTION ( 'NONE',  ( -0.6736849260863841948, 0.000000000000000000, 0.7390186874254148774 ) ) ;
#56732=DIRECTION ( 'NONE',  ( 1.755985294532464991E-16, -1.000000000000000000, 1.338183447452830017E-16 ) ) ;
#56754=DIRECTION ( 'NONE',  ( -0.6736849260149578855, 0.000000000000000000, 0.7390186874905266823 ) ) ;
#56788=FACE_BOUND ( 'NONE', #13584, .T. ) ;
#56816=AXIS2_PLACEMENT_3D ( 'NONE', #47387, #5372, #105646 ) ;
#56834=EDGE_CURVE ( 'NONE', #39961, #54634, #81944, .T. ) ;
#56845=AXIS2_PLACEMENT_3D ( 'NONE', #33782, #25369, #36013 ) ;
#56906=ORIENTED_EDGE ( 'NONE', *, *, #38752, .T. ) ;
#56917=DIRECTION ( 'NONE',  ( 0.9455185755993178454, 0.000000000000000000, -0.3255681544571537578 ) ) ;
#56930=VERTEX_POINT ( 'NONE', #61208 ) ;
#56947=ORIENTED_EDGE ( 'NONE', *, *, #59577, .T. ) ;
#56954=CIRCLE ( 'NONE', #10498, 2.000000000000003553 ) ;
#56963=ADVANCED_FACE ( 'NONE', ( #15012 ), #73298, .F. ) ;
#56998=CARTESIAN_POINT ( 'NONE',  ( 22.96901158543817090, 1517.151704408390060, 206.5493031772561778 ) ) ;
#57009=EDGE_LOOP ( 'NONE', ( #65070, #2520, #62910, #71488, #104468 ) ) ;
#57013=EDGE_CURVE ( 'NONE', #30027, #72223, #66169, .T. ) ;
#57025=FACE_OUTER_BOUND ( 'NONE', #110513, .T. ) ;
#57034=AXIS2_PLACEMENT_3D ( 'NONE', #56135, #9851, #106538 ) ;
#57075=AXIS2_PLACEMENT_3D ( 'NONE', #99481, #5995, #40147 ) ;
#57092=ORIENTED_EDGE ( 'NONE', *, *, #40027, .F. ) ;
#57114=AXIS2_PLACEMENT_3D ( 'NONE', #17178, #44090, #50826 ) ;
#57134=ADVANCED_FACE ( 'NONE', ( #88314 ), #11607, .F. ) ;
#57143=EDGE_CURVE ( 'NONE', #104582, #65829, #18873, .T. ) ;
#57177=CARTESIAN_POINT ( 'NONE',  ( 19.66678637246580053, 1517.151704408390060, 202.3500283489900085 ) ) ;
#57218=DIRECTION ( 'NONE',  ( 5.980589973904019347E-17, -1.000000000000000000, 1.736889445713099699E-16 ) ) ;
#57231=EDGE_LOOP ( 'NONE', ( #73351, #69671, #69116, #72797 ) ) ;
#57233=ORIENTED_EDGE ( 'NONE', *, *, #50557, .F. ) ;
#57265=CARTESIAN_POINT ( 'NONE',  ( 17.71193101246160140, 1517.051704408389924, 196.6727161460330251 ) ) ;
#57277=CARTESIAN_POINT ( 'NONE',  ( -15.12003195112066933, 1522.051704408389924, 218.5174026476448432 ) ) ;
#57306=DIRECTION ( 'NONE',  ( 1.755985294532469921E-16, -1.000000000000000000, 1.338183447452831989E-16 ) ) ;
#57308=DIRECTION ( 'NONE',  ( -1.755985294532469921E-16, 1.000000000000000000, -1.338183447452831989E-16 ) ) ;
#57326=DIRECTION ( 'NONE',  ( 1.755985294532469921E-16, -1.000000000000000000, 1.338183447452831989E-16 ) ) ;
#57331=DIRECTION ( 'NONE',  ( -5.980589973904019347E-17, 1.000000000000000000, -1.736889445713099699E-16 ) ) ;
#57340=FACE_OUTER_BOUND ( 'NONE', #105196, .T. ) ;
#57357=AXIS2_PLACEMENT_3D ( 'NONE', #103584, #17903, #27425 ) ;
#57376=VECTOR ( 'NONE', #42678, 1000.000000000000000 ) ;
#57380=SURFACE_STYLE_FILL_AREA ( #56251 ) ;
#57430=CIRCLE ( 'NONE', #19826, 1.999999999999999556 ) ;
#57450=DIRECTION ( 'NONE',  ( -1.755985294532469921E-16, 1.000000000000000000, -1.338183447452831989E-16 ) ) ;
#57458=DIRECTION ( 'NONE',  ( -5.980589973904019347E-17, 1.000000000000000000, -1.736889445713099699E-16 ) ) ;
#57504=LINE ( 'NONE', #108433, #61013 ) ;
#57510=VERTEX_POINT ( 'NONE', #90360 ) ;
#57523=AXIS2_PLACEMENT_3D ( 'NONE', #70983, #48932, #21471 ) ;
#57532=ORIENTED_EDGE ( 'NONE', *, *, #33087, .F. ) ;
#57539=AXIS2_PLACEMENT_3D ( 'NONE', #7417, #57308, #16341 ) ;
#57555=DIRECTION ( 'NONE',  ( -5.980589973904019347E-17, 1.000000000000000000, -1.736889445713099699E-16 ) ) ;
#57558=CARTESIAN_POINT ( 'NONE',  ( -13.10606021074817029, 1522.051704408389924, 192.4222450282478292 ) ) ;
#57594=EDGE_CURVE ( 'NONE', #104584, #64002, #92031, .T. ) ;
#57619=FACE_OUTER_BOUND ( 'NONE', #78087, .T. ) ;
#57630=CIRCLE ( 'NONE', #9328, 2.000000000000003553 ) ;
#57633=DIRECTION ( 'NONE',  ( -1.755985294532469921E-16, 1.000000000000000000, -1.338183447452831989E-16 ) ) ;
#57670=CARTESIAN_POINT ( 'NONE',  ( -10.10023367162169983, 1517.051704408389924, 185.1638560673330005 ) ) ;
#57672=ADVANCED_FACE ( 'NONE', ( #109941 ), #33219, .F. ) ;
#57711=DIRECTION ( 'NONE',  ( -0.6736849260863841948, 0.000000000000000000, 0.7390186874254148774 ) ) ;
#57713=CARTESIAN_POINT ( 'NONE',  ( -16.33500296837753041, 1517.051704408389924, 204.2067034917001536 ) ) ;
#57742=DIRECTION ( 'NONE',  ( -5.980589973904019347E-17, 1.000000000000000000, -1.736889445713099699E-16 ) ) ;
#57793=EDGE_LOOP ( 'NONE', ( #1827, #35476 ) ) ;
#57820=DIRECTION ( 'NONE',  ( 1.755985294532469921E-16, -1.000000000000000000, 1.338183447452831989E-16 ) ) ;
#57828=DIRECTION ( 'NONE',  ( 5.980589973904019347E-17, -1.000000000000000000, 1.736889445713099699E-16 ) ) ;
#57846=CARTESIAN_POINT ( 'NONE',  ( 3.897009772517886272, 1521.951704408389787, 231.0205787110200788 ) ) ;
#57862=EDGE_CURVE ( 'NONE', #22264, #85592, #105557, .T. ) ;
#57877=EDGE_CURVE ( 'NONE', #10824, #53407, #6097, .T. ) ;
#57892=CARTESIAN_POINT ( 'NONE',  ( -14.38014760757803145, 1517.051704408389924, 209.8840156948171511 ) ) ;
#57905=ORIENTED_EDGE ( 'NONE', *, *, #82339, .T. ) ;
#57970=CARTESIAN_POINT ( 'NONE',  ( -10.44087869485973030, 1517.151704408390060, 205.3524051900861593 ) ) ;
#57972=CIRCLE ( 'NONE', #32920, 1.999999999999999556 ) ;
#57993=EDGE_CURVE ( 'NONE', #52122, #81601, #42962, .T. ) ;
#58017=ORIENTED_EDGE ( 'NONE', *, *, #39405, .F. ) ;
#58024=CARTESIAN_POINT ( 'NONE',  ( -15.09047375999176843, 1517.051704408389924, 202.6311677367078232 ) ) ;
#58032=FACE_OUTER_BOUND ( 'NONE', #29093, .T. ) ;
#58050=CYLINDRICAL_SURFACE ( 'NONE', #9089, 2.000000000000003553 ) ;
#58053=VERTEX_POINT ( 'NONE', #103191 ) ;
#58073=ORIENTED_EDGE ( 'NONE', *, *, #40540, .F. ) ;
#58085=VECTOR ( 'NONE', #2475, 1000.000000000000000 ) ;
#58097=CARTESIAN_POINT ( 'NONE',  ( 18.28985832975333636, 1522.051704408389924, 219.7143006364888436 ) ) ;
#58106=EDGE_LOOP ( 'NONE', ( #91584, #57905, #31763, #29209, #71181 ) ) ;
#58125=CIRCLE ( 'NONE', #92082, 1.999999999999999556 ) ;
#58130=VECTOR ( 'NONE', #108637, 1000.000000000000000 ) ;
#58141=ORIENTED_EDGE ( 'NONE', *, *, #85108, .F. ) ;
#58179=CARTESIAN_POINT ( 'NONE',  ( 17.66967187227356817, 1521.951704408389787, 223.1030594000600900 ) ) ;
#58197=ORIENTED_EDGE ( 'NONE', *, *, #37214, .F. ) ;
#58210=ADVANCED_FACE ( 'NONE', ( #58444, #56788, #38860, #65746, #107732, #14211, #108832, #47831, #64655, #81964, #73038, #107177, #30469, #39425, #31017, #48397, #5836, #39976, #74152, #101511, #18069, #9676, #51145, #92572, #51697, #17500, #24797, #59549, #69625, #59002, #76339, #86388, #84723, #210, #109944, #102610, #93130, #50592, #7475, #41637, #33769, #84177, #85270, #25356, #77450, #8021, #75792, #35438, #25910, #33222 ), #42740, .F. ) ;
#58215=CARTESIAN_POINT ( 'NONE',  ( -21.63849897585056681, 1521.951704408389787, 215.5584779397909188 ) ) ;
#58216=EDGE_CURVE ( 'NONE', #65907, #87972, #64394, .T. ) ;
#58299=CARTESIAN_POINT ( 'NONE',  ( 9.862951377130659836, 1517.051704408389924, 189.8497022437369708 ) ) ;
#58309=VERTEX_POINT ( 'NONE', #66180 ) ;
#58355=EDGE_LOOP ( 'NONE', ( #8682, #68757 ) ) ;
#58366=ADVANCED_FACE ( 'NONE', ( #51556 ), #25774, .F. ) ;
#58368=CARTESIAN_POINT ( 'NONE',  ( 1.925297170580940076, 1517.151704408390060, 230.6853930747409720 ) ) ;
#58393=VERTEX_POINT ( 'NONE', #1167 ) ;
#58409=CIRCLE ( 'NONE', #78064, 1.999999999999998668 ) ;
#58444=FACE_BOUND ( 'NONE', #19227, .T. ) ;
#58460=EDGE_CURVE ( 'NONE', #70320, #44418, #70589, .T. ) ;
#58517=EDGE_CURVE ( 'NONE', #102115, #104584, #80535, .T. ) ;
#58561=CARTESIAN_POINT ( 'NONE',  ( 11.15120484727999894, 1517.051704408389924, 220.1441346914401720 ) ) ;
#58582=DIRECTION ( 'NONE',  ( -0.6736849260863841948, 0.000000000000000000, 0.7390186874254148774 ) ) ;
#58599=CARTESIAN_POINT ( 'NONE',  ( -13.77266209894789917, 1517.151704408390060, 217.0393652727940150 ) ) ;
#58600=ORIENTED_EDGE ( 'NONE', *, *, #94710, .T. ) ;
#58619=DIRECTION ( 'NONE',  ( 1.755985294532469921E-16, -1.000000000000000000, 1.338183447452831989E-16 ) ) ;
#58623=DIRECTION ( 'NONE',  ( 0.9455185755993178454, 0.000000000000000000, -0.3255681544571537578 ) ) ;
#58634=ORIENTED_EDGE ( 'NONE', *, *, #17238, .T. ) ;
#58638=VERTEX_POINT ( 'NONE', #106642 ) ;
#58646=DIRECTION ( 'NONE',  ( -1.295211781927295682E-16, 1.000000000000000000, 0.000000000000000000 ) ) ;
#58647=VECTOR ( 'NONE', #103986, 1000.000000000000000 ) ;
#58672=CARTESIAN_POINT ( 'NONE',  ( 9.225907677606098645, 1522.051704408389924, 198.5805875773771731 ) ) ;
#58676=CARTESIAN_POINT ( 'NONE',  ( 7.891238773745893553, 1517.051704408389924, 189.5145166091198803 ) ) ;
#58698=CARTESIAN_POINT ( 'NONE',  ( -15.69795926856320101, 1517.051704408389924, 195.4758181589010064 ) ) ;
#58747=CARTESIAN_POINT ( 'NONE',  ( -6.647330431358690284, 1522.051704408389924, 184.4413780136169976 ) ) ;
#58780=CARTESIAN_POINT ( 'NONE',  ( -19.66678637224480397, 1522.051704408389924, 215.8936635741279986 ) ) ;
#58783=CARTESIAN_POINT ( 'NONE',  ( -19.63722818156799832, 1517.151704408390060, 200.0074286628000095 ) ) ;
#58815=CARTESIAN_POINT ( 'NONE',  ( -16.36456115631863284, 1522.051704408389924, 220.0929384032941698 ) ) ;
#58826=CIRCLE ( 'NONE', #44391, 1.999999999999999556 ) ;
#58879=ORIENTED_EDGE ( 'NONE', *, *, #25456, .T. ) ;
#58880=CARTESIAN_POINT ( 'NONE',  ( -17.66967187341156986, 1519.551704408389924, 195.1406325240351123 ) ) ;
#58889=CIRCLE ( 'NONE', #108921, 1.999999999999998668 ) ;
#58956=DIRECTION ( 'NONE',  ( 5.980589973904019347E-17, -1.000000000000000000, 1.736889445713099699E-16 ) ) ;
#58984=EDGE_CURVE ( 'NONE', #40567, #66989, #75786, .T. ) ;
#58999=DIRECTION ( 'NONE',  ( -1.755985294532469921E-16, 1.000000000000000000, -1.338183447452831989E-16 ) ) ;
#59002=FACE_BOUND ( 'NONE', #67145, .T. ) ;
#59004=CIRCLE ( 'NONE', #85840, 1.999999999999998668 ) ;
#59011=VERTEX_POINT ( 'NONE', #105430 ) ;
#59023=CARTESIAN_POINT ( 'NONE',  ( 6.531167973260561865, 1522.051704408389924, 201.5366623270788295 ) ) ;
#59054=DIRECTION ( 'NONE',  ( 1.755985294532464991E-16, -1.000000000000000000, 1.338183447452830017E-16 ) ) ;
#59069=ORIENTED_EDGE ( 'NONE', *, *, #66582, .T. ) ;
#59077=AXIS2_PLACEMENT_3D ( 'NONE', #35745, #110234, #59858 ) ;
#59102=DIRECTION ( 'NONE',  ( -1.755985294532469921E-16, 1.000000000000000000, -1.338183447452831989E-16 ) ) ;
#59189=AXIS2_PLACEMENT_3D ( 'NONE', #73989, #30863, #55546 ) ;
#59239=DIRECTION ( 'NONE',  ( -0.6736849260863841948, 0.000000000000000000, 0.7390186874254148774 ) ) ;
#59288=CIRCLE ( 'NONE', #19927, 2.000000000000003553 ) ;
#59303=ORIENTED_EDGE ( 'NONE', *, *, #91812, .T. ) ;
#59330=ORIENTED_EDGE ( 'NONE', *, *, #61302, .F. ) ;
#59348=AXIS2_PLACEMENT_3D ( 'NONE', #24515, #15557, #103868 ) ;
#59428=EDGE_LOOP ( 'NONE', ( #38282, #54085 ) ) ;
#59436=CIRCLE ( 'NONE', #11157, 1.999999999999999556 ) ;
#59445=LINE ( 'NONE', #8450, #79466 ) ;
#59483=CARTESIAN_POINT ( 'NONE',  ( -6.531167973260561865, 1517.051704408389924, 216.7070295963201829 ) ) ;
#59519=DIRECTION ( 'NONE',  ( -1.755985294532469921E-16, 1.000000000000000000, -1.338183447452831989E-16 ) ) ;
#59534=DIRECTION ( 'NONE',  ( -0.6736849260863839728, 0.000000000000000000, 0.7390186874254150995 ) ) ;
#59549=FACE_BOUND ( 'NONE', #107901, .T. ) ;
#59551=CARTESIAN_POINT ( 'NONE',  ( 2.621457251729789384, 1519.551704408389924, 190.1820379210428200 ) ) ;
#59576=ORIENTED_EDGE ( 'NONE', *, *, #2384, .T. ) ;
#59577=EDGE_CURVE ( 'NONE', #34885, #81601, #94524, .T. ) ;
#59586=ORIENTED_EDGE ( 'NONE', *, *, #62735, .T. ) ;
#59607=EDGE_CURVE ( 'NONE', #23415, #42647, #91832, .T. ) ;
#59626=CARTESIAN_POINT ( 'NONE',  ( -3.909710721586109550, 1522.051704408389924, 197.7672215555029993 ) ) ;
#59645=ADVANCED_FACE ( 'NONE', ( #9432 ), #31092, .T. ) ;
#59648=CARTESIAN_POINT ( 'NONE',  ( -7.848979634317430509, 1517.051704408389924, 202.2988320601959913 ) ) ;
#59650=EDGE_CURVE ( 'NONE', #30342, #51456, #68816, .T. ) ;
#59666=CARTESIAN_POINT ( 'NONE',  ( 3.968827103902559550, 1517.151704408390060, 188.7040005461919918 ) ) ;
#59680=FACE_BOUND ( 'NONE', #46232, .T. ) ;
#59705=ORIENTED_EDGE ( 'NONE', *, *, #80351, .T. ) ;
#59709=EDGE_CURVE ( 'NONE', #20461, #63893, #79391, .T. ) ;
#59713=ORIENTED_EDGE ( 'NONE', *, *, #92251, .F. ) ;
#59732=AXIS2_PLACEMENT_3D ( 'NONE', #73519, #57820, #41557 ) ;
#59762=VERTEX_POINT ( 'NONE', #105154 ) ;
#59765=CARTESIAN_POINT ( 'NONE',  ( 5.316196956075327051, 1519.551704408389924, 187.2259631713411636 ) ) ;
#59780=EDGE_CURVE ( 'NONE', #66581, #9033, #74327, .T. ) ;
#59806=CIRCLE ( 'NONE', #13253, 26.50000000000001421 ) ;
#59811=DIRECTION ( 'NONE',  ( -0.9455185755993178454, 0.000000000000000000, 0.3255681544571537578 ) ) ;
#59848=AXIS2_PLACEMENT_3D ( 'NONE', #23080, #30394, #72967 ) ;
#59854=CARTESIAN_POINT ( 'NONE',  ( 16.36456115949343015, 1517.151704408390060, 198.1507535207238391 ) ) ;
#59858=DIRECTION ( 'NONE',  ( -0.9455185755993178454, 0.000000000000000000, 0.3255681544571537578 ) ) ;
#59888=AXIS2_PLACEMENT_3D ( 'NONE', #33416, #25014, #110692 ) ;
#59893=EDGE_CURVE ( 'NONE', #34577, #97374, #43581, .T. ) ;
#59897=ORIENTED_EDGE ( 'NONE', *, *, #6266, .F. ) ;
#59927=CIRCLE ( 'NONE', #67043, 26.00000000000000711 ) ;
#60021=AXIS2_PLACEMENT_3D ( 'NONE', #88501, #29136, #81180 ) ;
#60037=EDGE_CURVE ( 'NONE', #63956, #14535, #68686, .T. ) ;
#60086=DIRECTION ( 'NONE',  ( -0.6736849260863841948, 0.000000000000000000, 0.7390186874254148774 ) ) ;
#60087=DIRECTION ( 'NONE',  ( 1.755985294532464991E-16, -1.000000000000000000, 1.338183447452830017E-16 ) ) ;
#60135=ORIENTED_EDGE ( 'NONE', *, *, #38481, .T. ) ;
#60193=DIRECTION ( 'NONE',  ( 1.755985294532469921E-16, -1.000000000000000000, 1.338183447452831989E-16 ) ) ;
#60199=DIRECTION ( 'NONE',  ( 0.9455185755993178454, 0.000000000000000000, -0.3255681544571539243 ) ) ;
#60256=VERTEX_POINT ( 'NONE', #10927 ) ;
#60276=EDGE_LOOP ( 'NONE', ( #47182, #13646, #56681, #66447, #74952 ) ) ;
#60283=AXIS2_PLACEMENT_3D ( 'NONE', #84015, #75090, #101339 ) ;
#60287=ORIENTED_EDGE ( 'NONE', *, *, #18490, .T. ) ;
#60319=CARTESIAN_POINT ( 'NONE',  ( -19.63722818156799832, 1519.551704408389924, 200.0074286628000095 ) ) ;
#60335=CARTESIAN_POINT ( 'NONE',  ( 9.833393186232889605, 1517.051704408389924, 205.7359371553449989 ) ) ;
#60349=VERTEX_POINT ( 'NONE', #79243 ) ;
#60356=CIRCLE ( 'NONE', #19155, 1.999999999999998668 ) ;
#60366=CIRCLE ( 'NONE', #12071, 1.999999999999999556 ) ;
#60370=EDGE_CURVE ( 'NONE', #83271, #56110, #59445, .T. ) ;
#60388=EDGE_CURVE ( 'NONE', #66989, #40567, #43651, .T. ) ;
#60406=CARTESIAN_POINT ( 'NONE',  ( -17.71193100849139768, 1522.051704408389924, 221.5709757781449980 ) ) ;
#60428=ORIENTED_EDGE ( 'NONE', *, *, #38974, .F. ) ;
#60452=EDGE_CURVE ( 'NONE', #47444, #61158, #16832, .T. ) ;
#60495=AXIS2_PLACEMENT_3D ( 'NONE', #34865, #69054, #1850 ) ;
#60508=ORIENTED_EDGE ( 'NONE', *, *, #42564, .F. ) ;
#60514=DIRECTION ( 'NONE',  ( -0.9455185755993177343, 0.000000000000000000, 0.3255681544571540909 ) ) ;
#60532=DIRECTION ( 'NONE',  ( 0.9455185755993167351, 0.000000000000000000, -0.3255681544571568109 ) ) ;
#60554=VERTEX_POINT ( 'NONE', #56413 ) ;
#60560=VECTOR ( 'NONE', #60952, 1000.000000000000000 ) ;
#60593=ORIENTED_EDGE ( 'NONE', *, *, #47425, .T. ) ;
#60633=DIRECTION ( 'NONE',  ( -0.9455185755993178454, 0.000000000000000000, 0.3255681544571537578 ) ) ;
#60684=AXIS2_PLACEMENT_3D ( 'NONE', #24782, #9659, #59534 ) ;
#60694=ORIENTED_EDGE ( 'NONE', *, *, #7436, .F. ) ;
#60698=VERTEX_POINT ( 'NONE', #26083 ) ;
#60705=AXIS2_PLACEMENT_3D ( 'NONE', #58780, #92918, #8352 ) ;
#60724=DIRECTION ( 'NONE',  ( 0.9455185755993178454, 0.000000000000000000, -0.3255681544571537578 ) ) ;
#60727=CARTESIAN_POINT ( 'NONE',  ( -5.316196955749758146, 1522.051704408389924, 231.0177287530028423 ) ) ;
#60740=VECTOR ( 'NONE', #79368, 1000.000000000000000 ) ;
#60743=CARTESIAN_POINT ( 'NONE',  ( 11.18076303840566155, 1522.051704408389924, 204.2578997804941707 ) ) ;
#60779=CIRCLE ( 'NONE', #17789, 1.999999999999999556 ) ;
#60806=ADVANCED_FACE ( 'NONE', ( #38775 ), #96629, .F. ) ;
#60815=EDGE_CURVE ( 'NONE', #60256, #88934, #19338, .T. ) ;
#60873=AXIS2_PLACEMENT_3D ( 'NONE', #22551, #57326, #56754 ) ;
#60888=AXIS2_PLACEMENT_3D ( 'NONE', #11835, #62840, #63911 ) ;
#60893=DIRECTION ( 'NONE',  ( 1.755985294532464991E-16, -1.000000000000000000, 1.338183447452830017E-16 ) ) ;
#60902=DIRECTION ( 'NONE',  ( -1.755985294532469921E-16, 1.000000000000000000, -1.338183447452830017E-16 ) ) ;
#60952=DIRECTION ( 'NONE',  ( -1.755985294532469921E-16, 1.000000000000000000, -1.338183447452831989E-16 ) ) ;
#60962=ORIENTED_EDGE ( 'NONE', *, *, #63226, .F. ) ;
#60971=ORIENTED_EDGE ( 'NONE', *, *, #8213, .T. ) ;
#60980=EDGE_CURVE ( 'NONE', #65868, #95431, #34686, .T. ) ;
#61013=VECTOR ( 'NONE', #92723, 1000.000000000000000 ) ;
#61024=DIRECTION ( 'NONE',  ( -0.6736849260863837507, 0.000000000000000000, 0.7390186874254154326 ) ) ;
#61025=EDGE_CURVE ( 'NONE', #64595, #4305, #2596, .T. ) ;
#61058=EDGE_CURVE ( 'NONE', #32612, #21086, #57972, .T. ) ;
#61094=( GEOMETRIC_REPRESENTATION_CONTEXT ( 3 ) GLOBAL_UNCERTAINTY_ASSIGNED_CONTEXT ( ( #44623 ) ) GLOBAL_UNIT_ASSIGNED_CONTEXT ( ( #45674, #105561, #62483 ) ) REPRESENTATION_CONTEXT ( 'NONE', 'WORKASPACE' ) );
#61138=CIRCLE ( 'NONE', #70003, 1.999999999999997780 ) ;
#61154=FACE_OUTER_BOUND ( 'NONE', #1134, .T. ) ;
#61158=VERTEX_POINT ( 'NONE', #24343 ) ;
#61163=DIRECTION ( 'NONE',  ( 5.980589973904019347E-17, -1.000000000000000000, 1.736889445713099699E-16 ) ) ;
#61208=CARTESIAN_POINT ( 'NONE',  ( -3.331783404088238143, 1517.051704408389924, 220.8088060444078451 ) ) ;
#61212=CYLINDRICAL_SURFACE ( 'NONE', #26685, 26.50000000000001421 ) ;
#61218=AXIS2_PLACEMENT_3D ( 'NONE', #66257, #57306, #56729 ) ;
#61234=PRESENTATION_STYLE_ASSIGNMENT (( #103746 ) ) ;
#61302=EDGE_CURVE ( 'NONE', #110436, #108856, #59806, .T. ) ;
#61306=EDGE_CURVE ( 'NONE', #87539, #104414, #6823, .T. ) ;
#61329=VERTEX_POINT ( 'NONE', #33129 ) ;
#61332=DIRECTION ( 'NONE',  ( -0.6736849260863839728, 0.000000000000000000, 0.7390186874254150995 ) ) ;
#61340=CARTESIAN_POINT ( 'NONE',  ( 3.909710721586100224, 1517.051704408389924, 220.4764703678949900 ) ) ;
#61501=AXIS2_PLACEMENT_3D ( 'NONE', #72152, #44171, #37419 ) ;
#61512=CYLINDRICAL_SURFACE ( 'NONE', #99734, 2.000000000000003553 ) ;
#61516=CARTESIAN_POINT ( 'NONE',  ( -14.35058941781813147, 1517.151704408390060, 193.9977807835901729 ) ) ;
#61632=CARTESIAN_POINT ( 'NONE',  ( -3.290427993577100100E-15, 1522.051704408389924, 209.1218459616989946 ) ) ;
#61639=EDGE_CURVE ( 'NONE', #3955, #23258, #33525, .T. ) ;
#61661=DIRECTION ( 'NONE',  ( 1.755985294532464991E-16, -1.000000000000000000, 1.338183447452830017E-16 ) ) ;
#61674=EDGE_LOOP ( 'NONE', ( #105570, #58634, #109549, #38884, #58073 ) ) ;
#61687=EDGE_CURVE ( 'NONE', #50393, #98226, #52021, .T. ) ;
#61700=AXIS2_PLACEMENT_3D ( 'NONE', #110096, #33371, #16011 ) ;
#61706=DIRECTION ( 'NONE',  ( 1.755985294532464991E-16, -1.000000000000000000, 1.338183447452830017E-16 ) ) ;
#61779=ORIENTED_EDGE ( 'NONE', *, *, #98012, .T. ) ;
#61806=ADVANCED_FACE ( 'NONE', ( #88918 ), #12204, .F. ) ;
#61817=ORIENTED_EDGE ( 'NONE', *, *, #8349, .F. ) ;
#61829=CARTESIAN_POINT ( 'NONE',  ( -11.75869035857540013, 1519.551704408389924, 190.9442076533970010 ) ) ;
#61906=FACE_BOUND ( 'NONE', #24290, .T. ) ;
#61941=AXIS2_PLACEMENT_3D ( 'NONE', #16452, #83686, #34395 ) ;
#61953=EDGE_LOOP ( 'NONE', ( #73261, #9966 ) ) ;
#61976=DIRECTION ( 'NONE',  ( 1.755985294532464991E-16, -1.000000000000000000, 1.338183447452830017E-16 ) ) ;
#61997=DIRECTION ( 'NONE',  ( -5.980589973904019347E-17, 1.000000000000000000, -1.736889445713099699E-16 ) ) ;
#62001=ORIENTED_EDGE ( 'NONE', *, *, #98919, .F. ) ;
#62006=CARTESIAN_POINT ( 'NONE',  ( -21.62164173379369814, 1519.551704408389924, 210.2163513719069954 ) ) ;
#62009=DIRECTION ( 'NONE',  ( 0.9858563016923833633, 0.000000000000000000, 0.1675928173085483863 ) ) ;
#62011=CIRCLE ( 'NONE', #67364, 1.999999999999999556 ) ;
#62018=ORIENTED_EDGE ( 'NONE', *, *, #78146, .F. ) ;
#62023=ORIENTED_EDGE ( 'NONE', *, *, #54807, .F. ) ;
#62033=CARTESIAN_POINT ( 'NONE',  ( -1.000362776118160035E-16, 1517.151704408390060, 209.1218459616989946 ) ) ;
#62058=ORIENTED_EDGE ( 'NONE', *, *, #107746, .F. ) ;
#62071=CARTESIAN_POINT ( 'NONE',  ( 19.63722818192610120, 1517.151704408390060, 218.2362632616380154 ) ) ;
#62143=CARTESIAN_POINT ( 'NONE',  ( -9.803834995107230554, 1517.051704408389924, 196.6215198571080123 ) ) ;
#62167=EDGE_LOOP ( 'NONE', ( #103862, #34727, #38507, #42805, #109640 ) ) ;
#62200=CYLINDRICAL_SURFACE ( 'NONE', #109097, 2.000000000000003553 ) ;
#62214=ORIENTED_EDGE ( 'NONE', *, *, #89073, .F. ) ;
#62290=EDGE_LOOP ( 'NONE', ( #15970, #43183, #102397, #84047, #43712 ) ) ;
#62326=DIRECTION ( 'NONE',  ( -0.9455185755993178454, 0.000000000000000000, 0.3255681544571537578 ) ) ;
#62329=COLOUR_RGB ( '', 0.31764706, 0.68627451, 0.89019608) ;
#62330=DIRECTION ( 'NONE',  ( -0.6736849260863841948, 0.000000000000000000, 0.7390186874254148774 ) ) ;
#62338=ORIENTED_EDGE ( 'NONE', *, *, #40540, .T. ) ;
#62398=ORIENTED_EDGE ( 'NONE', *, *, #9699, .T. ) ;
#62419=EDGE_CURVE ( 'NONE', #70558, #83569, #101027, .T. ) ;
#62473=CARTESIAN_POINT ( 'NONE',  ( -10.26338073471560008, 1521.551704408389924, 184.6900425920350131 ) ) ;
#62481=CARTESIAN_POINT ( 'NONE',  ( 9.862951377130659836, 1517.051704408389924, 189.8497022437369708 ) ) ;
#62483=( NAMED_UNIT ( * ) SI_UNIT ( $, .STERADIAN. ) SOLID_ANGLE_UNIT ( ) );
#62484=DIRECTION ( 'NONE',  ( -1.755985294532469921E-16, 1.000000000000000000, -1.338183447452831989E-16 ) ) ;
#62501=CYLINDRICAL_SURFACE ( 'NONE', #39307, 2.000000000000003553 ) ;
#62540=CARTESIAN_POINT ( 'NONE',  ( -10.02843955878900140, 1517.051704408389924, 185.3723613107750054 ) ) ;
#62551=EDGE_CURVE ( 'NONE', #63587, #77632, #47328, .T. ) ;
#62589=ORIENTED_EDGE ( 'NONE', *, *, #32431, .F. ) ;
#62612=CYLINDRICAL_SURFACE ( 'NONE', #74799, 2.000000000000003553 ) ;
#62613=ORIENTED_EDGE ( 'NONE', *, *, #69224, .F. ) ;
#62615=CARTESIAN_POINT ( 'NONE',  ( 1.997114501359403604, 1517.051704408389924, 188.3688149103338958 ) ) ;
#62621=AXIS2_PLACEMENT_3D ( 'NONE', #94244, #34354, #79136 ) ;
#62630=ORIENTED_EDGE ( 'NONE', *, *, #10758, .F. ) ;
#62635=CARTESIAN_POINT ( 'NONE',  ( -3.897009771321175986, 1521.951704408389787, 187.2231132109079113 ) ) ;
#62636=ORIENTED_EDGE ( 'NONE', *, *, #87021, .F. ) ;
#62685=DIRECTION ( 'NONE',  ( 1.755985294532469921E-16, -1.000000000000000000, 1.338183447452831989E-16 ) ) ;
#62701=DIRECTION ( 'NONE',  ( 5.980589973904019347E-17, -1.000000000000000000, 1.736889445713099699E-16 ) ) ;
#62735=EDGE_CURVE ( 'NONE', #8045, #22220, #24030, .T. ) ;
#62784=AXIS2_PLACEMENT_3D ( 'NONE', #3851, #38512, #30105 ) ;
#62788=VERTEX_POINT ( 'NONE', #103377 ) ;
#62814=CARTESIAN_POINT ( 'NONE',  ( -11.75869035456349998, 1521.951704408389787, 190.9442076542370046 ) ) ;
#62816=CIRCLE ( 'NONE', #28803, 2.000000000000003553 ) ;
#62830=CIRCLE ( 'NONE', #53868, 2.000000000000003109 ) ;
#62840=DIRECTION ( 'NONE',  ( 1.755985294532464991E-16, -1.000000000000000000, 1.338183447452830017E-16 ) ) ;
#62894=FACE_OUTER_BOUND ( 'NONE', #37859, .T. ) ;
#62900=DIRECTION ( 'NONE',  ( -5.980589973904019347E-17, 1.000000000000000000, -1.736889445713099699E-16 ) ) ;
#62910=ORIENTED_EDGE ( 'NONE', *, *, #51819, .T. ) ;
#62929=VERTEX_POINT ( 'NONE', #44440 ) ;
#62963=LINE ( 'NONE', #78613, #65875 ) ;
#62998=ORIENTED_EDGE ( 'NONE', *, *, #38623, .F. ) ;
#63007=DIRECTION ( 'NONE',  ( -0.9455185755993177343, 0.000000000000000000, 0.3255681544571540909 ) ) ;
#63011=AXIS2_PLACEMENT_3D ( 'NONE', #50063, #33236, #74166 ) ;
#63034=DIRECTION ( 'NONE',  ( 1.755985294532464991E-16, -1.000000000000000000, 1.338183447452830017E-16 ) ) ;
#63043=CARTESIAN_POINT ( 'NONE',  ( 19.02974267272307074, 1517.151704408390060, 211.0809136819971741 ) ) ;
#63053=DIRECTION ( 'NONE',  ( 0.9455185755993178454, 0.000000000000000000, -0.3255681544571537578 ) ) ;
#63071=ORIENTED_EDGE ( 'NONE', *, *, #62419, .T. ) ;
#63078=CIRCLE ( 'NONE', #80863, 2.000000000000003553 ) ;
#63095=EDGE_CURVE ( 'NONE', #31476, #56110, #18688, .T. ) ;
#63160=VERTEX_POINT ( 'NONE', #105292 ) ;
#63168=ADVANCED_FACE ( 'NONE', ( #29133 ), #72261, .F. ) ;
#63184=EDGE_CURVE ( 'NONE', #31573, #10167, #95681, .T. ) ;
#63192=CARTESIAN_POINT ( 'NONE',  ( -16.33500296837753041, 1517.151704408390060, 204.2067034917001536 ) ) ;
#63209=ORIENTED_EDGE ( 'NONE', *, *, #69383, .T. ) ;
#63212=ORIENTED_EDGE ( 'NONE', *, *, #54322, .T. ) ;
#63215=CARTESIAN_POINT ( 'NONE',  ( 19.66678637246580053, 1517.151704408390060, 202.3500283489900085 ) ) ;
#63218=DIRECTION ( 'NONE',  ( 1.755985294532469921E-16, -1.000000000000000000, 1.338183447452831989E-16 ) ) ;
#63226=EDGE_CURVE ( 'NONE', #36010, #104582, #58125, .T. ) ;
#63257=EDGE_LOOP ( 'NONE', ( #51232, #30150 ) ) ;
#63264=EDGE_LOOP ( 'NONE', ( #77691, #76777 ) ) ;
#63283=EDGE_CURVE ( 'NONE', #63956, #108856, #64409, .T. ) ;
#63306=EDGE_CURVE ( 'NONE', #36571, #43462, #63514, .T. ) ;
#63310=LINE ( 'NONE', #36417, #85745 ) ;
#63343=EDGE_CURVE ( 'NONE', #110436, #42621, #45510, .T. ) ;
#63344=DIRECTION ( 'NONE',  ( 5.980589973904019347E-17, -1.000000000000000000, 1.736889445713099699E-16 ) ) ;
#63346=CARTESIAN_POINT ( 'NONE',  ( 4.576312612474012553, 1522.051704408389924, 195.8593501239998318 ) ) ;
#63390=CARTESIAN_POINT ( 'NONE',  ( 1.984413551915469975, 1522.051704408389924, 198.9129232538419956 ) ) ;
#63415=FACE_OUTER_BOUND ( 'NONE', #92207, .T. ) ;
#63416=ORIENTED_EDGE ( 'NONE', *, *, #5486, .T. ) ;
#63418=DIRECTION ( 'NONE',  ( -1.755985294532469921E-16, 1.000000000000000000, -1.338183447452831989E-16 ) ) ;
#63446=DIRECTION ( 'NONE',  ( -1.755985294532469921E-16, 1.000000000000000000, -1.338183447452831989E-16 ) ) ;
#63489=DIRECTION ( 'NONE',  ( 1.755985294532464991E-16, -1.000000000000000000, 1.338183447452830017E-16 ) ) ;
#63491=DIRECTION ( 'NONE',  ( -0.9455185755993178454, 0.000000000000000000, 0.3255681544571537578 ) ) ;
#63514=CIRCLE ( 'NONE', #47413, 1.999999999999999556 ) ;
#63539=FACE_OUTER_BOUND ( 'NONE', #85184, .T. ) ;
#63550=ORIENTED_EDGE ( 'NONE', *, *, #29592, .T. ) ;
#63587=VERTEX_POINT ( 'NONE', #102929 ) ;
#63618=AXIS2_PLACEMENT_3D ( 'NONE', #54280, #54823, #22262 ) ;
#63621=VERTEX_POINT ( 'NONE', #45281 ) ;
#63628=VECTOR ( 'NONE', #30780, 1000.000000000000000 ) ;
#63691=DIRECTION ( 'NONE',  ( 0.9455185755993177343, 0.000000000000000000, -0.3255681544571540909 ) ) ;
#63702=DIRECTION ( 'NONE',  ( -1.744230429721540409E-14, -1.000000000000000000, -3.290755053036525162E-15 ) ) ;
#63755=ADVANCED_FACE ( 'NONE', ( #106800 ), #99491, .F. ) ;
#63756=CARTESIAN_POINT ( 'NONE',  ( -6.719124544191419801, 1522.051704408389924, 184.2328727701749926 ) ) ;
#63775=ORIENTED_EDGE ( 'NONE', *, *, #3777, .F. ) ;
#63838=DIRECTION ( 'NONE',  ( -5.980589973904019347E-17, 1.000000000000000000, -1.736889445713099699E-16 ) ) ;
#63841=ORIENTED_EDGE ( 'NONE', *, *, #54807, .T. ) ;
#63863=EDGE_CURVE ( 'NONE', #1004, #109826, #66861, .T. ) ;
#63893=VERTEX_POINT ( 'NONE', #65115 ) ;
#63896=AXIS2_PLACEMENT_3D ( 'NONE', #44112, #102334, #59811 ) ;
#63899=DIRECTION ( 'NONE',  ( -5.980589973904019347E-17, 1.000000000000000000, -1.736889445713099699E-16 ) ) ;
#63901=VERTEX_POINT ( 'NONE', #83536 ) ;
#63911=DIRECTION ( 'NONE',  ( 0.9455185755993178454, 0.000000000000000000, -0.3255681544571537578 ) ) ;
#63935=ORIENTED_EDGE ( 'NONE', *, *, #93928, .T. ) ;
#63951=CARTESIAN_POINT ( 'NONE',  ( -9.862951376772540968, 1517.051704408389924, 228.3939896807019920 ) ) ;
#63956=VERTEX_POINT ( 'NONE', #106953 ) ;
#63959=CARTESIAN_POINT ( 'NONE',  ( -19.02974267272306719, 1522.051704408389924, 207.1627782414018100 ) ) ;
#63961=FACE_OUTER_BOUND ( 'NONE', #57231, .T. ) ;
#63973=AXIS2_PLACEMENT_3D ( 'NONE', #41449, #17303, #108643 ) ;
#64002=VERTEX_POINT ( 'NONE', #24576 ) ;
#64013=CARTESIAN_POINT ( 'NONE',  ( -8.515581525576479294, 1519.551704408389924, 226.9159523030141372 ) ) ;
#64021=VERTEX_POINT ( 'NONE', #69397 ) ;
#64024=DIRECTION ( 'NONE',  ( 5.980589973904019347E-17, -1.000000000000000000, 1.736889445713099699E-16 ) ) ;
#64054=EDGE_LOOP ( 'NONE', ( #97825, #60428, #99628, #58879, #16581 ) ) ;
#64064=DIRECTION ( 'NONE',  ( -0.9455185755993178454, 0.000000000000000000, 0.3255681544571539243 ) ) ;
#64076=AXIS2_PLACEMENT_3D ( 'NONE', #21612, #98338, #80452 ) ;
#64116=ADVANCED_FACE ( 'NONE', ( #88379 ), #78319, .F. ) ;
#64146=ORIENTED_EDGE ( 'NONE', *, *, #34185, .F. ) ;
#64161=CYLINDRICAL_SURFACE ( 'NONE', #37436, 2.000000000000003109 ) ;
#64197=ORIENTED_EDGE ( 'NONE', *, *, #17197, .F. ) ;
#64212=AXIS2_PLACEMENT_3D ( 'NONE', #103378, #51908, #86048 ) ;
#64221=VERTEX_POINT ( 'NONE', #36867 ) ;
#64232=DIRECTION ( 'NONE',  ( 1.755985294532464991E-16, -1.000000000000000000, 1.338183447452830017E-16 ) ) ;
#64235=CARTESIAN_POINT ( 'NONE',  ( 7.878537825433329367, 1522.051704408389924, 200.0586249522280013 ) ) ;
#64258=ORIENTED_EDGE ( 'NONE', *, *, #3657, .F. ) ;
#64279=VERTEX_POINT ( 'NONE', #54791 ) ;
#64296=DIRECTION ( 'NONE',  ( -0.6736849260863841948, 0.000000000000000000, 0.7390186874254148774 ) ) ;
#64310=CARTESIAN_POINT ( 'NONE',  ( -21.62164173379369814, 1517.151704408390060, 210.2163513719069954 ) ) ;
#64328=DIRECTION ( 'NONE',  ( -1.755985294532469921E-16, 1.000000000000000000, -1.338183447452831989E-16 ) ) ;
#64343=AXIS2_PLACEMENT_3D ( 'NONE', #64767, #23265, #41733 ) ;
#64347=DIRECTION ( 'NONE',  ( -1.755985294532469921E-16, 1.000000000000000000, -1.338183447452831989E-16 ) ) ;
#64378=EDGE_CURVE ( 'NONE', #18252, #54175, #18538, .T. ) ;
#64381=CIRCLE ( 'NONE', #16056, 1.999999999999998668 ) ;
#64394=CIRCLE ( 'NONE', #30406, 1.999999999999998668 ) ;
#64409=LINE ( 'NONE', #82833, #33080 ) ;
#64422=AXIS2_PLACEMENT_3D ( 'NONE', #92448, #15722, #15186 ) ;
#64437=FACE_OUTER_BOUND ( 'NONE', #26925, .T. ) ;
#64466=DIRECTION ( 'NONE',  ( -1.755985294532469921E-16, 1.000000000000000000, -1.338183447452831989E-16 ) ) ;
#64481=CIRCLE ( 'NONE', #17999, 2.000000000000011102 ) ;
#64509=CARTESIAN_POINT ( 'NONE',  ( 5.864566082395450408, 1517.151704408390060, 226.1537825710409777 ) ) ;
#64546=VECTOR ( 'NONE', #10089, 1000.000000000000000 ) ;
#64576=FACE_OUTER_BOUND ( 'NONE', #69158, .T. ) ;
#64587=EDGE_CURVE ( 'NONE', #66446, #36071, #6086, .T. ) ;
#64593=CARTESIAN_POINT ( 'NONE',  ( 5.923682464646780943, 1522.051704408389924, 194.3813127491490036 ) ) ;
#64595=VERTEX_POINT ( 'NONE', #80217 ) ;
#64625=AXIS2_PLACEMENT_3D ( 'NONE', #32773, #66957, #42841 ) ;
#64637=AXIS2_PLACEMENT_3D ( 'NONE', #75859, #31637, #99935 ) ;
#64655=FACE_BOUND ( 'NONE', #51443, .T. ) ;
#64657=AXIS2_PLACEMENT_3D ( 'NONE', #11016, #61997, #12665 ) ;
#64691=ORIENTED_EDGE ( 'NONE', *, *, #107012, .T. ) ;
#64701=EDGE_CURVE ( 'NONE', #20783, #17997, #47189, .T. ) ;
#64742=ORIENTED_EDGE ( 'NONE', *, *, #3777, .T. ) ;
#64767=CARTESIAN_POINT ( 'NONE',  ( -13.77266209894789917, 1517.051704408389924, 217.0393652727940150 ) ) ;
#64808=CARTESIAN_POINT ( 'NONE',  ( 1.997114500746473675, 1519.551704408389924, 188.3688149102297018 ) ) ;
#64850=EDGE_LOOP ( 'NONE', ( #61779, #34536 ) ) ;
#64860=CARTESIAN_POINT ( 'NONE',  ( 0.5779273184081717973, 1522.051704408389924, 232.1634304495918002 ) ) ;
#64863=DIRECTION ( 'NONE',  ( -0.9455185755993177343, 0.000000000000000000, 0.3255681544571540909 ) ) ;
#64883=ORIENTED_EDGE ( 'NONE', *, *, #102468, .F. ) ;
#64918=ORIENTED_EDGE ( 'NONE', *, *, #107484, .F. ) ;
#64934=CARTESIAN_POINT ( 'NONE',  ( -3.968827103576990201, 1517.151704408390060, 229.5396913781519856 ) ) ;
#64955=VERTEX_POINT ( 'NONE', #33319 ) ;
#64960=VERTEX_POINT ( 'NONE', #32238 ) ;
#65038=DIRECTION ( 'NONE',  ( -0.6736849260863839728, 0.000000000000000000, 0.7390186874254150995 ) ) ;
#65070=ORIENTED_EDGE ( 'NONE', *, *, #34461, .F. ) ;
#65097=AXIS2_PLACEMENT_3D ( 'NONE', #107361, #13280, #72146 ) ;
#65099=DIRECTION ( 'NONE',  ( -0.9455185755993178454, 0.000000000000000000, 0.3255681544571537578 ) ) ;
#65114=CYLINDRICAL_SURFACE ( 'NONE', #34962, 1.999999999999999556 ) ;
#65115=CARTESIAN_POINT ( 'NONE',  ( -19.05930086066416607, 1522.051704408389924, 223.0490131529958262 ) ) ;
#65124=AXIS2_PLACEMENT_3D ( 'NONE', #91084, #6537, #47995 ) ;
#65159=CARTESIAN_POINT ( 'NONE',  ( 2.359533070475779804E-16, 1517.051704408389924, 209.1218459616989946 ) ) ;
#65192=EDGE_CURVE ( 'NONE', #59762, #98761, #103577, .T. ) ;
#65229=DIRECTION ( 'NONE',  ( 1.755985294532469921E-16, -1.000000000000000000, 1.338183447452831989E-16 ) ) ;
#65239=VERTEX_POINT ( 'NONE', #2807 ) ;
#65299=DIRECTION ( 'NONE',  ( -1.755985294532469921E-16, 1.000000000000000000, -1.338183447452831989E-16 ) ) ;
#65336=FACE_BOUND ( 'NONE', #100070, .T. ) ;
#65359=EDGE_CURVE ( 'NONE', #22619, #75633, #50853, .T. ) ;
#65382=ORIENTED_EDGE ( 'NONE', *, *, #93088, .F. ) ;
#65405=CARTESIAN_POINT ( 'NONE',  ( -19.68364361505096483, 1517.051704408389924, 221.2357901429078879 ) ) ;
#65447=VERTEX_POINT ( 'NONE', #50585 ) ;
#65455=EDGE_LOOP ( 'NONE', ( #54863, #14163, #89307, #2578, #2454 ) ) ;
#65471=ORIENTED_EDGE ( 'NONE', *, *, #22650, .T. ) ;
#65472=CARTESIAN_POINT ( 'NONE',  ( 15.09047375999176843, 1522.051704408389924, 215.6125241866901661 ) ) ;
#65489=VERTEX_POINT ( 'NONE', #57892 ) ;
#65506=ORIENTED_EDGE ( 'NONE', *, *, #88303, .F. ) ;
#65521=ORIENTED_EDGE ( 'NONE', *, *, #28902, .F. ) ;
#65523=CARTESIAN_POINT ( 'NONE',  ( 19.66678637246580053, 1519.551704408389924, 202.3500283489900085 ) ) ;
#65528=LINE ( 'NONE', #37554, #68130 ) ;
#65538=LINE ( 'NONE', #89061, #94034 ) ;
#65574=DIRECTION ( 'NONE',  ( 1.755985294532469921E-16, -1.000000000000000000, 1.338183447452831989E-16 ) ) ;
#65580=CARTESIAN_POINT ( 'NONE',  ( -13.13561839920527063, 1517.151704408390060, 208.3084799397878157 ) ) ;
#65641=VERTEX_POINT ( 'NONE', #109937 ) ;
#65654=ORIENTED_EDGE ( 'NONE', *, *, #85543, .F. ) ;
#65675=ORIENTED_EDGE ( 'NONE', *, *, #17108, .T. ) ;
#65719=DIRECTION ( 'NONE',  ( -1.755985294532469921E-16, 1.000000000000000000, -1.338183447452831989E-16 ) ) ;
#65723=CYLINDRICAL_SURFACE ( 'NONE', #48566, 2.000000000000002220 ) ;
#65746=FACE_BOUND ( 'NONE', #17004, .T. ) ;
#65754=ORIENTED_EDGE ( 'NONE', *, *, #50753, .T. ) ;
#65806=ADVANCED_FACE ( 'NONE', ( #99171 ), #37641, .F. ) ;
#65820=LINE ( 'NONE', #7548, #29446 ) ;
#65822=CARTESIAN_POINT ( 'NONE',  ( 17.71193101166619854, 1517.151704408390060, 196.6727161458730109 ) ) ;
#65829=VERTEX_POINT ( 'NONE', #46620 ) ;
#65853=DIRECTION ( 'NONE',  ( -1.755985294532469921E-16, 1.000000000000000000, -1.338183447452831989E-16 ) ) ;
#65864=ORIENTED_EDGE ( 'NONE', *, *, #60452, .T. ) ;
#65868=VERTEX_POINT ( 'NONE', #107043 ) ;
#65875=VECTOR ( 'NONE', #70251, 1000.000000000000000 ) ;
#65882=FACE_BOUND ( 'NONE', #15591, .T. ) ;
#65901=DIRECTION ( 'NONE',  ( -0.9455185755993178454, 0.000000000000000000, 0.3255681544571537578 ) ) ;
#65907=VERTEX_POINT ( 'NONE', #50463 ) ;
#65926=DIRECTION ( 'NONE',  ( 1.755985294532464991E-16, -1.000000000000000000, 1.338183447452830017E-16 ) ) ;
#65941=DIRECTION ( 'NONE',  ( 5.980589973904019347E-17, -1.000000000000000000, 1.736889445713099699E-16 ) ) ;
#66009=ORIENTED_EDGE ( 'NONE', *, *, #22780, .T. ) ;
#66045=VECTOR ( 'NONE', #104205, 1000.000000000000000 ) ;
#66063=VERTEX_POINT ( 'NONE', #59023 ) ;
#66068=DIRECTION ( 'NONE',  ( 0.9455185755993177343, 0.000000000000000000, -0.3255681544571540909 ) ) ;
#66070=DIRECTION ( 'NONE',  ( -0.9455185755993178454, 0.000000000000000000, 0.3255681544571537578 ) ) ;
#66105=ADVANCED_FACE ( 'NONE', ( #102852 ), #47657, .F. ) ;
#66134=ADVANCED_FACE ( 'NONE', ( #95030 ), #87182, .F. ) ;
#66148=DIRECTION ( 'NONE',  ( -0.6736849260863839728, 0.000000000000000000, 0.7390186874254150995 ) ) ;
#66169=CIRCLE ( 'NONE', #17741, 2.000000000000003553 ) ;
#66180=CARTESIAN_POINT ( 'NONE',  ( -6.954065720117950100, 1517.551704408389924, 183.5505540514350002 ) ) ;
#66211=DIRECTION ( 'NONE',  ( -0.9455185755993178454, 0.000000000000000000, 0.3255681544571537578 ) ) ;
#66216=CARTESIAN_POINT ( 'NONE',  ( 9.803834995107230554, 1517.051704408389924, 221.6221720662910002 ) ) ;
#66227=LINE ( 'NONE', #67869, #66045 ) ;
#66251=ORIENTED_EDGE ( 'NONE', *, *, #16504, .F. ) ;
#66257=CARTESIAN_POINT ( 'NONE',  ( -15.69795926999090163, 1519.551704408389924, 195.4758181584410011 ) ) ;
#66288=DIRECTION ( 'NONE',  ( 0.9455185755993178454, 0.000000000000000000, -0.3255681544571537578 ) ) ;
#66291=AXIS2_PLACEMENT_3D ( 'NONE', #93413, #16680, #8302 ) ;
#66292=DIRECTION ( 'NONE',  ( -0.6736849260863837507, 0.000000000000000000, 0.7390186874254154326 ) ) ;
#66299=DIRECTION ( 'NONE',  ( 0.9858563016923833633, 0.000000000000000000, 0.1675928173085483863 ) ) ;
#66341=ORIENTED_EDGE ( 'NONE', *, *, #89147, .T. ) ;
#66365=CIRCLE ( 'NONE', #62784, 2.000000000000003553 ) ;
#66372=CARTESIAN_POINT ( 'NONE',  ( -20.27427188162092975, 1517.151704408390060, 208.7383139970561672 ) ) ;
#66429=EDGE_LOOP ( 'NONE', ( #16301, #67012 ) ) ;
#66440=FACE_BOUND ( 'NONE', #30375, .T. ) ;
#66446=VERTEX_POINT ( 'NONE', #106846 ) ;
#66447=ORIENTED_EDGE ( 'NONE', *, *, #87716, .T. ) ;
#66455=VECTOR ( 'NONE', #104892, 1000.000000000000000 ) ;
#66462=CARTESIAN_POINT ( 'NONE',  ( -5.257080573758877939, 1522.051704408389924, 199.2452589303538275 ) ) ;
#66475=DIRECTION ( 'NONE',  ( -0.6736849260863839728, 0.000000000000000000, 0.7390186874254150995 ) ) ;
#66477=DIRECTION ( 'NONE',  ( -0.6736849260863841948, 0.000000000000000000, 0.7390186874254148774 ) ) ;
#66489=DIRECTION ( 'NONE',  ( -0.6736849260863841948, 0.000000000000000000, 0.7390186874254148774 ) ) ;
#66505=VERTEX_POINT ( 'NONE', #58676 ) ;
#66533=CARTESIAN_POINT ( 'NONE',  ( -1.984413551915469975, 1517.051704408389924, 219.3307686695569885 ) ) ;
#66536=DIRECTION ( 'NONE',  ( -1.755985294532469921E-16, 1.000000000000000000, -1.338183447452831989E-16 ) ) ;
#66569=CARTESIAN_POINT ( 'NONE',  ( -9.833393186232900263, 1517.151704408390060, 212.5077547680540135 ) ) ;
#66579=AXIS2_PLACEMENT_3D ( 'NONE', #35632, #46282, #87148 ) ;
#66581=VERTEX_POINT ( 'NONE', #44081 ) ;
#66582=EDGE_CURVE ( 'NONE', #51456, #48164, #50685, .T. ) ;
#66596=ADVANCED_FACE ( 'NONE', ( #17169 ), #110167, .F. ) ;
#66602=ORIENTED_EDGE ( 'NONE', *, *, #34965, .T. ) ;
#66609=DIRECTION ( 'NONE',  ( -5.980589973904019347E-17, 1.000000000000000000, -1.736889445713099699E-16 ) ) ;
#66618=EDGE_CURVE ( 'NONE', #36010, #33249, #51362, .T. ) ;
#66637=LINE ( 'NONE', #16715, #37413 ) ;
#66667=EDGE_CURVE ( 'NONE', #53940, #98249, #87747, .T. ) ;
#66762=DIRECTION ( 'NONE',  ( 1.755985294532469921E-16, -1.000000000000000000, 1.338183447452831989E-16 ) ) ;
#66771=ORIENTED_EDGE ( 'NONE', *, *, #9926, .T. ) ;
#66781=DIRECTION ( 'NONE',  ( 0.9455185755993178454, 0.000000000000000000, -0.3255681544571537578 ) ) ;
#66861=CIRCLE ( 'NONE', #59732, 2.000000000000003109 ) ;
#66914=DIRECTION ( 'NONE',  ( -1.755985294532469921E-16, 1.000000000000000000, -1.338183447452831989E-16 ) ) ;
#66930=AXIS2_PLACEMENT_3D ( 'NONE', #21946, #14115, #27214 ) ;
#66933=CARTESIAN_POINT ( 'NONE',  ( 0.3255681544566436103, 1492.051704408390151, 210.0673645372983174 ) ) ;
#66939=VECTOR ( 'NONE', #95185, 1000.000000000000000 ) ;
#66957=DIRECTION ( 'NONE',  ( 1.755985294532469921E-16, -1.000000000000000000, 1.338183447452831989E-16 ) ) ;
#66983=FACE_BOUND ( 'NONE', #50349, .T. ) ;
#66989=VERTEX_POINT ( 'NONE', #310 ) ;
#66999=ADVANCED_FACE ( 'NONE', ( #50687 ), #41732, .F. ) ;
#67011=ORIENTED_EDGE ( 'NONE', *, *, #49019, .T. ) ;
#67012=ORIENTED_EDGE ( 'NONE', *, *, #70047, .T. ) ;
#67017=DIRECTION ( 'NONE',  ( 1.755985294532464991E-16, -1.000000000000000000, 1.338183447452830017E-16 ) ) ;
#67022=ORIENTED_EDGE ( 'NONE', *, *, #97884, .F. ) ;
#67023=DIRECTION ( 'NONE',  ( -1.755985294532469921E-16, 1.000000000000000000, -1.338183447452831989E-16 ) ) ;
#67043=AXIS2_PLACEMENT_3D ( 'NONE', #61632, #16812, #60532 ) ;
#67053=CIRCLE ( 'NONE', #50976, 1.999999999999999556 ) ;
#67084=VERTEX_POINT ( 'NONE', #96559 ) ;
#67096=CARTESIAN_POINT ( 'NONE',  ( -9.604690719327259566E-16, 1522.051704408389924, 209.1218459616989946 ) ) ;
#67122=VERTEX_POINT ( 'NONE', #5240 ) ;
#67145=EDGE_LOOP ( 'NONE', ( #32572, #70074 ) ) ;
#67162=EDGE_CURVE ( 'NONE', #62788, #66505, #15273, .T. ) ;
#67196=VECTOR ( 'NONE', #11881, 1000.000000000000000 ) ;
#67209=EDGE_CURVE ( 'NONE', #34958, #108026, #109908, .T. ) ;
#67233=DIRECTION ( 'NONE',  ( -0.6736849260863839728, 0.000000000000000000, 0.7390186874254150995 ) ) ;
#67238=EDGE_CURVE ( 'NONE', #9574, #44418, #73950, .T. ) ;
#67256=DIRECTION ( 'NONE',  ( 5.980589973904019347E-17, -1.000000000000000000, 1.736889445713099699E-16 ) ) ;
#67280=CIRCLE ( 'NONE', #104829, 1.999999999999998668 ) ;
#67296=EDGE_LOOP ( 'NONE', ( #108681, #108837 ) ) ;
#67336=ORIENTED_EDGE ( 'NONE', *, *, #81902, .F. ) ;
#67341=CARTESIAN_POINT ( 'NONE',  ( 17.69507376876702764, 1521.951704408389787, 202.0148427140983358 ) ) ;
#67346=CARTESIAN_POINT ( 'NONE',  ( 17.71193101246160140, 1521.951704408389787, 196.6727161460330251 ) ) ;
#67349=DIRECTION ( 'NONE',  ( 0.9455185755993178454, 0.000000000000000000, -0.3255681544571539243 ) ) ;
#67364=AXIS2_PLACEMENT_3D ( 'NONE', #50137, #5168, #66211 ) ;
#67411=CARTESIAN_POINT ( 'NONE',  ( 7.878537825433329367, 1517.051704408389924, 200.0586249522280013 ) ) ;
#67422=DIRECTION ( 'NONE',  ( -1.755985294532469921E-16, 1.000000000000000000, -1.338183447452830017E-16 ) ) ;
#67460=DIRECTION ( 'NONE',  ( -1.755985294532469921E-16, 1.000000000000000000, -1.338183447452831989E-16 ) ) ;
#67494=DIRECTION ( 'NONE',  ( -5.980589973904019347E-17, 1.000000000000000000, -1.736889445713099699E-16 ) ) ;
#67512=VECTOR ( 'NONE', #428, 1000.000000000000000 ) ;
#67539=FACE_BOUND ( 'NONE', #70471, .T. ) ;
#67641=CIRCLE ( 'NONE', #92631, 1.999999999999999556 ) ;
#67693=FACE_OUTER_BOUND ( 'NONE', #5998, .T. ) ;
#67706=ORIENTED_EDGE ( 'NONE', *, *, #6266, .T. ) ;
#67741=CIRCLE ( 'NONE', #23022, 1.999999999999998668 ) ;
#67744=ORIENTED_EDGE ( 'NONE', *, *, #15362, .T. ) ;
#67786=CARTESIAN_POINT ( 'NONE',  ( -17.71193100849139768, 1519.551704408389924, 221.5709757781449980 ) ) ;
#67827=EDGE_CURVE ( 'NONE', #60554, #47910, #79910, .T. ) ;
#67861=ORIENTED_EDGE ( 'NONE', *, *, #97083, .F. ) ;
#67864=EDGE_LOOP ( 'NONE', ( #16475, #60962, #51402, #68667 ) ) ;
#67866=AXIS2_PLACEMENT_3D ( 'NONE', #3905, #38569, #106874 ) ;
#67869=CARTESIAN_POINT ( 'NONE',  ( 17.66551557756463353, 1521.951704408389787, 217.9010776241849214 ) ) ;
#67917=CARTESIAN_POINT ( 'NONE',  ( -13.77266209894789917, 1517.051704408389924, 217.0393652727940150 ) ) ;
#67925=LINE ( 'NONE', #22553, #5026 ) ;
#67965=CARTESIAN_POINT ( 'NONE',  ( -8.881784197001250351E-16, 1522.051704408389924, 209.1218459616989946 ) ) ;
#68006=ORIENTED_EDGE ( 'NONE', *, *, #104717, .T. ) ;
#68036=AXIS2_PLACEMENT_3D ( 'NONE', #11074, #19449, #80483 ) ;
#68039=CARTESIAN_POINT ( 'NONE',  ( 23.59335433453006559, 1521.951704408389787, 208.3625261891680793 ) ) ;
#68043=ORIENTED_EDGE ( 'NONE', *, *, #91812, .F. ) ;
#68054=CARTESIAN_POINT ( 'NONE',  ( 9.862951377358559313, 1517.151704408390060, 189.8497022443989977 ) ) ;
#68072=DIRECTION ( 'NONE',  ( -0.6736849260863837507, 0.000000000000000000, 0.7390186874254154326 ) ) ;
#68096=FACE_BOUND ( 'NONE', #30651, .T. ) ;
#68130=VECTOR ( 'NONE', #55471, 1000.000000000000000 ) ;
#68150=CIRCLE ( 'NONE', #94897, 2.000000000000003553 ) ;
#68199=DIRECTION ( 'NONE',  ( -5.980589973904019347E-17, 1.000000000000000000, -1.736889445713099699E-16 ) ) ;
#68212=ORIENTED_EDGE ( 'NONE', *, *, #28233, .F. ) ;
#68255=EDGE_LOOP ( 'NONE', ( #37400, #6420, #3771, #94376, #14475 ) ) ;
#68263=EDGE_CURVE ( 'NONE', #50393, #26041, #96388, .T. ) ;
#68278=ORIENTED_EDGE ( 'NONE', *, *, #30146, .T. ) ;
#68293=FACE_OUTER_BOUND ( 'NONE', #96845, .T. ) ;
#68359=EDGE_LOOP ( 'NONE', ( #8945, #63209 ) ) ;
#68369=DIRECTION ( 'NONE',  ( -5.980589973904019347E-17, 1.000000000000000000, -1.736889445713099699E-16 ) ) ;
#68373=CARTESIAN_POINT ( 'NONE',  ( 15.09047375999177021, 1517.151704408390060, 215.6125241866901661 ) ) ;
#68402=DIRECTION ( 'NONE',  ( -1.755985294532469921E-16, 1.000000000000000000, -1.338183447452831989E-16 ) ) ;
#68405=ORIENTED_EDGE ( 'NONE', *, *, #82518, .T. ) ;
#68418=EDGE_LOOP ( 'NONE', ( #58017, #76520, #15241, #79748, #21478 ) ) ;
#68581=LINE ( 'NONE', #68039, #75089 ) ;
#68585=EDGE_LOOP ( 'NONE', ( #32516, #98096 ) ) ;
#68603=CARTESIAN_POINT ( 'NONE',  ( -7.848979634317430509, 1522.051704408389924, 202.2988320601959913 ) ) ;
#68648=CARTESIAN_POINT ( 'NONE',  ( -10.18103031238528899, 1521.804095990992209, 184.9292055843479829 ) ) ;
#68649=CARTESIAN_POINT ( 'NONE',  ( -4.576312612474013441, 1522.051704408389924, 222.3843417993991807 ) ) ;
#68663=DIRECTION ( 'NONE',  ( -0.6736849260863841948, 0.000000000000000000, 0.7390186874254148774 ) ) ;
#68667=ORIENTED_EDGE ( 'NONE', *, *, #49464, .F. ) ;
#68672=EDGE_CURVE ( 'NONE', #103394, #66505, #69642, .T. ) ;
#68674=FACE_OUTER_BOUND ( 'NONE', #20869, .T. ) ;
#68686=CIRCLE ( 'NONE', #61501, 26.50000000000001421 ) ;
#68701=VERTEX_POINT ( 'NONE', #75110 ) ;
#68718=ORIENTED_EDGE ( 'NONE', *, *, #399, .T. ) ;
#68728=DIRECTION ( 'NONE',  ( 1.755985294532464991E-16, -1.000000000000000000, 1.338183447452830017E-16 ) ) ;
#68739=ORIENTED_EDGE ( 'NONE', *, *, #10303, .F. ) ;
#68755=DIRECTION ( 'NONE',  ( 5.980589973904019347E-17, -1.000000000000000000, 1.736889445713099699E-16 ) ) ;
#68757=ORIENTED_EDGE ( 'NONE', *, *, #73521, .T. ) ;
#68816=LINE ( 'NONE', #59854, #90068 ) ;
#68817=ORIENTED_EDGE ( 'NONE', *, *, #41315, .T. ) ;
#68848=VECTOR ( 'NONE', #31629, 1000.000000000000000 ) ;
#68855=CIRCLE ( 'NONE', #36628, 26.00000000000000711 ) ;
#68860=DIRECTION ( 'NONE',  ( -0.6736849260863840838, 0.000000000000000000, 0.7390186874254150995 ) ) ;
#68887=AXIS2_PLACEMENT_3D ( 'NONE', #24435, #31746, #58623 ) ;
#68894=CARTESIAN_POINT ( 'NONE',  ( 11.21032122953132948, 1517.151704408390060, 188.3716648695481695 ) ) ;
#68933=DIRECTION ( 'NONE',  ( -1.755985294532469921E-16, 1.000000000000000000, -1.338183447452831989E-16 ) ) ;
#68957=EDGE_LOOP ( 'NONE', ( #1983, #52448, #63071, #62018, #31194 ) ) ;
#68979=CARTESIAN_POINT ( 'NONE',  ( 11.83466398051542612, 1517.051704408389924, 190.1848878783540897 ) ) ;
#68982=CIRCLE ( 'NONE', #60021, 2.000000000000003109 ) ;
#69019=CIRCLE ( 'NONE', #83292, 2.000000000000003553 ) ;
#69022=CIRCLE ( 'NONE', #20690, 2.000000000000003553 ) ;
#69037=CARTESIAN_POINT ( 'NONE',  ( 17.71193101246160140, 1517.051704408389924, 196.6727161460330251 ) ) ;
#69046=DIRECTION ( 'NONE',  ( 0.9455185755993178454, 0.000000000000000000, -0.3255681544571537578 ) ) ;
#69049=VECTOR ( 'NONE', #37073, 1000.000000000000000 ) ;
#69054=DIRECTION ( 'NONE',  ( -5.980589973904019347E-17, 1.000000000000000000, -1.736889445713099699E-16 ) ) ;
#69116=ORIENTED_EDGE ( 'NONE', *, *, #88550, .T. ) ;
#69131=VERTEX_POINT ( 'NONE', #34605 ) ;
#69136=AXIS2_PLACEMENT_3D ( 'NONE', #20302, #54506, #73490 ) ;
#69158=EDGE_LOOP ( 'NONE', ( #109000, #34616, #29798, #13710, #92237 ) ) ;
#69159=CARTESIAN_POINT ( 'NONE',  ( -17.07488731192356823, 1522.051704408389924, 212.8400904445188075 ) ) ;
#69193=DIRECTION ( 'NONE',  ( -1.755985294532469921E-16, 1.000000000000000000, -1.338183447452831989E-16 ) ) ;
#69194=ORIENTED_EDGE ( 'NONE', *, *, #46086, .F. ) ;
#69224=EDGE_CURVE ( 'NONE', #82445, #92620, #7746, .T. ) ;
#69293=AXIS2_PLACEMENT_3D ( 'NONE', #77121, #96109, #427 ) ;
#69298=CARTESIAN_POINT ( 'NONE',  ( 3.968827104744170331, 1521.951704408389787, 188.7040005449509863 ) ) ;
#69320=AXIS2_PLACEMENT_3D ( 'NONE', #28348, #54681, #3727 ) ;
#69329=DIRECTION ( 'NONE',  ( -0.6736849260863839728, 0.000000000000000000, 0.7390186874254150995 ) ) ;
#69353=CARTESIAN_POINT ( 'NONE',  ( -1.984413551915469975, 1517.051704408389924, 219.3307686695569885 ) ) ;
#69362=ADVANCED_FACE ( 'NONE', ( #52213 ), #102567, .F. ) ;
#69383=EDGE_CURVE ( 'NONE', #54175, #18252, #74976, .T. ) ;
#69397=CARTESIAN_POINT ( 'NONE',  ( -8.456465142934460388, 1522.051704408389924, 195.1434824822571841 ) ) ;
#69409=AXIS2_PLACEMENT_3D ( 'NONE', #88025, #98037, #2378 ) ;
#69414=DIRECTION ( 'NONE',  ( -5.980589973904019347E-17, 1.000000000000000000, -1.736889445713099699E-16 ) ) ;
#69457=CARTESIAN_POINT ( 'NONE',  ( 11.75869035456349998, 1521.951704408389787, 227.2994842691620079 ) ) ;
#69482=AXIS2_PLACEMENT_3D ( 'NONE', #7441, #101474, #50008 ) ;
#69511=ORIENTED_EDGE ( 'NONE', *, *, #42085, .F. ) ;
#69539=CARTESIAN_POINT ( 'NONE',  ( -17.69507376891250416, 1519.551704408389924, 216.2288492090537488 ) ) ;
#69555=ADVANCED_FACE ( 'NONE', ( #39664 ), #48070, .F. ) ;
#69558=VERTEX_POINT ( 'NONE', #73832 ) ;
#69572=VECTOR ( 'NONE', #78688, 1000.000000000000000 ) ;
#69624=SURFACE_SIDE_STYLE ('',( #77991 ) ) ;
#69625=FACE_BOUND ( 'NONE', #42900, .T. ) ;
#69642=CIRCLE ( 'NONE', #46373, 1.999999999999997780 ) ;
#69667=AXIS2_PLACEMENT_3D ( 'NONE', #109380, #41615, #60086 ) ;
#69671=ORIENTED_EDGE ( 'NONE', *, *, #97914, .F. ) ;
#69694=EDGE_CURVE ( 'NONE', #98048, #53402, #46446, .T. ) ;
#69725=ORIENTED_EDGE ( 'NONE', *, *, #17197, .T. ) ;
#69764=DIRECTION ( 'NONE',  ( -0.6736849260863841948, 0.000000000000000000, 0.7390186874254148774 ) ) ;
#69781=ORIENTED_EDGE ( 'NONE', *, *, #94287, .T. ) ;
#69790=CIRCLE ( 'NONE', #62621, 1.999999999999998668 ) ;
#69836=CARTESIAN_POINT ( 'NONE',  ( 9.833393186232900263, 1522.051704408389924, 205.7359371553449989 ) ) ;
#69845=DIRECTION ( 'NONE',  ( -5.980589973904019347E-17, 1.000000000000000000, -1.736889445713099699E-16 ) ) ;
#69856=CARTESIAN_POINT ( 'NONE',  ( 1.925297169133120212, 1521.951704408389787, 230.6853930764029883 ) ) ;
#69866=VERTEX_POINT ( 'NONE', #35666 ) ;
#69899=DIRECTION ( 'NONE',  ( -0.9455185755993178454, 0.000000000000000000, 0.3255681544571537578 ) ) ;
#69911=EDGE_CURVE ( 'NONE', #76345, #28393, #53042, .T. ) ;
#69926=DIRECTION ( 'NONE',  ( -1.755985294532469921E-16, 1.000000000000000000, -1.338183447452831989E-16 ) ) ;
#69928=VERTEX_POINT ( 'NONE', #18297 ) ;
#70003=AXIS2_PLACEMENT_3D ( 'NONE', #47492, #107380, #64863 ) ;
#70030=VERTEX_POINT ( 'NONE', #31672 ) ;
#70047=EDGE_CURVE ( 'NONE', #87539, #1077, #85736, .T. ) ;
#70051=ORIENTED_EDGE ( 'NONE', *, *, #81129, .T. ) ;
#70074=ORIENTED_EDGE ( 'NONE', *, *, #78879, .T. ) ;
#70075=AXIS2_PLACEMENT_3D ( 'NONE', #76724, #92966, #52092 ) ;
#70087=ORIENTED_EDGE ( 'NONE', *, *, #39174, .F. ) ;
#70091=ORIENTED_EDGE ( 'NONE', *, *, #399, .F. ) ;
#70106=EDGE_CURVE ( 'NONE', #48574, #110694, #15955, .T. ) ;
#70116=AXIS2_PLACEMENT_3D ( 'NONE', #70731, #107590, #8834 ) ;
#70118=ORIENTED_EDGE ( 'NONE', *, *, #106265, .F. ) ;
#70157=VECTOR ( 'NONE', #62484, 1000.000000000000000 ) ;
#70193=EDGE_CURVE ( 'NONE', #39961, #42280, #96469, .T. ) ;
#70194=CIRCLE ( 'NONE', #5815, 1.999999999999999556 ) ;
#70202=EDGE_LOOP ( 'NONE', ( #45288, #13217, #13083, #50639 ) ) ;
#70220=ORIENTED_EDGE ( 'NONE', *, *, #30943, .T. ) ;
#70221=ORIENTED_EDGE ( 'NONE', *, *, #92897, .F. ) ;
#70251=DIRECTION ( 'NONE',  ( -1.755985294532469921E-16, 1.000000000000000000, -1.338183447452831989E-16 ) ) ;
#70271=CARTESIAN_POINT ( 'NONE',  ( 11.21032122953132770, 1522.051704408389924, 188.3716648695481695 ) ) ;
#70285=LINE ( 'NONE', #106055, #1443 ) ;
#70302=ORIENTED_EDGE ( 'NONE', *, *, #20671, .T. ) ;
#70313=FACE_BOUND ( 'NONE', #97456, .T. ) ;
#70320=VERTEX_POINT ( 'NONE', #33056 ) ;
#70324=CARTESIAN_POINT ( 'NONE',  ( 3.272667022753710242, 1517.151704408390060, 229.2073556998901438 ) ) ;
#70345=ORIENTED_EDGE ( 'NONE', *, *, #17243, .T. ) ;
#70392=DIRECTION ( 'NONE',  ( 1.755985294532464991E-16, -1.000000000000000000, 1.338183447452830017E-16 ) ) ;
#70452=FACE_OUTER_BOUND ( 'NONE', #107493, .T. ) ;
#70471=EDGE_LOOP ( 'NONE', ( #25628, #89572 ) ) ;
#70493=AXIS2_PLACEMENT_3D ( 'NONE', #82696, #48560, #66475 ) ;
#70497=ADVANCED_FACE ( 'NONE', ( #37483 ), #36922, .F. ) ;
#70501=ORIENTED_EDGE ( 'NONE', *, *, #3914, .F. ) ;
#70522=CARTESIAN_POINT ( 'NONE',  ( 19.63722818192610120, 1519.551704408389924, 218.2362632616380154 ) ) ;
#70523=DIRECTION ( 'NONE',  ( -1.755985294532469921E-16, 1.000000000000000000, -1.338183447452831989E-16 ) ) ;
#70554=EDGE_CURVE ( 'NONE', #42052, #35207, #99020, .T. ) ;
#70556=ORIENTED_EDGE ( 'NONE', *, *, #26068, .F. ) ;
#70558=VERTEX_POINT ( 'NONE', #49206 ) ;
#70573=EDGE_LOOP ( 'NONE', ( #76639, #69725 ) ) ;
#70587=ADVANCED_FACE ( 'NONE', ( #40231 ), #22296, .F. ) ;
#70589=LINE ( 'NONE', #53794, #37602 ) ;
#70621=DIRECTION ( 'NONE',  ( -1.755985294532469921E-16, 1.000000000000000000, -1.338183447452831989E-16 ) ) ;
#70646=CARTESIAN_POINT ( 'NONE',  ( -3.897009771321176874, 1517.051704408389924, 187.2231132109079113 ) ) ;
#70669=ORIENTED_EDGE ( 'NONE', *, *, #48875, .F. ) ;
#70677=CARTESIAN_POINT ( 'NONE',  ( 13.73040296012064587, 1519.551704408389924, 227.6346699041483816 ) ) ;
#70690=DIRECTION ( 'NONE',  ( 1.755985294532464991E-16, -1.000000000000000000, 1.338183447452830017E-16 ) ) ;
#70731=CARTESIAN_POINT ( 'NONE',  ( -21.62164173326539895, 1517.051704408389924, 210.2163513712909833 ) ) ;
#70751=CARTESIAN_POINT ( 'NONE',  ( -22.96901158596647008, 1519.551704408389924, 211.6943887467578236 ) ) ;
#70769=VERTEX_POINT ( 'NONE', #110743 ) ;
#70773=CARTESIAN_POINT ( 'NONE',  ( -13.74310390781900004, 1522.051704408389924, 201.1531303618569950 ) ) ;
#70780=CARTESIAN_POINT ( 'NONE',  ( 12.42529224677512900, 1517.151704408390060, 202.6823640254548309 ) ) ;
#70786=EDGE_LOOP ( 'NONE', ( #53152, #76036 ) ) ;
#70807=CIRCLE ( 'NONE', #77945, 1.999999999999998446 ) ;
#70882=CARTESIAN_POINT ( 'NONE',  ( -1.997114497637953789, 1521.951704408389787, 229.8748770088220965 ) ) ;
#70952=DIRECTION ( 'NONE',  ( 0.9455185755993178454, 0.000000000000000000, -0.3255681544571537578 ) ) ;
#70983=CARTESIAN_POINT ( 'NONE',  ( -13.74310390781900004, 1517.151704408390060, 201.1531303618569950 ) ) ;
#71003=CARTESIAN_POINT ( 'NONE',  ( -9.225907677606098645, 1517.151704408390060, 219.6631043460218393 ) ) ;
#71022=CARTESIAN_POINT ( 'NONE',  ( -1.925297170580940076, 1517.151704408390060, 187.5582988486569889 ) ) ;
#71038=DIRECTION ( 'NONE',  ( -5.980589973904019347E-17, 1.000000000000000000, -1.736889445713099699E-16 ) ) ;
#71046=AXIS2_PLACEMENT_3D ( 'NONE', #84226, #59054, #60724 ) ;
#71110=ORIENTED_EDGE ( 'NONE', *, *, #80164, .F. ) ;
#71129=ORIENTED_EDGE ( 'NONE', *, *, #67209, .T. ) ;
#71141=AXIS2_PLACEMENT_3D ( 'NONE', #109229, #102998, #32513 ) ;
#71167=ORIENTED_EDGE ( 'NONE', *, *, #51660, .F. ) ;
#71181=ORIENTED_EDGE ( 'NONE', *, *, #30146, .F. ) ;
#71184=ORIENTED_EDGE ( 'NONE', *, *, #40774, .F. ) ;
#71224=ADVANCED_FACE ( 'NONE', ( #62894 ), #12425, .F. ) ;
#71252=CIRCLE ( 'NONE', #22900, 1.999999999999999556 ) ;
#71275=CARTESIAN_POINT ( 'NONE',  ( 13.77266209894789917, 1517.051704408389924, 201.2043266506040027 ) ) ;
#71398=DIRECTION ( 'NONE',  ( -1.755985294532469921E-16, 1.000000000000000000, -1.338183447452831989E-16 ) ) ;
#71413=CIRCLE ( 'NONE', #57075, 1.999999999999999556 ) ;
#71448=CARTESIAN_POINT ( 'NONE',  ( -11.75869035456349998, 1517.051704408389924, 190.9442076542370046 ) ) ;
#71473=CARTESIAN_POINT ( 'NONE',  ( 17.66551557756463353, 1517.051704408389924, 217.9010776241849214 ) ) ;
#71475=CYLINDRICAL_SURFACE ( 'NONE', #101694, 2.000000000000003553 ) ;
#71488=ORIENTED_EDGE ( 'NONE', *, *, #66667, .T. ) ;
#71504=ORIENTED_EDGE ( 'NONE', *, *, #61306, .T. ) ;
#71543=VECTOR ( 'NONE', #23690, 1000.000000000000000 ) ;
#71569=ORIENTED_EDGE ( 'NONE', *, *, #40687, .T. ) ;
#71573=CARTESIAN_POINT ( 'NONE',  ( -7.878537825433329367, 1517.051704408389924, 218.1850669711710111 ) ) ;
#71592=LINE ( 'NONE', #62635, #101875 ) ;
#71599=ORIENTED_EDGE ( 'NONE', *, *, #40017, .T. ) ;
#71619=ORIENTED_EDGE ( 'NONE', *, *, #61025, .F. ) ;
#71662=AXIS2_PLACEMENT_3D ( 'NONE', #71022, #27881, #28432 ) ;
#71669=DIRECTION ( 'NONE',  ( -0.6736849260863839728, 0.000000000000000000, 0.7390186874254150995 ) ) ;
#71672=VERTEX_POINT ( 'NONE', #31585 ) ;
#71680=ORIENTED_EDGE ( 'NONE', *, *, #32333, .F. ) ;
#71781=DIRECTION ( 'NONE',  ( -0.6736849260863841948, 0.000000000000000000, 0.7390186874254148774 ) ) ;
#71795=VECTOR ( 'NONE', #22792, 1000.000000000000000 ) ;
#71861=LINE ( 'NONE', #89703, #97621 ) ;
#71877=VERTEX_POINT ( 'NONE', #77469 ) ;
#71913=EDGE_CURVE ( 'NONE', #86132, #10824, #46521, .T. ) ;
#71920=EDGE_CURVE ( 'NONE', #70558, #67122, #41144, .T. ) ;
#71960=EDGE_CURVE ( 'NONE', #39586, #97416, #69790, .T. ) ;
#71998=CARTESIAN_POINT ( 'NONE',  ( 17.68237282055029880, 1517.151704408390060, 212.5589510568480023 ) ) ;
#72020=CIRCLE ( 'NONE', #9174, 3.999999999999997335 ) ;
#72045=EDGE_LOOP ( 'NONE', ( #98909, #36433 ) ) ;
#72047=DIRECTION ( 'NONE',  ( 1.755985294532464991E-16, -1.000000000000000000, 1.338183447452830017E-16 ) ) ;
#72050=EDGE_CURVE ( 'NONE', #88934, #26765, #1848, .T. ) ;
#72051=CARTESIAN_POINT ( 'NONE',  ( -13.74310390781900004, 1517.051704408389924, 201.1531303618569950 ) ) ;
#72071=DIRECTION ( 'NONE',  ( -0.9455185755993178454, 0.000000000000000000, 0.3255681544571539798 ) ) ;
#72123=EDGE_LOOP ( 'NONE', ( #55598, #15443, #81732, #15631 ) ) ;
#72125=ADVANCED_FACE ( 'NONE', ( #11766 ), #62200, .F. ) ;
#72146=DIRECTION ( 'NONE',  ( -0.6736849260863839728, 0.000000000000000000, 0.7390186874254150995 ) ) ;
#72152=CARTESIAN_POINT ( 'NONE',  ( -7.005862043813290743E-15, 1521.551704408389924, 209.1218459616989946 ) ) ;
#72171=ORIENTED_EDGE ( 'NONE', *, *, #41765, .F. ) ;
#72199=FACE_OUTER_BOUND ( 'NONE', #73778, .T. ) ;
#72206=ORIENTED_EDGE ( 'NONE', *, *, #89185, .F. ) ;
#72223=VERTEX_POINT ( 'NONE', #24548 ) ;
#72254=DIRECTION ( 'NONE',  ( -0.9455185755993178454, 0.000000000000000000, 0.3255681544571537578 ) ) ;
#72261=CYLINDRICAL_SURFACE ( 'NONE', #101016, 2.000000000000003553 ) ;
#72269=EDGE_LOOP ( 'NONE', ( #13663, #54773, #2743, #91234, #72171 ) ) ;
#72299=SHAPE_REPRESENTATION ( 'Grinding Plate', ( #21632 ), #61094 ) ;
#72324=ADVANCED_FACE ( 'NONE', ( #17241 ), #62501, .F. ) ;
#72394=CARTESIAN_POINT ( 'NONE',  ( 11.21032122953132770, 1519.551704408389924, 188.3716648695481695 ) ) ;
#72424=DIRECTION ( 'NONE',  ( -0.6736849260863839728, 0.000000000000000000, 0.7390186874254150995 ) ) ;
#72432=EDGE_CURVE ( 'NONE', #75633, #22619, #30430, .T. ) ;
#72436=DIRECTION ( 'NONE',  ( 0.9455185755993167351, 0.000000000000000000, -0.3255681544571568109 ) ) ;
#72465=ORIENTED_EDGE ( 'NONE', *, *, #54269, .F. ) ;
#72476=AXIS2_PLACEMENT_3D ( 'NONE', #6827, #119, #49954 ) ;
#72519=EDGE_LOOP ( 'NONE', ( #56664, #20 ) ) ;
#72525=ORIENTED_EDGE ( 'NONE', *, *, #42564, .T. ) ;
#72576=DIRECTION ( 'NONE',  ( -0.9455185755993178454, 0.000000000000000000, 0.3255681544571537578 ) ) ;
#72630=FACE_OUTER_BOUND ( 'NONE', #51056, .T. ) ;
#72631=EDGE_CURVE ( 'NONE', #30342, #86629, #94773, .T. ) ;
#72705=CARTESIAN_POINT ( 'NONE',  ( -15.74021840509336556, 1519.551704408389924, 221.9061614126840425 ) ) ;
#72745=DIRECTION ( 'NONE',  ( 1.755985294532464991E-16, -1.000000000000000000, 1.338183447452830017E-16 ) ) ;
#72756=ORIENTED_EDGE ( 'NONE', *, *, #5777, .F. ) ;
#72797=ORIENTED_EDGE ( 'NONE', *, *, #10580, .F. ) ;
#72808=ORIENTED_EDGE ( 'NONE', *, *, #58984, .T. ) ;
#72828=DIRECTION ( 'NONE',  ( -1.755985294532469921E-16, 1.000000000000000000, -1.338183447452831989E-16 ) ) ;
#72829=CIRCLE ( 'NONE', #24510, 1.999999999999998668 ) ;
#72836=AXIS2_PLACEMENT_3D ( 'NONE', #6074, #84439, #74956 ) ;
#72839=CARTESIAN_POINT ( 'NONE',  ( -5.864566082395439750, 1517.051704408389924, 192.0899093523580063 ) ) ;
#72843=CARTESIAN_POINT ( 'NONE',  ( 21.01415622463856891, 1519.551704408389924, 200.8719909741391803 ) ) ;
#72852=FACE_OUTER_BOUND ( 'NONE', #26102, .T. ) ;
#72967=DIRECTION ( 'NONE',  ( 0.9455185755993178454, 0.000000000000000000, -0.3255681544571537578 ) ) ;
#72968=AXIS2_PLACEMENT_3D ( 'NONE', #64509, #81269, #80189 ) ;
#72999=CIRCLE ( 'NONE', #24665, 2.000000000000003553 ) ;
#73038=FACE_BOUND ( 'NONE', #15460, .T. ) ;
#73064=ORIENTED_EDGE ( 'NONE', *, *, #42085, .T. ) ;
#73107=DIRECTION ( 'NONE',  ( -1.755985294532469921E-16, 1.000000000000000000, -1.338183447452831989E-16 ) ) ;
#73117=DIRECTION ( 'NONE',  ( 0.9455185755993178454, 0.000000000000000000, -0.3255681544571537578 ) ) ;
#73154=EDGE_LOOP ( 'NONE', ( #25288, #58141, #67011, #88147 ) ) ;
#73214=CARTESIAN_POINT ( 'NONE',  ( -6.790918657024139549, 1522.051704408389924, 184.0243675267330161 ) ) ;
#73221=CIRCLE ( 'NONE', #35643, 1.749999999999996891 ) ;
#73229=ORIENTED_EDGE ( 'NONE', *, *, #14108, .F. ) ;
#73230=LINE ( 'NONE', #106813, #21306 ) ;
#73241=CIRCLE ( 'NONE', #108970, 1.999999999999999556 ) ;
#73260=FACE_OUTER_BOUND ( 'NONE', #25759, .T. ) ;
#73261=ORIENTED_EDGE ( 'NONE', *, *, #48911, .T. ) ;
#73272=ADVANCED_FACE ( 'NONE', ( #64437 ), #96926, .F. ) ;
#73276=FACE_OUTER_BOUND ( 'NONE', #90055, .T. ) ;
#73283=ORIENTED_EDGE ( 'NONE', *, *, #108925, .F. ) ;
#73298=CYLINDRICAL_SURFACE ( 'NONE', #91146, 2.000000000000003109 ) ;
#73299=CARTESIAN_POINT ( 'NONE',  ( -9.786977751178733698, 1517.051704408389924, 191.2793932888540951 ) ) ;
#73341=ORIENTED_EDGE ( 'NONE', *, *, #3657, .T. ) ;
#73345=VERTEX_POINT ( 'NONE', #63346 ) ;
#73351=ORIENTED_EDGE ( 'NONE', *, *, #3139, .F. ) ;
#73368=CIRCLE ( 'NONE', #80493, 1.999999999999999556 ) ;
#73378=ADVANCED_FACE ( 'NONE', ( #20193 ), #28610, .F. ) ;
#73401=DIRECTION ( 'NONE',  ( -5.980589973904019347E-17, 1.000000000000000000, -1.736889445713099699E-16 ) ) ;
#73409=FACE_OUTER_BOUND ( 'NONE', #108603, .T. ) ;
#73418=AXIS2_PLACEMENT_3D ( 'NONE', #12521, #56732, #106576 ) ;
#73451=AXIS2_PLACEMENT_3D ( 'NONE', #96724, #94487, #69329 ) ;
#73471=ORIENTED_EDGE ( 'NONE', *, *, #103731, .F. ) ;
#73490=DIRECTION ( 'NONE',  ( -0.6736849260863841948, 0.000000000000000000, 0.7390186874254148774 ) ) ;
#73492=ORIENTED_EDGE ( 'NONE', *, *, #96617, .F. ) ;
#73496=CIRCLE ( 'NONE', #53854, 1.999999999999999556 ) ;
#73507=ORIENTED_EDGE ( 'NONE', *, *, #109924, .T. ) ;
#73519=CARTESIAN_POINT ( 'NONE',  ( -1.925297170580940076, 1519.551704408389924, 187.5582988486569889 ) ) ;
#73521=EDGE_CURVE ( 'NONE', #71877, #67084, #10870, .T. ) ;
#73552=ORIENTED_EDGE ( 'NONE', *, *, #17108, .F. ) ;
#73571=CARTESIAN_POINT ( 'NONE',  ( -11.75869035456349998, 1517.051704408389924, 190.9442076542370046 ) ) ;
#73586=AXIS2_PLACEMENT_3D ( 'NONE', #99843, #105099, #92009 ) ;
#73628=ORIENTED_EDGE ( 'NONE', *, *, #27754, .F. ) ;
#73629=ORIENTED_EDGE ( 'NONE', *, *, #832, .T. ) ;
#73630=LINE ( 'NONE', #74181, #84150 ) ;
#73636=ORIENTED_EDGE ( 'NONE', *, *, #104265, .F. ) ;
#73638=DIRECTION ( 'NONE',  ( 1.755985294532464991E-16, -1.000000000000000000, 1.338183447452830017E-16 ) ) ;
#73687=AXIS2_PLACEMENT_3D ( 'NONE', #294, #27133, #18702 ) ;
#73778=EDGE_LOOP ( 'NONE', ( #31457, #19168, #72465, #15683 ) ) ;
#73795=ORIENTED_EDGE ( 'NONE', *, *, #12307, .F. ) ;
#73800=CARTESIAN_POINT ( 'NONE',  ( -15.69795926999090163, 1519.551704408389924, 195.4758181584410011 ) ) ;
#73826=ORIENTED_EDGE ( 'NONE', *, *, #77582, .T. ) ;
#73827=ORIENTED_EDGE ( 'NONE', *, *, #20671, .F. ) ;
#73832=CARTESIAN_POINT ( 'NONE',  ( 18.28985832975333281, 1519.551704408389924, 219.7143006364888436 ) ) ;
#73848=ORIENTED_EDGE ( 'NONE', *, *, #59607, .F. ) ;
#73863=DIRECTION ( 'NONE',  ( 1.755985294532464991E-16, -1.000000000000000000, 1.338183447452830017E-16 ) ) ;
#73884=CARTESIAN_POINT ( 'NONE',  ( -19.63722818156799832, 1519.551704408389924, 200.0074286628000095 ) ) ;
#73899=ORIENTED_EDGE ( 'NONE', *, *, #78055, .T. ) ;
#73950=CIRCLE ( 'NONE', #36372, 1.999999999999999556 ) ;
#73989=CARTESIAN_POINT ( 'NONE',  ( -11.75869035857540013, 1519.551704408389924, 190.9442076533970010 ) ) ;
#74019=CARTESIAN_POINT ( 'NONE',  ( -11.81780673814840021, 1522.051704408389924, 222.7166774759110126 ) ) ;
#74040=EDGE_CURVE ( 'NONE', #58638, #4755, #34021, .T. ) ;
#74063=DIRECTION ( 'NONE',  ( 0.9858563016923833633, 0.000000000000000000, 0.1675928173085483863 ) ) ;
#74092=CARTESIAN_POINT ( 'NONE',  ( -5.923682464646780943, 1522.051704408389924, 223.8623791742500089 ) ) ;
#74123=CARTESIAN_POINT ( 'NONE',  ( 13.74310390781900004, 1522.051704408389924, 217.0905615615409943 ) ) ;
#74152=FACE_BOUND ( 'NONE', #36967, .T. ) ;
#74156=ORIENTED_EDGE ( 'NONE', *, *, #90539, .F. ) ;
#74166=DIRECTION ( 'NONE',  ( 0.9858563016923833633, 0.000000000000000000, 0.1675928173085483863 ) ) ;
#74181=CARTESIAN_POINT ( 'NONE',  ( 9.786977751178733698, 1521.951704408389787, 226.9642986345448890 ) ) ;
#74191=CARTESIAN_POINT ( 'NONE',  ( 17.71193101166619854, 1519.551704408389924, 196.6727161458730109 ) ) ;
#74232=DIRECTION ( 'NONE',  ( 0.2302114497549562488, 0.7071067811868637643, 0.6685825965438183527 ) ) ;
#74235=ORIENTED_EDGE ( 'NONE', *, *, #48155, .T. ) ;
#74291=ORIENTED_EDGE ( 'NONE', *, *, #18490, .F. ) ;
#74324=VECTOR ( 'NONE', #33134, 1000.000000000000000 ) ;
#74327=LINE ( 'NONE', #81582, #45437 ) ;
#74345=LINE ( 'NONE', #84904, #9206 ) ;
#74350=DIRECTION ( 'NONE',  ( -1.755985294532469921E-16, 1.000000000000000000, -1.338183447452831989E-16 ) ) ;
#74359=CARTESIAN_POINT ( 'NONE',  ( 11.78824854703250047, 1517.151704408390060, 211.4132493584619965 ) ) ;
#74378=DIRECTION ( 'NONE',  ( -0.9455185755993178454, 0.000000000000000000, 0.3255681544571539243 ) ) ;
#74383=CARTESIAN_POINT ( 'NONE',  ( -3.909710721586109550, 1522.051704408389924, 197.7672215555029993 ) ) ;
#74406=AXIS2_PLACEMENT_3D ( 'NONE', #19081, #94708, #10154 ) ;
#74460=EDGE_LOOP ( 'NONE', ( #83011, #73064, #93577, #48627, #29691 ) ) ;
#74495=ORIENTED_EDGE ( 'NONE', *, *, #49785, .T. ) ;
#74502=ORIENTED_EDGE ( 'NONE', *, *, #19994, .F. ) ;
#74508=CARTESIAN_POINT ( 'NONE',  ( -13.10606021074817207, 1517.151704408390060, 192.4222450282478292 ) ) ;
#74511=CARTESIAN_POINT ( 'NONE',  ( 0.6370436997426999204, 1517.151704408390060, 200.3909606286928238 ) ) ;
#74535=FACE_OUTER_BOUND ( 'NONE', #28146, .T. ) ;
#74548=ORIENTED_EDGE ( 'NONE', *, *, #34733, .T. ) ;
#74600=DIRECTION ( 'NONE',  ( -0.6736849260863837507, 0.000000000000000000, 0.7390186874254154326 ) ) ;
#74618=DIRECTION ( 'NONE',  ( -1.755985294532469921E-16, 1.000000000000000000, -1.338183447452831989E-16 ) ) ;
#74624=CARTESIAN_POINT ( 'NONE',  ( -11.18076303840566865, 1522.051704408389924, 213.9857921429048417 ) ) ;
#74626=EDGE_LOOP ( 'NONE', ( #58600, #76180 ) ) ;
#74632=CARTESIAN_POINT ( 'NONE',  ( -6.531167973260561865, 1522.051704408389924, 216.7070295963201829 ) ) ;
#74640=FACE_OUTER_BOUND ( 'NONE', #37529, .T. ) ;
#74653=ADVANCED_FACE ( 'NONE', ( #17224 ), #85551, .F. ) ;
#74685=CARTESIAN_POINT ( 'NONE',  ( -21.62164173326539895, 1521.951704408389787, 210.2163513712909833 ) ) ;
#74698=CIRCLE ( 'NONE', #6809, 1.999999999999997780 ) ;
#74771=CYLINDRICAL_SURFACE ( 'NONE', #104105, 2.000000000000003553 ) ;
#74799=AXIS2_PLACEMENT_3D ( 'NONE', #26745, #2689, #105123 ) ;
#74827=AXIS2_PLACEMENT_3D ( 'NONE', #46033, #20242, #80718 ) ;
#74830=ADVANCED_FACE ( 'NONE', ( #23858 ), #58050, .F. ) ;
#74831=FACE_BOUND ( 'NONE', #3965, .T. ) ;
#74839=AXIS2_PLACEMENT_3D ( 'NONE', #21966, #14140, #99794 ) ;
#74901=EDGE_CURVE ( 'NONE', #69928, #103394, #52963, .T. ) ;
#74949=CARTESIAN_POINT ( 'NONE',  ( 0.5779273184081700210, 1517.151704408390060, 232.1634304495918002 ) ) ;
#74952=ORIENTED_EDGE ( 'NONE', *, *, #38978, .F. ) ;
#74956=DIRECTION ( 'NONE',  ( -0.9455185755993178454, 0.000000000000000000, 0.3255681544571539243 ) ) ;
#74959=CARTESIAN_POINT ( 'NONE',  ( 7.211935934568218798, 1522.051704408389924, 224.6757451961901495 ) ) ;
#74976=CIRCLE ( 'NONE', #26665, 1.999999999999998890 ) ;
#75052=AXIS2_PLACEMENT_3D ( 'NONE', #82202, #5506, #22829 ) ;
#75072=DIRECTION ( 'NONE',  ( -0.6736849260863841948, 0.000000000000000000, 0.7390186874254148774 ) ) ;
#75089=VECTOR ( 'NONE', #32750, 1000.000000000000000 ) ;
#75090=DIRECTION ( 'NONE',  ( -5.980589973904019347E-17, 1.000000000000000000, -1.736889445713099699E-16 ) ) ;
#75110=CARTESIAN_POINT ( 'NONE',  ( -9.225907677606096868, 1517.051704408389924, 219.6631043460218393 ) ) ;
#75119=ORIENTED_EDGE ( 'NONE', *, *, #69694, .F. ) ;
#75169=DIRECTION ( 'NONE',  ( -0.6736849260863841948, 0.000000000000000000, 0.7390186874254148774 ) ) ;
#75175=FACE_OUTER_BOUND ( 'NONE', #109601, .T. ) ;
#75187=VERTEX_POINT ( 'NONE', #72394 ) ;
#75190=CYLINDRICAL_SURFACE ( 'NONE', #92495, 1.999999999999999556 ) ;
#75227=CIRCLE ( 'NONE', #53747, 1.999999999999998668 ) ;
#75247=CARTESIAN_POINT ( 'NONE',  ( -17.71193101166619854, 1517.051704408389924, 221.5709757775249784 ) ) ;
#75258=VERTEX_POINT ( 'NONE', #58880 ) ;
#75305=DIRECTION ( 'NONE',  ( 0.9455185755993178454, 0.000000000000000000, -0.3255681544571537578 ) ) ;
#75309=CIRCLE ( 'NONE', #109267, 1.999999999999999556 ) ;
#75332=CARTESIAN_POINT ( 'NONE',  ( 9.196349486490202452, 1517.151704408390060, 214.4668224883511698 ) ) ;
#75346=DIRECTION ( 'NONE',  ( -0.6736849260863841948, 0.000000000000000000, 0.7390186874254148774 ) ) ;
#75356=DIRECTION ( 'NONE',  ( -1.755985294532469921E-16, 1.000000000000000000, -1.338183447452831989E-16 ) ) ;
#75357=DIRECTION ( 'NONE',  ( 1.755985294532464991E-16, -1.000000000000000000, 1.338183447452830017E-16 ) ) ;
#75383=EDGE_CURVE ( 'NONE', #48151, #39586, #63310, .T. ) ;
#75386=FACE_BOUND ( 'NONE', #103678, .T. ) ;
#75387=STYLED_ITEM ( 'NONE', ( #48417 ), #19969 ) ;
#75412=CIRCLE ( 'NONE', #70075, 1.999999999999999556 ) ;
#75456=EDGE_CURVE ( 'NONE', #106669, #31574, #24975, .T. ) ;
#75490=DIRECTION ( 'NONE',  ( -5.980589973904019347E-17, 1.000000000000000000, -1.736889445713099699E-16 ) ) ;
#75509=FACE_OUTER_BOUND ( 'NONE', #8317, .T. ) ;
#75535=CARTESIAN_POINT ( 'NONE',  ( 3.968827104744170331, 1517.051704408389924, 188.7040005449509863 ) ) ;
#75563=EDGE_CURVE ( 'NONE', #110607, #102937, #37481, .T. ) ;
#75580=LINE ( 'NONE', #16713, #94457 ) ;
#75633=VERTEX_POINT ( 'NONE', #15822 ) ;
#75687=CYLINDRICAL_SURFACE ( 'NONE', #15456, 2.000000000000003109 ) ;
#75704=VERTEX_POINT ( 'NONE', #9118 ) ;
#75707=VERTEX_POINT ( 'NONE', #76881 ) ;
#75726=CARTESIAN_POINT ( 'NONE',  ( -21.62164173379369814, 1519.551704408389924, 210.2163513719069954 ) ) ;
#75752=DIRECTION ( 'NONE',  ( 1.755985294532464991E-16, -1.000000000000000000, 1.338183447452830017E-16 ) ) ;
#75786=CIRCLE ( 'NONE', #22110, 1.999999999999999556 ) ;
#75792=FACE_BOUND ( 'NONE', #58355, .T. ) ;
#75824=DIRECTION ( 'NONE',  ( 0.9455185755993177343, 0.000000000000000000, -0.3255681544571540909 ) ) ;
#75859=CARTESIAN_POINT ( 'NONE',  ( 11.78824854703250047, 1522.051704408389924, 211.4132493584619965 ) ) ;
#75891=CARTESIAN_POINT ( 'NONE',  ( 7.878537825433329367, 1517.151704408390060, 200.0586249522280013 ) ) ;
#75916=FACE_BOUND ( 'NONE', #88426, .T. ) ;
#75999=CARTESIAN_POINT ( 'NONE',  ( 17.69507376911758101, 1519.551704408389924, 202.0148427141579361 ) ) ;
#76002=DIRECTION ( 'NONE',  ( 0.9455185755993178454, 0.000000000000000000, -0.3255681544571537578 ) ) ;
#76035=VERTEX_POINT ( 'NONE', #8976 ) ;
#76036=ORIENTED_EDGE ( 'NONE', *, *, #7436, .T. ) ;
#76059=ADVANCED_FACE ( 'NONE', ( #85127 ), #1157, .F. ) ;
#76061=DIRECTION ( 'NONE',  ( 0.9455185755993178454, 0.000000000000000000, -0.3255681544571537578 ) ) ;
#76084=EDGE_LOOP ( 'NONE', ( #108656, #2798 ) ) ;
#76100=ORIENTED_EDGE ( 'NONE', *, *, #45994, .T. ) ;
#76114=ORIENTED_EDGE ( 'NONE', *, *, #24699, .F. ) ;
#76163=CYLINDRICAL_SURFACE ( 'NONE', #12117, 2.000000000000003553 ) ;
#76170=DIRECTION ( 'NONE',  ( -0.6736849260863841948, 0.000000000000000000, 0.7390186874254148774 ) ) ;
#76180=ORIENTED_EDGE ( 'NONE', *, *, #39174, .T. ) ;
#76210=VERTEX_POINT ( 'NONE', #45799 ) ;
#76253=DIRECTION ( 'NONE',  ( 1.755985294532469921E-16, -1.000000000000000000, 1.338183447452831989E-16 ) ) ;
#76260=DIRECTION ( 'NONE',  ( 5.980589973904019347E-17, -1.000000000000000000, 1.736889445713099699E-16 ) ) ;
#76262=ADVANCED_FACE ( 'NONE', ( #104013 ), #54748, .F. ) ;
#76276=ADVANCED_FACE ( 'NONE', ( #70452 ), #104572, .F. ) ;
#76286=ORIENTED_EDGE ( 'NONE', *, *, #84896, .F. ) ;
#76339=FACE_BOUND ( 'NONE', #43065, .T. ) ;
#76343=AXIS2_PLACEMENT_3D ( 'NONE', #88042, #721, #43814 ) ;
#76345=VERTEX_POINT ( 'NONE', #81557 ) ;
#76390=CIRCLE ( 'NONE', #96055, 1.999999999999999556 ) ;
#76407=AXIS2_PLACEMENT_3D ( 'NONE', #106986, #64466, #98582 ) ;
#76480=DIRECTION ( 'NONE',  ( -0.6736849260863841948, 0.000000000000000000, 0.7390186874254148774 ) ) ;
#76507=VERTEX_POINT ( 'NONE', #64808 ) ;
#76510=CARTESIAN_POINT ( 'NONE',  ( -11.83466398015730725, 1521.951704408389787, 228.0588040460849015 ) ) ;
#76520=ORIENTED_EDGE ( 'NONE', *, *, #2344, .T. ) ;
#76588=CARTESIAN_POINT ( 'NONE',  ( -8.301987938657498844, 1519.551704408389924, 185.0111222839169898 ) ) ;
#76604=DIRECTION ( 'NONE',  ( 0.9455185755993178454, 0.000000000000000000, -0.3255681544571537578 ) ) ;
#76639=ORIENTED_EDGE ( 'NONE', *, *, #106228, .T. ) ;
#76724=CARTESIAN_POINT ( 'NONE',  ( -9.833393186232889605, 1517.051704408389924, 212.5077547680540135 ) ) ;
#76729=ORIENTED_EDGE ( 'NONE', *, *, #32467, .T. ) ;
#76777=ORIENTED_EDGE ( 'NONE', *, *, #19379, .T. ) ;
#76781=CARTESIAN_POINT ( 'NONE',  ( -21.62164173326539895, 1521.951704408389787, 210.2163513712909833 ) ) ;
#76798=EDGE_CURVE ( 'NONE', #99771, #65489, #14359, .T. ) ;
#76819=AXIS2_PLACEMENT_3D ( 'NONE', #78760, #2076, #52470 ) ;
#76835=DIRECTION ( 'NONE',  ( -5.980589973904019347E-17, 1.000000000000000000, -1.736889445713099699E-16 ) ) ;
#76881=CARTESIAN_POINT ( 'NONE',  ( -10.47043688597563182, 1517.051704408389924, 221.2386401010601844 ) ) ;
#76940=ORIENTED_EDGE ( 'NONE', *, *, #87682, .T. ) ;
#76952=CARTESIAN_POINT ( 'NONE',  ( -13.77266209894789917, 1522.051704408389924, 217.0393652727940150 ) ) ;
#76965=ORIENTED_EDGE ( 'NONE', *, *, #60452, .F. ) ;
#76986=CARTESIAN_POINT ( 'NONE',  ( -19.63722818134010240, 1521.951704408389787, 200.0074286634620364 ) ) ;
#77004=VECTOR ( 'NONE', #61163, 1000.000000000000000 ) ;
#77032=FACE_BOUND ( 'NONE', #95499, .T. ) ;
#77064=VERTEX_POINT ( 'NONE', #47863 ) ;
#77066=AXIS2_PLACEMENT_3D ( 'NONE', #76952, #262, #94847 ) ;
#77095=ORIENTED_EDGE ( 'NONE', *, *, #30943, .F. ) ;
#77104=DIRECTION ( 'NONE',  ( -0.9455185755993178454, 0.000000000000000000, 0.3255681544571537578 ) ) ;
#77105=FACE_OUTER_BOUND ( 'NONE', #99988, .T. ) ;
#77121=CARTESIAN_POINT ( 'NONE',  ( -1.984413551915469975, 1517.151704408390060, 219.3307686695569885 ) ) ;
#77144=DIRECTION ( 'NONE',  ( 0.9858563016923833633, 0.000000000000000000, 0.1675928173085483863 ) ) ;
#77161=AXIS2_PLACEMENT_3D ( 'NONE', #74123, #108253, #66288 ) ;
#77205=DIRECTION ( 'NONE',  ( 1.755985294532464991E-16, -1.000000000000000000, 1.338183447452830017E-16 ) ) ;
#77228=CYLINDRICAL_SURFACE ( 'NONE', #13971, 1.999999999999999556 ) ;
#77275=AXIS2_PLACEMENT_3D ( 'NONE', #34049, #41905, #76061 ) ;
#77305=CARTESIAN_POINT ( 'NONE',  ( -13.77266209894789917, 1517.151704408390060, 217.0393652727940150 ) ) ;
#77328=FACE_OUTER_BOUND ( 'NONE', #86147, .T. ) ;
#77421=CARTESIAN_POINT ( 'NONE',  ( 9.786977751178733698, 1517.051704408389924, 226.9642986345448890 ) ) ;
#77424=DIRECTION ( 'NONE',  ( 0.9455185755993178454, 0.000000000000000000, -0.3255681544571537578 ) ) ;
#77435=EDGE_CURVE ( 'NONE', #5162, #25680, #41151, .T. ) ;
#77449=CARTESIAN_POINT ( 'NONE',  ( 19.66678637246580053, 1519.551704408389924, 202.3500283489900085 ) ) ;
#77450=FACE_BOUND ( 'NONE', #32621, .T. ) ;
#77469=CARTESIAN_POINT ( 'NONE',  ( 13.13561839920526886, 1522.051704408389924, 209.9352119836111683 ) ) ;
#77472=ADVANCED_FACE ( 'NONE', ( #43601 ), #1860, .T. ) ;
#77496=ORIENTED_EDGE ( 'NONE', *, *, #24172, .T. ) ;
#77513=EDGE_CURVE ( 'NONE', #31342, #28739, #73368, .T. ) ;
#77557=DIRECTION ( 'NONE',  ( -1.755985294532469921E-16, 1.000000000000000000, -1.338183447452831989E-16 ) ) ;
#77569=VERTEX_POINT ( 'NONE', #24851 ) ;
#77570=ORIENTED_EDGE ( 'NONE', *, *, #34461, .T. ) ;
#77582=EDGE_CURVE ( 'NONE', #10167, #31573, #78722, .T. ) ;
#77623=AXIS2_PLACEMENT_3D ( 'NONE', #106381, #11241, #106921 ) ;
#77632=VERTEX_POINT ( 'NONE', #15899 ) ;
#77647=DIRECTION ( 'NONE',  ( -5.980589973904019347E-17, 1.000000000000000000, -1.736889445713099699E-16 ) ) ;
#77660=LINE ( 'NONE', #54142, #67512 ) ;
#77661=EDGE_CURVE ( 'NONE', #365, #27217, #15578, .T. ) ;
#77689=EDGE_CURVE ( 'NONE', #97374, #34577, #103201, .T. ) ;
#77691=ORIENTED_EDGE ( 'NONE', *, *, #9807, .T. ) ;
#77705=DIRECTION ( 'NONE',  ( -0.6736849260863839728, 0.000000000000000000, 0.7390186874254150995 ) ) ;
#77784=CARTESIAN_POINT ( 'NONE',  ( -3.272667022753710242, 1517.151704408390060, 189.0363362235078171 ) ) ;
#77786=CIRCLE ( 'NONE', #108145, 2.000000000000003553 ) ;
#77868=VECTOR ( 'NONE', #1552, 1000.000000000000000 ) ;
#77872=CARTESIAN_POINT ( 'NONE',  ( -9.196349486490202452, 1517.151704408390060, 203.7768694350468195 ) ) ;
#77888=CYLINDRICAL_SURFACE ( 'NONE', #43868, 1.999999999999999556 ) ;
#77928=DIRECTION ( 'NONE',  ( 0.9455185755993178454, 0.000000000000000000, -0.3255681544571537578 ) ) ;
#77943=CIRCLE ( 'NONE', #27908, 2.000000000000003553 ) ;
#77945=AXIS2_PLACEMENT_3D ( 'NONE', #104529, #80985, #72071 ) ;
#77968=CIRCLE ( 'NONE', #61941, 1.999999999999999556 ) ;
#77991=SURFACE_STYLE_FILL_AREA ( #34880 ) ;
#78041=FACE_OUTER_BOUND ( 'NONE', #44005, .T. ) ;
#78055=EDGE_CURVE ( 'NONE', #105548, #63893, #38787, .T. ) ;
#78064=AXIS2_PLACEMENT_3D ( 'NONE', #7906, #108168, #50490 ) ;
#78087=EDGE_LOOP ( 'NONE', ( #100192, #85645, #59330, #82089 ) ) ;
#78141=EDGE_CURVE ( 'NONE', #64595, #75633, #109861, .T. ) ;
#78146=EDGE_CURVE ( 'NONE', #96293, #83569, #3099, .T. ) ;
#78161=ORIENTED_EDGE ( 'NONE', *, *, #31621, .T. ) ;
#78162=DIRECTION ( 'NONE',  ( 1.755985294532469921E-16, -1.000000000000000000, 1.338183447452831989E-16 ) ) ;
#78174=ORIENTED_EDGE ( 'NONE', *, *, #72432, .F. ) ;
#78194=CIRCLE ( 'NONE', #104979, 2.000000000000003553 ) ;
#78220=DIRECTION ( 'NONE',  ( 1.755985294532464991E-16, -1.000000000000000000, 1.338183447452830017E-16 ) ) ;
#78253=AXIS2_PLACEMENT_3D ( 'NONE', #85283, #8582, #42752 ) ;
#78294=DIRECTION ( 'NONE',  ( 0.3255681544571546460, 0.000000000000000000, 0.9455185755993176233 ) ) ;
#78297=ORIENTED_EDGE ( 'NONE', *, *, #102131, .F. ) ;
#78316=CARTESIAN_POINT ( 'NONE',  ( -3.968827101022720072, 1521.951704408389787, 229.5396913742049776 ) ) ;
#78319=CYLINDRICAL_SURFACE ( 'NONE', #93665, 2.000000000000003553 ) ;
#78343=VECTOR ( 'NONE', #18911, 1000.000000000000000 ) ;
#78367=CYLINDRICAL_SURFACE ( 'NONE', #36164, 2.000000000000003109 ) ;
#78370=VERTEX_POINT ( 'NONE', #37299 ) ;
#78408=CYLINDRICAL_SURFACE ( 'NONE', #78817, 2.000000000000003553 ) ;
#78412=CARTESIAN_POINT ( 'NONE',  ( 11.78824854703250047, 1517.151704408390060, 211.4132493584619965 ) ) ;
#78443=DIRECTION ( 'NONE',  ( 1.755985294532464991E-16, -1.000000000000000000, 1.338183447452830017E-16 ) ) ;
#78444=DIRECTION ( 'NONE',  ( -0.6736849260863837507, 0.000000000000000000, 0.7390186874254154326 ) ) ;
#78459=ADVANCED_FACE ( 'NONE', ( #4248 ), #37849, .F. ) ;
#78497=AXIS2_PLACEMENT_3D ( 'NONE', #75247, #107171, #82534 ) ;
#78552=AXIS2_PLACEMENT_3D ( 'NONE', #15136, #31955, #66148 ) ;
#78563=CYLINDRICAL_SURFACE ( 'NONE', #88954, 2.000000000000003553 ) ;
#78607=AXIS2_PLACEMENT_3D ( 'NONE', #29850, #39910, #55636 ) ;
#78613=CARTESIAN_POINT ( 'NONE',  ( -18.31941652021487954, 1517.151704408390060, 214.4156261991469421 ) ) ;
#78622=EDGE_CURVE ( 'NONE', #84204, #100346, #53124, .T. ) ;
#78630=ORIENTED_EDGE ( 'NONE', *, *, #29302, .F. ) ;
#78657=CIRCLE ( 'NONE', #30368, 1.999999999999999556 ) ;
#78664=DIRECTION ( 'NONE',  ( 1.755985294532469921E-16, -1.000000000000000000, 1.338183447452831989E-16 ) ) ;
#78688=DIRECTION ( 'NONE',  ( -1.755985294532469921E-16, 1.000000000000000000, -1.338183447452831989E-16 ) ) ;
#78693=DIRECTION ( 'NONE',  ( 1.755985294532469921E-16, -1.000000000000000000, 1.338183447452831989E-16 ) ) ;
#78722=CIRCLE ( 'NONE', #71046, 1.999999999999999556 ) ;
#78743=DIRECTION ( 'NONE',  ( -0.6736849260863841948, 0.000000000000000000, 0.7390186874254148774 ) ) ;
#78760=CARTESIAN_POINT ( 'NONE',  ( 11.75869035672759999, 1519.551704408389924, 227.2994842695800060 ) ) ;
#78772=DIRECTION ( 'NONE',  ( -5.980589973904019347E-17, 1.000000000000000000, -1.736889445713099699E-16 ) ) ;
#78817=AXIS2_PLACEMENT_3D ( 'NONE', #1720, #17918, #3804 ) ;
#78829=EDGE_CURVE ( 'NONE', #41356, #86539, #78194, .T. ) ;
#78832=ADVANCED_FACE ( 'NONE', ( #34265 ), #75190, .F. ) ;
#78861=CIRCLE ( 'NONE', #93145, 2.000000000000003553 ) ;
#78879=EDGE_CURVE ( 'NONE', #64021, #69131, #88979, .T. ) ;
#78894=CARTESIAN_POINT ( 'NONE',  ( -1.925297170580940076, 1522.051704408389924, 187.5582988486569889 ) ) ;
#78904=EDGE_LOOP ( 'NONE', ( #85296, #48168, #77570, #49193, #23024 ) ) ;
#78906=AXIS2_PLACEMENT_3D ( 'NONE', #49780, #22878, #56524 ) ;
#78923=DIRECTION ( 'NONE',  ( 0.9858563016923833633, 0.000000000000000000, 0.1675928173085483863 ) ) ;
#78939=AXIS2_PLACEMENT_3D ( 'NONE', #42794, #25963, #51757 ) ;
#78947=AXIS2_PLACEMENT_3D ( 'NONE', #55927, #90047, #47521 ) ;
#78963=DIRECTION ( 'NONE',  ( 0.9455185755993178454, 0.000000000000000000, -0.3255681544571537578 ) ) ;
#78966=VERTEX_POINT ( 'NONE', #72843 ) ;
#79041=CARTESIAN_POINT ( 'NONE',  ( 16.36456115949343015, 1519.551704408389924, 198.1507535207238391 ) ) ;
#79124=ADVANCED_FACE ( 'NONE', ( #11691 ), #29050, .F. ) ;
#79136=DIRECTION ( 'NONE',  ( 0.9455185755993178454, 0.000000000000000000, -0.3255681544571539243 ) ) ;
#79179=CARTESIAN_POINT ( 'NONE',  ( 11.75869035672759999, 1517.151704408390060, 227.2994842695800060 ) ) ;
#79243=CARTESIAN_POINT ( 'NONE',  ( 8.464772015878841316, 1522.051704408389924, 233.7053289272604104 ) ) ;
#79256=CARTESIAN_POINT ( 'NONE',  ( 15.09047375999176843, 1517.051704408389924, 215.6125241866901661 ) ) ;
#79273=VERTEX_POINT ( 'NONE', #37997 ) ;
#79297=ORIENTED_EDGE ( 'NONE', *, *, #87677, .F. ) ;
#79329=DIRECTION ( 'NONE',  ( -0.9455185755993182894, 0.000000000000000000, 0.3255681544571523145 ) ) ;
#79354=CARTESIAN_POINT ( 'NONE',  ( 13.10606020890037016, 1517.151704408390060, 225.8214468947291493 ) ) ;
#79368=DIRECTION ( 'NONE',  ( -1.755985294532469921E-16, 1.000000000000000000, -1.338183447452831989E-16 ) ) ;
#79373=FACE_OUTER_BOUND ( 'NONE', #4892, .T. ) ;
#79374=ORIENTED_EDGE ( 'NONE', *, *, #58460, .F. ) ;
#79391=CIRCLE ( 'NONE', #25715, 1.999999999999999556 ) ;
#79437=DIRECTION ( 'NONE',  ( 1.755985294532464991E-16, -1.000000000000000000, 1.338183447452830017E-16 ) ) ;
#79455=EDGE_CURVE ( 'NONE', #81426, #85274, #77660, .T. ) ;
#79466=VECTOR ( 'NONE', #68402, 1000.000000000000000 ) ;
#79478=DIRECTION ( 'NONE',  ( -0.9455185755993178454, 0.000000000000000000, 0.3255681544571537578 ) ) ;
#79483=ORIENTED_EDGE ( 'NONE', *, *, #51660, .T. ) ;
#79534=DIRECTION ( 'NONE',  ( 0.9455185755993178454, 0.000000000000000000, -0.3255681544571539243 ) ) ;
#79536=CARTESIAN_POINT ( 'NONE',  ( 15.69795926444620271, 1517.151704408390060, 222.7678737639049871 ) ) ;
#79538=CARTESIAN_POINT ( 'NONE',  ( -15.69795926856320101, 1521.951704408389787, 195.4758181589010064 ) ) ;
#79544=VERTEX_POINT ( 'NONE', #8781 ) ;
#79550=VERTEX_POINT ( 'NONE', #53588 ) ;
#79604=AXIS2_PLACEMENT_3D ( 'NONE', #74019, #108154, #93541 ) ;
#79651=LINE ( 'NONE', #105390, #92268 ) ;
#79670=CARTESIAN_POINT ( 'NONE',  ( 13.73040295794826626, 1521.951704408389787, 227.6346699037790984 ) ) ;
#79748=ORIENTED_EDGE ( 'NONE', *, *, #59780, .T. ) ;
#79842=DIRECTION ( 'NONE',  ( -0.6736849260863841948, 0.000000000000000000, 0.7390186874254148774 ) ) ;
#79854=VERTEX_POINT ( 'NONE', #45145 ) ;
#79870=VERTEX_POINT ( 'NONE', #71473 ) ;
#79883=DIRECTION ( 'NONE',  ( -0.9455185755993178454, 0.000000000000000000, 0.3255681544571539243 ) ) ;
#79910=LINE ( 'NONE', #45775, #13328 ) ;
#79935=AXIS2_PLACEMENT_3D ( 'NONE', #94423, #77647, #86592 ) ;
#79973=DIRECTION ( 'NONE',  ( 5.980589973904019347E-17, -1.000000000000000000, 1.736889445713099699E-16 ) ) ;
#80044=ORIENTED_EDGE ( 'NONE', *, *, #50922, .T. ) ;
#80095=ORIENTED_EDGE ( 'NONE', *, *, #1145, .T. ) ;
#80097=ORIENTED_EDGE ( 'NONE', *, *, #37063, .F. ) ;
#80140=AXIS2_PLACEMENT_3D ( 'NONE', #74685, #16381, #66299 ) ;
#80163=VECTOR ( 'NONE', #31227, 1000.000000000000000 ) ;
#80164=EDGE_CURVE ( 'NONE', #99465, #77064, #15651, .T. ) ;
#80178=AXIS2_PLACEMENT_3D ( 'NONE', #12133, #90488, #38973 ) ;
#80189=DIRECTION ( 'NONE',  ( -0.6736849260863839728, 0.000000000000000000, 0.7390186874254150995 ) ) ;
#80212=CARTESIAN_POINT ( 'NONE',  ( -19.66678637246580053, 1521.951704408389787, 215.8936635744080093 ) ) ;
#80217=CARTESIAN_POINT ( 'NONE',  ( -1.317811661047102012, 1517.051704408389924, 194.7136484256038500 ) ) ;
#80260=EDGE_CURVE ( 'NONE', #1077, #87539, #22774, .T. ) ;
#80268=EDGE_CURVE ( 'NONE', #64955, #47444, #49998, .T. ) ;
#80289=EDGE_LOOP ( 'NONE', ( #86866, #43622, #8165, #32328, #9143 ) ) ;
#80313=CIRCLE ( 'NONE', #89255, 2.000000000000003553 ) ;
#80351=EDGE_CURVE ( 'NONE', #105626, #66063, #74698, .T. ) ;
#80363=ORIENTED_EDGE ( 'NONE', *, *, #63184, .T. ) ;
#80378=DIRECTION ( 'NONE',  ( -0.6736849260149578855, 0.000000000000000000, 0.7390186874905266823 ) ) ;
#80383=DIRECTION ( 'NONE',  ( 5.980589973904019347E-17, -1.000000000000000000, 1.736889445713099699E-16 ) ) ;
#80390=AXIS2_PLACEMENT_3D ( 'NONE', #104786, #3450, #71781 ) ;
#80452=DIRECTION ( 'NONE',  ( 0.9455185755993178454, 0.000000000000000000, -0.3255681544571537578 ) ) ;
#80453=VERTEX_POINT ( 'NONE', #10189 ) ;
#80457=ORIENTED_EDGE ( 'NONE', *, *, #87210, .T. ) ;
#80483=DIRECTION ( 'NONE',  ( -0.6736849260863839728, 0.000000000000000000, 0.7390186874254150995 ) ) ;
#80493=AXIS2_PLACEMENT_3D ( 'NONE', #36846, #71038, #12747 ) ;
#80516=EDGE_LOOP ( 'NONE', ( #27204, #63212, #3732, #91814 ) ) ;
#80535=CIRCLE ( 'NONE', #32245, 2.000000000000003553 ) ;
#80538=LINE ( 'NONE', #4386, #71795 ) ;
#80546=DIRECTION ( 'NONE',  ( -1.755985294532469921E-16, 1.000000000000000000, -1.338183447452831989E-16 ) ) ;
#80553=DIRECTION ( 'NONE',  ( 0.9858563016923833633, 0.000000000000000000, 0.1675928173085483863 ) ) ;
#80573=DIRECTION ( 'NONE',  ( 1.755985294532469921E-16, -1.000000000000000000, 1.338183447452831989E-16 ) ) ;
#80585=AXIS2_PLACEMENT_3D ( 'NONE', #15298, #50038, #99856 ) ;
#80630=ADVANCED_FACE ( 'NONE', ( #82899 ), #93493, .F. ) ;
#80631=FACE_OUTER_BOUND ( 'NONE', #55643, .T. ) ;
#80691=CIRCLE ( 'NONE', #39602, 2.000000000000002220 ) ;
#80706=DIRECTION ( 'NONE',  ( 0.9858563016923833633, 0.000000000000000000, 0.1675928173085483863 ) ) ;
#80718=DIRECTION ( 'NONE',  ( 0.9455185755993178454, 0.000000000000000000, -0.3255681544571537578 ) ) ;
#80719=DIRECTION ( 'NONE',  ( -0.9455185755993167351, 0.000000000000000000, 0.3255681544571568109 ) ) ;
#80720=ORIENTED_EDGE ( 'NONE', *, *, #61302, .T. ) ;
#80787=DIRECTION ( 'NONE',  ( -1.755985294532469921E-16, 1.000000000000000000, -1.338183447452831989E-16 ) ) ;
#80793=DIRECTION ( 'NONE',  ( -0.9455185755993166241, 1.675808339056839216E-14, 0.3255681544571569219 ) ) ;
#80863=AXIS2_PLACEMENT_3D ( 'NONE', #38389, #5345, #31091 ) ;
#80889=ORIENTED_EDGE ( 'NONE', *, *, #82339, .F. ) ;
#80982=ADVANCED_FACE ( 'NONE', ( #73276 ), #46443, .F. ) ;
#80985=DIRECTION ( 'NONE',  ( -5.980589973904019347E-17, 1.000000000000000000, -1.736889445713099699E-16 ) ) ;
#81112=ORIENTED_EDGE ( 'NONE', *, *, #27754, .T. ) ;
#81119=ORIENTED_EDGE ( 'NONE', *, *, #34965, .F. ) ;
#81124=CARTESIAN_POINT ( 'NONE',  ( -23.59335433665016524, 1521.951704408389787, 209.8811657366738928 ) ) ;
#81129=EDGE_CURVE ( 'NONE', #81525, #32285, #96188, .T. ) ;
#81132=AXIS2_PLACEMENT_3D ( 'NONE', #88923, #12209, #105183 ) ;
#81148=CIRCLE ( 'NONE', #104420, 1.999999999999998668 ) ;
#81180=DIRECTION ( 'NONE',  ( -0.6736849260863839728, 0.000000000000000000, 0.7390186874254150995 ) ) ;
#81195=CARTESIAN_POINT ( 'NONE',  ( 3.968827103902559550, 1522.051704408389924, 188.7040005461919918 ) ) ;
#81262=FACE_OUTER_BOUND ( 'NONE', #70202, .T. ) ;
#81269=DIRECTION ( 'NONE',  ( -1.755985294532469921E-16, 1.000000000000000000, -1.338183447452831989E-16 ) ) ;
#81280=AXIS2_PLACEMENT_3D ( 'NONE', #82164, #74350, #64296 ) ;
#81285=AXIS2_PLACEMENT_3D ( 'NONE', #10457, #78772, #79883 ) ;
#81291=ORIENTED_EDGE ( 'NONE', *, *, #61639, .F. ) ;
#81293=ORIENTED_EDGE ( 'NONE', *, *, #40526, .F. ) ;
#81317=DIRECTION ( 'NONE',  ( -5.980589973904019347E-17, 1.000000000000000000, -1.736889445713099699E-16 ) ) ;
#81318=AXIS2_PLACEMENT_3D ( 'NONE', #89284, #63034, #12029 ) ;
#81324=ORIENTED_EDGE ( 'NONE', *, *, #26072, .F. ) ;
#81342=CYLINDRICAL_SURFACE ( 'NONE', #74839, 2.000000000000003553 ) ;
#81355=DIRECTION ( 'NONE',  ( -0.6736849260863841948, 0.000000000000000000, 0.7390186874254148774 ) ) ;
#81391=VERTEX_POINT ( 'NONE', #77421 ) ;
#81426=VERTEX_POINT ( 'NONE', #58561 ) ;
#81434=DIRECTION ( 'NONE',  ( -0.6736849260863841948, 0.000000000000000000, 0.7390186874254148774 ) ) ;
#81449=ADVANCED_FACE ( 'NONE', ( #88589 ), #53911, .F. ) ;
#81488=ORIENTED_EDGE ( 'NONE', *, *, #5135, .T. ) ;
#81525=VERTEX_POINT ( 'NONE', #22995 ) ;
#81532=CARTESIAN_POINT ( 'NONE',  ( 17.69507376876702764, 1517.051704408389924, 202.0148427140983358 ) ) ;
#81538=CYLINDRICAL_SURFACE ( 'NONE', #8775, 1.999999999999999556 ) ;
#81557=CARTESIAN_POINT ( 'NONE',  ( -6.647330431358690284, 1517.051704408389924, 184.4413780136169976 ) ) ;
#81582=CARTESIAN_POINT ( 'NONE',  ( -10.02843955878900140, 1522.051704408389924, 185.3723613107750054 ) ) ;
#81601=VERTEX_POINT ( 'NONE', #73299 ) ;
#81603=EDGE_LOOP ( 'NONE', ( #26803, #27821 ) ) ;
#81623=DIRECTION ( 'NONE',  ( -1.755985294532469921E-16, 1.000000000000000000, -1.338183447452831989E-16 ) ) ;
#81655=CARTESIAN_POINT ( 'NONE',  ( 9.225907677606098645, 1517.051704408389924, 198.5805875773771731 ) ) ;
#81668=CARTESIAN_POINT ( 'NONE',  ( 15.69795926444620271, 1519.551704408389924, 222.7678737639049871 ) ) ;
#81723=CARTESIAN_POINT ( 'NONE',  ( -3.968827103576990201, 1522.051704408389924, 229.5396913781519856 ) ) ;
#81732=ORIENTED_EDGE ( 'NONE', *, *, #21536, .T. ) ;
#81733=ORIENTED_EDGE ( 'NONE', *, *, #38623, .T. ) ;
#81755=AXIS2_PLACEMENT_3D ( 'NONE', #91187, #7191, #49207 ) ;
#81762=ORIENTED_EDGE ( 'NONE', *, *, #30221, .F. ) ;
#81785=LINE ( 'NONE', #107551, #95791 ) ;
#81836=AXIS2_PLACEMENT_3D ( 'NONE', #46616, #104291, #53926 ) ;
#81848=EDGE_CURVE ( 'NONE', #66063, #105626, #105143, .T. ) ;
#81877=DIRECTION ( 'NONE',  ( -0.6736849260863839728, 0.000000000000000000, 0.7390186874254150995 ) ) ;
#81882=EDGE_LOOP ( 'NONE', ( #21948, #41710 ) ) ;
#81902=EDGE_CURVE ( 'NONE', #65447, #43851, #89063, .T. ) ;
#81909=DIRECTION ( 'NONE',  ( 1.755985294532464991E-16, -1.000000000000000000, 1.338183447452830017E-16 ) ) ;
#81929=CARTESIAN_POINT ( 'NONE',  ( 1.984413551915469975, 1517.051704408389924, 198.9129232538419956 ) ) ;
#81939=DIRECTION ( 'NONE',  ( -0.9455185755993178454, 0.000000000000000000, 0.3255681544571537578 ) ) ;
#81942=CARTESIAN_POINT ( 'NONE',  ( -17.71193100849139768, 1519.551704408389924, 221.5709757781449980 ) ) ;
#81944=LINE ( 'NONE', #14186, #71543 ) ;
#81954=CARTESIAN_POINT ( 'NONE',  ( 21.62164173326539895, 1519.551704408389924, 208.0273405521070060 ) ) ;
#81964=FACE_BOUND ( 'NONE', #50428, .T. ) ;
#81969=ORIENTED_EDGE ( 'NONE', *, *, #105576, .F. ) ;
#81974=CARTESIAN_POINT ( 'NONE',  ( -10.26338073471560008, 1519.551704408389924, 184.6900425920350131 ) ) ;
#81975=CARTESIAN_POINT ( 'NONE',  ( -19.66678637246580053, 1517.051704408389924, 215.8936635744080093 ) ) ;
#81981=( LENGTH_UNIT ( ) NAMED_UNIT ( * ) SI_UNIT ( .MILLI., .METRE. ) );
#82004=CIRCLE ( 'NONE', #55262, 1.999999999999999556 ) ;
#82070=VECTOR ( 'NONE', #65299, 1000.000000000000000 ) ;
#82085=ORIENTED_EDGE ( 'NONE', *, *, #34316, .F. ) ;
#82087=EDGE_CURVE ( 'NONE', #20697, #37122, #101591, .T. ) ;
#82089=ORIENTED_EDGE ( 'NONE', *, *, #63343, .T. ) ;
#82164=CARTESIAN_POINT ( 'NONE',  ( 9.833393186232889605, 1517.151704408390060, 205.7359371553449989 ) ) ;
#82177=ADVANCED_FACE ( 'NONE', ( #108416, #65882, #14889, #40104, #66983, #31700, #100003, #23836, #74831, #23291, #50185, #108974, #41757, #31148, #49628, #83215, #66440, #100556, #109523, #92163, #75386, #7059, #15436, #101094, #24393, #92706, #15983, #84311, #7603, #75916, #33344, #67539, #93260, #16524, #65336, #22721, #77032, #61906, #886, #59680, #70313, #10926, #94349, #68096, #9811, #9269, #19295, #26603, #95477, #96024 ), #52938, .F. ) ;
#82202=CARTESIAN_POINT ( 'NONE',  ( -5.864566082395450408, 1517.151704408390060, 192.0899093523580063 ) ) ;
#82286=ORIENTED_EDGE ( 'NONE', *, *, #20296, .F. ) ;
#82291=DIRECTION ( 'NONE',  ( 0.9455185755993178454, 0.000000000000000000, -0.3255681544571537578 ) ) ;
#82294=LINE ( 'NONE', #97979, #63628 ) ;
#82303=AXIS2_PLACEMENT_3D ( 'NONE', #88524, #56572, #45978 ) ;
#82338=MANIFOLD_SOLID_BREP ( 'Stock-MAS-682-1', #5599 ) ;
#82339=EDGE_CURVE ( 'NONE', #78966, #365, #56954, .T. ) ;
#82428=AXIS2_PLACEMENT_3D ( 'NONE', #60335, #102307, #85499 ) ;
#82445=VERTEX_POINT ( 'NONE', #100160 ) ;
#82487=ORIENTED_EDGE ( 'NONE', *, *, #74901, .F. ) ;
#82512=CARTESIAN_POINT ( 'NONE',  ( 22.96901158543816734, 1522.051704408389924, 206.5493031772561778 ) ) ;
#82518=EDGE_CURVE ( 'NONE', #66989, #43462, #103457, .T. ) ;
#82529=CIRCLE ( 'NONE', #34244, 2.000000000000003553 ) ;
#82534=DIRECTION ( 'NONE',  ( -0.9455185755993178454, 0.000000000000000000, 0.3255681544571537578 ) ) ;
#82543=ADVANCED_FACE ( 'NONE', ( #51982 ), #44694, .F. ) ;
#82547=ORIENTED_EDGE ( 'NONE', *, *, #42389, .T. ) ;
#82628=CARTESIAN_POINT ( 'NONE',  ( -21.01415622427471774, 1522.051704408389924, 217.3717009491090835 ) ) ;
#82696=CARTESIAN_POINT ( 'NONE',  ( 3.968827103902559550, 1519.551704408389924, 188.7040005461919918 ) ) ;
#82757=DIRECTION ( 'NONE',  ( 1.755985294532464991E-16, -1.000000000000000000, 1.338183447452830017E-16 ) ) ;
#82777=VERTEX_POINT ( 'NONE', #54625 ) ;
#82827=EDGE_LOOP ( 'NONE', ( #102386, #5096, #18448, #44935, #77095 ) ) ;
#82833=CARTESIAN_POINT ( 'NONE',  ( 8.627556093114659319, 1519.551704408389924, 234.1780882150808907 ) ) ;
#82836=ORIENTED_EDGE ( 'NONE', *, *, #5486, .F. ) ;
#82899=FACE_OUTER_BOUND ( 'NONE', #95046, .T. ) ;
#82902=DIRECTION ( 'NONE',  ( -0.6736849260863841948, 0.000000000000000000, 0.7390186874254148774 ) ) ;
#82920=EDGE_LOOP ( 'NONE', ( #29690, #107498, #26162, #31460, #42501 ) ) ;
#82984=EDGE_CURVE ( 'NONE', #56110, #31476, #94482, .T. ) ;
#83008=CARTESIAN_POINT ( 'NONE',  ( 13.72624666550403560, 1521.951704408389787, 222.4326881308259090 ) ) ;
#83011=ORIENTED_EDGE ( 'NONE', *, *, #55884, .F. ) ;
#83048=DIRECTION ( 'NONE',  ( -0.3255681544571569219, -1.836970198721028948E-16, -0.9455185755993167351 ) ) ;
#83050=VECTOR ( 'NONE', #110251, 1000.000000000000000 ) ;
#83060=CARTESIAN_POINT ( 'NONE',  ( -9.862951377749247683, 1517.151704408390060, 228.3939896778649654 ) ) ;
#83081=CARTESIAN_POINT ( 'NONE',  ( -15.74021840828143404, 1521.951704408389787, 221.9061614121420973 ) ) ;
#83112=ORIENTED_EDGE ( 'NONE', *, *, #61306, .F. ) ;
#83130=ADVANCED_FACE ( 'NONE', ( #80631 ), #28572, .F. ) ;
#83211=FACE_OUTER_BOUND ( 'NONE', #20282, .T. ) ;
#83215=FACE_BOUND ( 'NONE', #31503, .T. ) ;
#83249=EDGE_CURVE ( 'NONE', #108494, #98226, #67741, .T. ) ;
#83271=VERTEX_POINT ( 'NONE', #95094 ) ;
#83292=AXIS2_PLACEMENT_3D ( 'NONE', #61829, #37150, #53987 ) ;
#83298=FACE_OUTER_BOUND ( 'NONE', #48749, .T. ) ;
#83316=AXIS2_PLACEMENT_3D ( 'NONE', #8804, #68755, #77144 ) ;
#83328=CARTESIAN_POINT ( 'NONE',  ( -11.18076303840567043, 1517.151704408390060, 213.9857921429048417 ) ) ;
#83338=CARTESIAN_POINT ( 'NONE',  ( 3.909710721586129534, 1517.151704408390060, 220.4764703678949900 ) ) ;
#83352=DIRECTION ( 'NONE',  ( -0.9455185755993178454, 0.000000000000000000, 0.3255681544571539243 ) ) ;
#83356=DIRECTION ( 'NONE',  ( 5.980589973904019347E-17, -1.000000000000000000, 1.736889445713099699E-16 ) ) ;
#83363=DIRECTION ( 'NONE',  ( -0.9455185755993178454, 0.000000000000000000, 0.3255681544571539243 ) ) ;
#83367=CARTESIAN_POINT ( 'NONE',  ( -3.968827101022720072, 1517.051704408389924, 229.5396913742049776 ) ) ;
#83369=ORIENTED_EDGE ( 'NONE', *, *, #72631, .T. ) ;
#83384=AXIS2_PLACEMENT_3D ( 'NONE', #83804, #58619, #66489 ) ;
#83451=LINE ( 'NONE', #65580, #90323 ) ;
#83469=ADVANCED_FACE ( 'NONE', ( #26216 ), #16692, .F. ) ;
#83489=EDGE_LOOP ( 'NONE', ( #6541, #98113, #63550, #40202 ) ) ;
#83508=DIRECTION ( 'NONE',  ( -0.6736849260863839728, 0.000000000000000000, 0.7390186874254150995 ) ) ;
#83518=VECTOR ( 'NONE', #11057, 1000.000000000000000 ) ;
#83529=DIRECTION ( 'NONE',  ( -0.9455185755993166241, 1.675808339056839216E-14, 0.3255681544571569219 ) ) ;
#83531=ORIENTED_EDGE ( 'NONE', *, *, #33330, .F. ) ;
#83536=CARTESIAN_POINT ( 'NONE',  ( 11.18076303840565799, 1517.051704408389924, 204.2578997804941707 ) ) ;
#83569=VERTEX_POINT ( 'NONE', #29536 ) ;
#83577=CARTESIAN_POINT ( 'NONE',  ( 9.196349486490200675, 1522.051704408389924, 214.4668224883511698 ) ) ;
#83620=AXIS2_PLACEMENT_3D ( 'NONE', #37021, #61706, #77928 ) ;
#83653=ORIENTED_EDGE ( 'NONE', *, *, #54269, .T. ) ;
#83674=CARTESIAN_POINT ( 'NONE',  ( 19.66678637246580053, 1519.551704408389924, 202.3500283489900085 ) ) ;
#83680=AXIS2_PLACEMENT_3D ( 'NONE', #13069, #71398, #2526 ) ;
#83686=DIRECTION ( 'NONE',  ( -5.980589973904019347E-17, 1.000000000000000000, -1.736889445713099699E-16 ) ) ;
#83722=DIRECTION ( 'NONE',  ( -1.755985294532469921E-16, 1.000000000000000000, -1.338183447452831989E-16 ) ) ;
#83731=AXIS2_PLACEMENT_3D ( 'NONE', #47970, #31155, #56380 ) ;
#83749=EDGE_LOOP ( 'NONE', ( #21119, #73507 ) ) ;
#83797=ORIENTED_EDGE ( 'NONE', *, *, #92251, .T. ) ;
#83804=CARTESIAN_POINT ( 'NONE',  ( -19.63722818156799832, 1519.551704408389924, 200.0074286628000095 ) ) ;
#83828=DIRECTION ( 'NONE',  ( -0.9455185755993178454, 0.000000000000000000, 0.3255681544571537578 ) ) ;
#83848=DIRECTION ( 'NONE',  ( 1.755985294532464991E-16, -1.000000000000000000, 1.338183447452830017E-16 ) ) ;
#83850=DIRECTION ( 'NONE',  ( -5.980589973904019347E-17, 1.000000000000000000, -1.736889445713099699E-16 ) ) ;
#83895=ORIENTED_EDGE ( 'NONE', *, *, #33180, .T. ) ;
#84015=CARTESIAN_POINT ( 'NONE',  ( 11.78824854703250047, 1517.051704408389924, 211.4132493584619965 ) ) ;
#84047=ORIENTED_EDGE ( 'NONE', *, *, #85030, .T. ) ;
#84090=CARTESIAN_POINT ( 'NONE',  ( 19.64992912941728420, 1519.551704408389924, 207.6921549202155290 ) ) ;
#84124=ORIENTED_EDGE ( 'NONE', *, *, #15619, .T. ) ;
#84150=VECTOR ( 'NONE', #31044, 1000.000000000000000 ) ;
#84158=FACE_OUTER_BOUND ( 'NONE', #90239, .T. ) ;
#84163=CARTESIAN_POINT ( 'NONE',  ( 20.27427188109263412, 1522.051704408389924, 209.5053779269578342 ) ) ;
#84177=FACE_BOUND ( 'NONE', #106323, .T. ) ;
#84202=ORIENTED_EDGE ( 'NONE', *, *, #50162, .F. ) ;
#84204=VERTEX_POINT ( 'NONE', #64013 ) ;
#84226=CARTESIAN_POINT ( 'NONE',  ( -9.833393186232900263, 1522.051704408389924, 212.5077547680540135 ) ) ;
#84235=EDGE_CURVE ( 'NONE', #108856, #58309, #42712, .T. ) ;
#84237=ADVANCED_FACE ( 'NONE', ( #10402 ), #44572, .F. ) ;
#84247=EDGE_CURVE ( 'NONE', #53816, #88646, #8724, .T. ) ;
#84296=ORIENTED_EDGE ( 'NONE', *, *, #69383, .F. ) ;
#84311=FACE_BOUND ( 'NONE', #95593, .T. ) ;
#84365=VECTOR ( 'NONE', #40741, 1000.000000000000000 ) ;
#84439=DIRECTION ( 'NONE',  ( -5.980589973904019347E-17, 1.000000000000000000, -1.736889445713099699E-16 ) ) ;
#84491=ORIENTED_EDGE ( 'NONE', *, *, #37919, .F. ) ;
#84539=CARTESIAN_POINT ( 'NONE',  ( 9.862951377358559313, 1519.551704408389924, 189.8497022443989977 ) ) ;
#84572=ORIENTED_EDGE ( 'NONE', *, *, #32610, .F. ) ;
#84647=CARTESIAN_POINT ( 'NONE',  ( -7.891238773387773797, 1521.951704408389787, 228.7291753153190825 ) ) ;
#84723=FACE_BOUND ( 'NONE', #101044, .T. ) ;
#84769=ORIENTED_EDGE ( 'NONE', *, *, #77513, .T. ) ;
#84771=DIRECTION ( 'NONE',  ( 1.755985294532469921E-16, -1.000000000000000000, 1.338183447452831989E-16 ) ) ;
#84779=ADVANCED_FACE ( 'NONE', ( #90421 ), #64161, .F. ) ;
#84814=VERTEX_POINT ( 'NONE', #47887 ) ;
#84816=FACE_OUTER_BOUND ( 'NONE', #41202, .T. ) ;
#84896=EDGE_CURVE ( 'NONE', #43055, #64021, #92633, .T. ) ;
#84904=CARTESIAN_POINT ( 'NONE',  ( -21.60894078472486868, 1521.951704408389787, 199.6722430288449175 ) ) ;
#84907=ORIENTED_EDGE ( 'NONE', *, *, #87021, .T. ) ;
#84931=UNCERTAINTY_MEASURE_WITH_UNIT (LENGTH_MEASURE( 1.000000000000000082E-05 ), #81981, 'distance_accuracy_value', 'NONE');
#84932=LINE ( 'NONE', #100099, #84365 ) ;
#84933=DIRECTION ( 'NONE',  ( -0.6736849260863841948, 0.000000000000000000, 0.7390186874254148774 ) ) ;
#84944=ORIENTED_EDGE ( 'NONE', *, *, #90350, .F. ) ;
#84990=ADVANCED_FACE ( 'NONE', ( #104918 ), #38248, .F. ) ;
#85030=EDGE_CURVE ( 'NONE', #109826, #79273, #95686, .T. ) ;
#85087=DIRECTION ( 'NONE',  ( 1.755985294532469921E-16, -1.000000000000000000, 1.338183447452831989E-16 ) ) ;
#85100=CARTESIAN_POINT ( 'NONE',  ( 23.59335433453006559, 1517.051704408389924, 208.3625261891680793 ) ) ;
#85104=ORIENTED_EDGE ( 'NONE', *, *, #14108, .T. ) ;
#85108=EDGE_CURVE ( 'NONE', #31779, #63901, #73241, .T. ) ;
#85127=FACE_OUTER_BOUND ( 'NONE', #40449, .T. ) ;
#85184=EDGE_LOOP ( 'NONE', ( #17072, #75119, #99010, #67336 ) ) ;
#85187=ORIENTED_EDGE ( 'NONE', *, *, #18261, .T. ) ;
#85190=DIRECTION ( 'NONE',  ( 1.755985294532464991E-16, -1.000000000000000000, 1.338183447452830017E-16 ) ) ;
#85194=DIRECTION ( 'NONE',  ( 1.755985294532464991E-16, -1.000000000000000000, 1.338183447452830017E-16 ) ) ;
#85229=DIRECTION ( 'NONE',  ( -1.755985294532469921E-16, 1.000000000000000000, -1.338183447452831989E-16 ) ) ;
#85257=CIRCLE ( 'NONE', #79935, 1.999999999999998668 ) ;
#85270=FACE_BOUND ( 'NONE', #49251, .T. ) ;
#85274=VERTEX_POINT ( 'NONE', #25507 ) ;
#85279=EDGE_LOOP ( 'NONE', ( #93593, #50738, #101409, #79374, #90831 ) ) ;
#85283=CARTESIAN_POINT ( 'NONE',  ( -11.75869035857540013, 1522.051704408389924, 190.9442076533970010 ) ) ;
#85296=ORIENTED_EDGE ( 'NONE', *, *, #37848, .T. ) ;
#85297=ORIENTED_EDGE ( 'NONE', *, *, #77435, .F. ) ;
#85301=AXIS2_PLACEMENT_3D ( 'NONE', #87711, #97743, #78743 ) ;
#85311=ORIENTED_EDGE ( 'NONE', *, *, #50403, .F. ) ;
#85343=CARTESIAN_POINT ( 'NONE',  ( -0.02955819112566620069, 1517.051704408389924, 225.0080808726450243 ) ) ;
#85347=ORIENTED_EDGE ( 'NONE', *, *, #75456, .F. ) ;
#85351=AXIS2_PLACEMENT_3D ( 'NONE', #76588, #110739, #16644 ) ;
#85385=EDGE_LOOP ( 'NONE', ( #90950, #35677, #104451, #82085, #99914 ) ) ;
#85403=EDGE_CURVE ( 'NONE', #13291, #43055, #39258, .T. ) ;
#85440=ORIENTED_EDGE ( 'NONE', *, *, #72432, .T. ) ;
#85446=AXIS2_PLACEMENT_3D ( 'NONE', #64235, #19997, #63691 ) ;
#85466=AXIS2_PLACEMENT_3D ( 'NONE', #32803, #110072, #58582 ) ;
#85491=ORIENTED_EDGE ( 'NONE', *, *, #20683, .F. ) ;
#85495=CARTESIAN_POINT ( 'NONE',  ( 11.75869035672759999, 1519.551704408389924, 227.2994842695800060 ) ) ;
#85497=CIRCLE ( 'NONE', #74827, 1.999999999999999556 ) ;
#85499=DIRECTION ( 'NONE',  ( -0.9455185755993178454, 0.000000000000000000, 0.3255681544571537578 ) ) ;
#85543=EDGE_CURVE ( 'NONE', #78370, #87307, #105379, .T. ) ;
#85551=CYLINDRICAL_SURFACE ( 'NONE', #105665, 1.999999999999999556 ) ;
#85581=AXIS2_PLACEMENT_3D ( 'NONE', #59666, #33886, #25473 ) ;
#85592=VERTEX_POINT ( 'NONE', #109091 ) ;
#85641=ADVANCED_FACE ( 'NONE', ( #86625 ), #42983, .F. ) ;
#85645=ORIENTED_EDGE ( 'NONE', *, *, #2971, .T. ) ;
#85660=DIRECTION ( 'NONE',  ( -5.980589973904019347E-17, 1.000000000000000000, -1.736889445713099699E-16 ) ) ;
#85673=EDGE_LOOP ( 'NONE', ( #83653, #46549 ) ) ;
#85686=DIRECTION ( 'NONE',  ( -5.980589973904019347E-17, 1.000000000000000000, -1.736889445713099699E-16 ) ) ;
#85690=AXIS2_PLACEMENT_3D ( 'NONE', #62143, #2241, #79478 ) ;
#85696=ORIENTED_EDGE ( 'NONE', *, *, #98574, .T. ) ;
#85736=CIRCLE ( 'NONE', #64343, 1.999999999999999556 ) ;
#85739=ORIENTED_EDGE ( 'NONE', *, *, #58216, .T. ) ;
#85745=VECTOR ( 'NONE', #11770, 1000.000000000000000 ) ;
#85793=AXIS2_PLACEMENT_3D ( 'NONE', #102313, #86079, #25600 ) ;
#85840=AXIS2_PLACEMENT_3D ( 'NONE', #107979, #31276, #90069 ) ;
#85845=ORIENTED_EDGE ( 'NONE', *, *, #9926, .F. ) ;
#85891=CYLINDRICAL_SURFACE ( 'NONE', #27028, 2.000000000000001332 ) ;
#85921=AXIS2_PLACEMENT_3D ( 'NONE', #45127, #35590, #63053 ) ;
#85958=CARTESIAN_POINT ( 'NONE',  ( 19.63722818192610120, 1519.551704408389924, 218.2362632616380154 ) ) ;
#85979=DIRECTION ( 'NONE',  ( 0.9455185755993178454, 0.000000000000000000, -0.3255681544571537578 ) ) ;
#86048=DIRECTION ( 'NONE',  ( -0.6736849260863841948, 0.000000000000000000, 0.7390186874254148774 ) ) ;
#86051=CARTESIAN_POINT ( 'NONE',  ( 9.803834995107230554, 1517.151704408390060, 221.6221720662910002 ) ) ;
#86071=DIRECTION ( 'NONE',  ( 0.9455185755993178454, 0.000000000000000000, -0.3255681544571537578 ) ) ;
#86079=DIRECTION ( 'NONE',  ( 1.755985294532464991E-16, -1.000000000000000000, 1.338183447452830017E-16 ) ) ;
#86099=LINE ( 'NONE', #44670, #83518 ) ;
#86123=CARTESIAN_POINT ( 'NONE',  ( -5.864566082395450408, 1517.151704408390060, 192.0899093523580063 ) ) ;
#86130=VECTOR ( 'NONE', #32746, 1000.000000000000000 ) ;
#86132=VERTEX_POINT ( 'NONE', #33746 ) ;
#86147=EDGE_LOOP ( 'NONE', ( #87241, #62636, #39123, #103646 ) ) ;
#86179=DIRECTION ( 'NONE',  ( -1.755985294532469921E-16, 1.000000000000000000, -1.338183447452831989E-16 ) ) ;
#86198=AXIS2_PLACEMENT_3D ( 'NONE', #62814, #4521, #46538 ) ;
#86231=VERTEX_POINT ( 'NONE', #93641 ) ;
#86232=CARTESIAN_POINT ( 'NONE',  ( 5.864566082395450408, 1522.051704408389924, 226.1537825710409777 ) ) ;
#86242=CARTESIAN_POINT ( 'NONE',  ( -11.81780673814840021, 1517.051704408389924, 222.7166774759110126 ) ) ;
#86274=ORIENTED_EDGE ( 'NONE', *, *, #110461, .F. ) ;
#86280=DIRECTION ( 'NONE',  ( 5.980589973904019347E-17, -1.000000000000000000, 1.736889445713099699E-16 ) ) ;
#86321=ORIENTED_EDGE ( 'NONE', *, *, #238, .F. ) ;
#86339=CARTESIAN_POINT ( 'NONE',  ( 19.66678637211940028, 1521.951704408389787, 202.3500283489059939 ) ) ;
#86367=CARTESIAN_POINT ( 'NONE',  ( -11.21032122992201607, 1522.051704408389924, 229.8720270527158220 ) ) ;
#86388=FACE_BOUND ( 'NONE', #20258, .T. ) ;
#86424=EDGE_CURVE ( 'NONE', #103193, #106306, #51828, .T. ) ;
#86431=VERTEX_POINT ( 'NONE', #53208 ) ;
#86443=DIRECTION ( 'NONE',  ( -0.6736849260863840838, 0.000000000000000000, 0.7390186874254150995 ) ) ;
#86500=ORIENTED_EDGE ( 'NONE', *, *, #3139, .T. ) ;
#86503=DIRECTION ( 'NONE',  ( -0.6736849260863841948, 0.000000000000000000, 0.7390186874254148774 ) ) ;
#86539=VERTEX_POINT ( 'NONE', #7055 ) ;
#86540=DIRECTION ( 'NONE',  ( 5.980589973904019347E-17, -1.000000000000000000, 1.736889445713099699E-16 ) ) ;
#86581=EDGE_LOOP ( 'NONE', ( #37544, #87916, #59576, #102343, #13941 ) ) ;
#86592=DIRECTION ( 'NONE',  ( -0.9455185755993178454, 0.000000000000000000, 0.3255681544571539243 ) ) ;
#86611=DIRECTION ( 'NONE',  ( 5.980589973904019347E-17, -1.000000000000000000, 1.736889445713099699E-16 ) ) ;
#86625=FACE_OUTER_BOUND ( 'NONE', #6458, .T. ) ;
#86629=VERTEX_POINT ( 'NONE', #108971 ) ;
#86636=LINE ( 'NONE', #103423, #77868 ) ;
#86660=DIRECTION ( 'NONE',  ( -1.755985294532469921E-16, 1.000000000000000000, -1.338183447452831989E-16 ) ) ;
#86720=DIRECTION ( 'NONE',  ( 0.9455185755993178454, 0.000000000000000000, -0.3255681544571539243 ) ) ;
#86724=AXIS2_PLACEMENT_3D ( 'NONE', #96899, #78443, #88495 ) ;
#86742=DIRECTION ( 'NONE',  ( 1.755985294532469921E-16, -1.000000000000000000, 1.338183447452831989E-16 ) ) ;
#86752=DIRECTION ( 'NONE',  ( 1.755985294532469921E-16, -1.000000000000000000, 1.338183447452831989E-16 ) ) ;
#86759=AXIS2_PLACEMENT_3D ( 'NONE', #74383, #82757, #23929 ) ;
#86807=EDGE_LOOP ( 'NONE', ( #88644, #48992, #7079, #80097 ) ) ;
#86825=ORIENTED_EDGE ( 'NONE', *, *, #107894, .T. ) ;
#86861=CARTESIAN_POINT ( 'NONE',  ( -20.98459803374077026, 1517.151704408390060, 201.4854660376508377 ) ) ;
#86864=DIRECTION ( 'NONE',  ( -0.6736849260863841948, 0.000000000000000000, 0.7390186874254148774 ) ) ;
#86866=ORIENTED_EDGE ( 'NONE', *, *, #103365, .F. ) ;
#86891=AXIS2_PLACEMENT_3D ( 'NONE', #36428, #70621, #78444 ) ;
#86894=EDGE_CURVE ( 'NONE', #79854, #101117, #68581, .T. ) ;
#86941=( LENGTH_UNIT ( ) NAMED_UNIT ( * ) SI_UNIT ( .MILLI., .METRE. ) );
#86953=FACE_OUTER_BOUND ( 'NONE', #53203, .T. ) ;
#86964=EDGE_LOOP ( 'NONE', ( #18217, #34219, #103134, #42954 ) ) ;
#86983=VERTEX_POINT ( 'NONE', #51776 ) ;
#87002=FACE_OUTER_BOUND ( 'NONE', #29670, .T. ) ;
#87008=EDGE_LOOP ( 'NONE', ( #90772, #7886 ) ) ;
#87021=EDGE_CURVE ( 'NONE', #90277, #8406, #64381, .T. ) ;
#87027=DIRECTION ( 'NONE',  ( 0.9858563016923833633, 0.000000000000000000, 0.1675928173085483863 ) ) ;
#87036=CARTESIAN_POINT ( 'NONE',  ( -7.891238774805787060, 1519.551704408389924, 228.7291753150780380 ) ) ;
#87098=ORIENTED_EDGE ( 'NONE', *, *, #27274, .T. ) ;
#87119=DIRECTION ( 'NONE',  ( -0.9455185755993178454, 0.000000000000000000, 0.3255681544571539243 ) ) ;
#87124=ADVANCED_FACE ( 'NONE', ( #57025 ), #49720, .F. ) ;
#87128=CIRCLE ( 'NONE', #63896, 1.999999999999999556 ) ;
#87148=DIRECTION ( 'NONE',  ( 0.9455185755993178454, 0.000000000000000000, -0.3255681544571537578 ) ) ;
#87153=EDGE_LOOP ( 'NONE', ( #7326, #37051 ) ) ;
#87155=CARTESIAN_POINT ( 'NONE',  ( 12.39573405564623165, 1517.051704408389924, 218.5685989363918225 ) ) ;
#87160=DIRECTION ( 'NONE',  ( -0.9455185755993178454, 0.000000000000000000, 0.3255681544571537578 ) ) ;
#87162=DIRECTION ( 'NONE',  ( 0.9455185755993178454, 0.000000000000000000, -0.3255681544571539243 ) ) ;
#87169=DIRECTION ( 'NONE',  ( 0.9455185755993178454, 0.000000000000000000, -0.3255681544571537578 ) ) ;
#87177=AXIS2_PLACEMENT_3D ( 'NONE', #7845, #17322, #67233 ) ;
#87182=CYLINDRICAL_SURFACE ( 'NONE', #43740, 1.999999999999999556 ) ;
#87189=FACE_OUTER_BOUND ( 'NONE', #451, .T. ) ;
#87195=ORIENTED_EDGE ( 'NONE', *, *, #87677, .T. ) ;
#87210=EDGE_CURVE ( 'NONE', #17997, #91497, #18838, .T. ) ;
#87241=ORIENTED_EDGE ( 'NONE', *, *, #109148, .F. ) ;
#87249=ORIENTED_EDGE ( 'NONE', *, *, #33087, .T. ) ;
#87286=FACE_OUTER_BOUND ( 'NONE', #68957, .T. ) ;
#87301=DIRECTION ( 'NONE',  ( 1.755985294532469921E-16, -1.000000000000000000, 1.338183447452831989E-16 ) ) ;
#87307=VERTEX_POINT ( 'NONE', #107827 ) ;
#87321=DIRECTION ( 'NONE',  ( -0.6736849260863841948, 0.000000000000000000, 0.7390186874254148774 ) ) ;
#87348=DIRECTION ( 'NONE',  ( 0.9455185755993178454, 0.000000000000000000, -0.3255681544571539243 ) ) ;
#87385=DIRECTION ( 'NONE',  ( 5.980589973904019347E-17, -1.000000000000000000, 1.736889445713099699E-16 ) ) ;
#87399=CYLINDRICAL_SURFACE ( 'NONE', #86891, 2.000000000000002220 ) ;
#87405=EDGE_LOOP ( 'NONE', ( #35504, #38190 ) ) ;
#87424=CYLINDRICAL_SURFACE ( 'NONE', #74406, 2.000000000000003553 ) ;
#87428=ORIENTED_EDGE ( 'NONE', *, *, #13471, .F. ) ;
#87438=ORIENTED_EDGE ( 'NONE', *, *, #6690, .F. ) ;
#87510=( NAMED_UNIT ( * ) SI_UNIT ( $, .STERADIAN. ) SOLID_ANGLE_UNIT ( ) );
#87539=VERTEX_POINT ( 'NONE', #29331 ) ;
#87541=ORIENTED_EDGE ( 'NONE', *, *, #10525, .F. ) ;
#87544=FACE_OUTER_BOUND ( 'NONE', #82827, .T. ) ;
#87551=AXIS2_PLACEMENT_3D ( 'NONE', #42277, #110581, #108935 ) ;
#87558=VERTEX_POINT ( 'NONE', #19824 ) ;
#87583=AXIS2_PLACEMENT_3D ( 'NONE', #24794, #58999, #93127 ) ;
#87634=CARTESIAN_POINT ( 'NONE',  ( 1.823067188510389982E-15, 1517.051704408389924, 209.1218459616989946 ) ) ;
#87677=EDGE_CURVE ( 'NONE', #41248, #3770, #105538, .T. ) ;
#87680=AXIS2_PLACEMENT_3D ( 'NONE', #34480, #94940, #10942 ) ;
#87682=EDGE_CURVE ( 'NONE', #79550, #3955, #41186, .T. ) ;
#87693=CARTESIAN_POINT ( 'NONE',  ( 15.72751745975079984, 1517.151704408390060, 206.8816388537309763 ) ) ;
#87708=ORIENTED_EDGE ( 'NONE', *, *, #52789, .F. ) ;
#87711=CARTESIAN_POINT ( 'NONE',  ( -17.68237282055029880, 1517.151704408390060, 205.6847408665509818 ) ) ;
#87716=EDGE_CURVE ( 'NONE', #1004, #84814, #100396, .T. ) ;
#87747=LINE ( 'NONE', #29466, #56291 ) ;
#87752=DIRECTION ( 'NONE',  ( 5.980589973904019347E-17, -1.000000000000000000, 1.736889445713099699E-16 ) ) ;
#87784=DIRECTION ( 'NONE',  ( -1.755985294532469921E-16, 1.000000000000000000, -1.338183447452831989E-16 ) ) ;
#87797=CIRCLE ( 'NONE', #82428, 1.999999999999999556 ) ;
#87802=ORIENTED_EDGE ( 'NONE', *, *, #20343, .F. ) ;
#87806=AXIS2_PLACEMENT_3D ( 'NONE', #12414, #38712, #65038 ) ;
#87817=VECTOR ( 'NONE', #34702, 1000.000000000000000 ) ;
#87859=FACE_OUTER_BOUND ( 'NONE', #40946, .T. ) ;
#87916=ORIENTED_EDGE ( 'NONE', *, *, #54949, .T. ) ;
#87948=EDGE_LOOP ( 'NONE', ( #87098, #35042 ) ) ;
#87952=CARTESIAN_POINT ( 'NONE',  ( 3.331783404088239919, 1517.151704408390060, 197.4348858789911674 ) ) ;
#87972=VERTEX_POINT ( 'NONE', #81655 ) ;
#87974=AXIS2_PLACEMENT_3D ( 'NONE', #109343, #81909, #67349 ) ;
#87992=ADVANCED_FACE ( 'NONE', ( #88969 ), #20642, .F. ) ;
#88024=CARTESIAN_POINT ( 'NONE',  ( 1.925297170580940076, 1522.051704408389924, 230.6853930747409720 ) ) ;
#88025=CARTESIAN_POINT ( 'NONE',  ( -1.000362776118160035E-16, 1517.151704408390060, 209.1218459616989946 ) ) ;
#88042=CARTESIAN_POINT ( 'NONE',  ( 11.75869035456349998, 1521.951704408389787, 227.2994842691620079 ) ) ;
#88046=DIRECTION ( 'NONE',  ( -1.755985294532469921E-16, 1.000000000000000000, -1.338183447452831989E-16 ) ) ;
#88050=CARTESIAN_POINT ( 'NONE',  ( 4.517196230222680242, 1517.151704408390060, 227.6318199458918343 ) ) ;
#88054=CIRCLE ( 'NONE', #39752, 2.000000000000003553 ) ;
#88100=DIRECTION ( 'NONE',  ( -0.6736849260863841948, 0.000000000000000000, 0.7390186874254148774 ) ) ;
#88123=CARTESIAN_POINT ( 'NONE',  ( 7.848979634317430509, 1517.151704408390060, 215.9448598632019980 ) ) ;
#88130=DIRECTION ( 'NONE',  ( -1.755985294532469921E-16, 1.000000000000000000, -1.338183447452831989E-16 ) ) ;
#88147=ORIENTED_EDGE ( 'NONE', *, *, #94723, .F. ) ;
#88221=ORIENTED_EDGE ( 'NONE', *, *, #74901, .T. ) ;
#88283=DIRECTION ( 'NONE',  ( -1.755985294532469921E-16, 1.000000000000000000, -1.338183447452831989E-16 ) ) ;
#88300=CARTESIAN_POINT ( 'NONE',  ( 9.196349486490200675, 1517.051704408389924, 214.4668224883511698 ) ) ;
#88303=EDGE_CURVE ( 'NONE', #48781, #34958, #21487, .T. ) ;
#88314=FACE_OUTER_BOUND ( 'NONE', #101082, .T. ) ;
#88333=CARTESIAN_POINT ( 'NONE',  ( -17.66967187194796551, 1517.051704408389924, 195.1406325242839159 ) ) ;
#88373=ORIENTED_EDGE ( 'NONE', *, *, #35846, .F. ) ;
#88379=FACE_OUTER_BOUND ( 'NONE', #49362, .T. ) ;
#88424=EDGE_CURVE ( 'NONE', #30117, #8025, #16922, .T. ) ;
#88426=EDGE_LOOP ( 'NONE', ( #44435, #71569 ) ) ;
#88440=DIRECTION ( 'NONE',  ( 5.980589973904019347E-17, -1.000000000000000000, 1.736889445713099699E-16 ) ) ;
#88495=DIRECTION ( 'NONE',  ( 0.9455185755993178454, 0.000000000000000000, -0.3255681544571537578 ) ) ;
#88500=EDGE_CURVE ( 'NONE', #98761, #85274, #100164, .T. ) ;
#88501=CARTESIAN_POINT ( 'NONE',  ( 1.925297170580940076, 1519.551704408389924, 230.6853930747409720 ) ) ;
#88524=CARTESIAN_POINT ( 'NONE',  ( -17.71193101166619854, 1521.951704408389787, 221.5709757775249784 ) ) ;
#88537=AXIS2_PLACEMENT_3D ( 'NONE', #18922, #101821, #93986 ) ;
#88550=EDGE_CURVE ( 'NONE', #1585, #103193, #10778, .T. ) ;
#88565=DIRECTION ( 'NONE',  ( 0.9858563016923833633, 0.000000000000000000, 0.1675928173085483863 ) ) ;
#88570=ADVANCED_FACE ( 'NONE', ( #63415 ), #37071, .F. ) ;
#88589=FACE_OUTER_BOUND ( 'NONE', #23170, .T. ) ;
#88627=AXIS2_PLACEMENT_3D ( 'NONE', #41853, #110161, #93350 ) ;
#88644=ORIENTED_EDGE ( 'NONE', *, *, #55661, .F. ) ;
#88646=VERTEX_POINT ( 'NONE', #86367 ) ;
#88671=DIRECTION ( 'NONE',  ( -5.980589973904019347E-17, 1.000000000000000000, -1.736889445713099699E-16 ) ) ;
#88674=CARTESIAN_POINT ( 'NONE',  ( -13.16517659032116860, 1517.051704408389924, 224.1947148507618408 ) ) ;
#88720=EDGE_CURVE ( 'NONE', #64221, #102140, #37677, .T. ) ;
#88753=LINE ( 'NONE', #54076, #90802 ) ;
#88782=ORIENTED_EDGE ( 'NONE', *, *, #17238, .F. ) ;
#88816=CARTESIAN_POINT ( 'NONE',  ( -19.63722818134010240, 1517.051704408389924, 200.0074286634620364 ) ) ;
#88831=CYLINDRICAL_SURFACE ( 'NONE', #56816, 2.000000000000002220 ) ;
#88843=ADVANCED_FACE ( 'NONE', ( #81262 ), #4577, .F. ) ;
#88848=FACE_OUTER_BOUND ( 'NONE', #56141, .T. ) ;
#88871=ORIENTED_EDGE ( 'NONE', *, *, #102131, .T. ) ;
#88876=DIRECTION ( 'NONE',  ( -5.980589973904019347E-17, 1.000000000000000000, -1.736889445713099699E-16 ) ) ;
#88881=VECTOR ( 'NONE', #74232, 999.9999999999998863 ) ;
#88895=FACE_OUTER_BOUND ( 'NONE', #86964, .T. ) ;
#88905=ORIENTED_EDGE ( 'NONE', *, *, #97268, .T. ) ;
#88918=FACE_OUTER_BOUND ( 'NONE', #94410, .T. ) ;
#88923=CARTESIAN_POINT ( 'NONE',  ( 1.925297170580940076, 1522.051704408389924, 230.6853930747409720 ) ) ;
#88930=CIRCLE ( 'NONE', #90679, 1.999999999999999556 ) ;
#88934=VERTEX_POINT ( 'NONE', #597 ) ;
#88954=AXIS2_PLACEMENT_3D ( 'NONE', #93675, #34347, #42203 ) ;
#88969=FACE_OUTER_BOUND ( 'NONE', #5144, .T. ) ;
#88979=CIRCLE ( 'NONE', #83620, 1.999999999999999556 ) ;
#88995=DIRECTION ( 'NONE',  ( 0.9455185755993178454, 0.000000000000000000, -0.3255681544571539243 ) ) ;
#89015=DIRECTION ( 'NONE',  ( -0.6736849260863841948, 0.000000000000000000, 0.7390186874254148774 ) ) ;
#89022=LINE ( 'NONE', #87952, #18552 ) ;
#89023=ORIENTED_EDGE ( 'NONE', *, *, #64701, .F. ) ;
#89031=CIRCLE ( 'NONE', #81836, 1.999999999999999556 ) ;
#89046=ORIENTED_EDGE ( 'NONE', *, *, #99829, .T. ) ;
#89055=CARTESIAN_POINT ( 'NONE',  ( -13.72624666517843472, 1521.951704408389787, 195.8110037935180969 ) ) ;
#89059=EDGE_CURVE ( 'NONE', #107071, #70320, #68150, .T. ) ;
#89061=CARTESIAN_POINT ( 'NONE',  ( 6.531167973260559201, 1517.151704408390060, 201.5366623270788295 ) ) ;
#89063=CIRCLE ( 'NONE', #40786, 1.999999999999999556 ) ;
#89073=EDGE_CURVE ( 'NONE', #58638, #35907, #33067, .T. ) ;
#89086=EDGE_CURVE ( 'NONE', #96069, #101117, #73496, .T. ) ;
#89147=EDGE_CURVE ( 'NONE', #64955, #37540, #10901, .T. ) ;
#89185=EDGE_CURVE ( 'NONE', #16564, #52504, #16210, .T. ) ;
#89198=CARTESIAN_POINT ( 'NONE',  ( -6.954065720117950100, 1517.551704408389924, 183.5505540514350002 ) ) ;
#89219=ORIENTED_EDGE ( 'NONE', *, *, #32389, .F. ) ;
#89239=CARTESIAN_POINT ( 'NONE',  ( -0.04641543425164652847, 1517.051704408389924, 230.3502074417858978 ) ) ;
#89255=AXIS2_PLACEMENT_3D ( 'NONE', #67786, #25190, #76170 ) ;
#89284=CARTESIAN_POINT ( 'NONE',  ( 7.848979634317430509, 1522.051704408389924, 215.9448598632019980 ) ) ;
#89307=ORIENTED_EDGE ( 'NONE', *, *, #97268, .F. ) ;
#89314=DIRECTION ( 'NONE',  ( 0.9455185755993178454, 0.000000000000000000, -0.3255681544571539243 ) ) ;
#89345=AXIS2_PLACEMENT_3D ( 'NONE', #69457, #88440, #104130 ) ;
#89381=CARTESIAN_POINT ( 'NONE',  ( -8.301987938657498844, 1522.051704408389924, 185.0111222839169898 ) ) ;
#89397=ORIENTED_EDGE ( 'NONE', *, *, #60037, .F. ) ;
#89483=CARTESIAN_POINT ( 'NONE',  ( -19.66678637224480397, 1517.151704408390060, 215.8936635741279986 ) ) ;
#89489=CARTESIAN_POINT ( 'NONE',  ( -2.621457251404222255, 1522.051704408389924, 228.0616540033011574 ) ) ;
#89516=CARTESIAN_POINT ( 'NONE',  ( 3.909710721586129534, 1517.151704408390060, 220.4764703678949900 ) ) ;
#89528=CARTESIAN_POINT ( 'NONE',  ( -8.456465142934460388, 1517.051704408389924, 195.1434824822571841 ) ) ;
#89540=ORIENTED_EDGE ( 'NONE', *, *, #13079, .T. ) ;
#89545=AXIS2_PLACEMENT_3D ( 'NONE', #26986, #9073, #34821 ) ;
#89564=DIRECTION ( 'NONE',  ( 1.755985294532469921E-16, -1.000000000000000000, 1.338183447452831989E-16 ) ) ;
#89572=ORIENTED_EDGE ( 'NONE', *, *, #82087, .T. ) ;
#89587=ORIENTED_EDGE ( 'NONE', *, *, #42783, .T. ) ;
#89595=ORIENTED_EDGE ( 'NONE', *, *, #98660, .F. ) ;
#89703=CARTESIAN_POINT ( 'NONE',  ( -15.09047375999177021, 1517.151704408390060, 202.6311677367078232 ) ) ;
#89705=CARTESIAN_POINT ( 'NONE',  ( -19.63722818156799832, 1519.551704408389924, 200.0074286628000095 ) ) ;
#89715=EDGE_CURVE ( 'NONE', #35721, #43348, #26974, .T. ) ;
#89739=ORIENTED_EDGE ( 'NONE', *, *, #82984, .F. ) ;
#89855=CYLINDRICAL_SURFACE ( 'NONE', #29532, 2.000000000000003553 ) ;
#89895=CARTESIAN_POINT ( 'NONE',  ( -21.62164173326539895, 1517.051704408389924, 210.2163513712909833 ) ) ;
#89904=ORIENTED_EDGE ( 'NONE', *, *, #2988, .F. ) ;
#89930=CARTESIAN_POINT ( 'NONE',  ( -19.66678637224480397, 1519.551704408389924, 215.8936635741279986 ) ) ;
#89968=DIRECTION ( 'NONE',  ( -5.980589973904019347E-17, 1.000000000000000000, -1.736889445713099699E-16 ) ) ;
#90029=CARTESIAN_POINT ( 'NONE',  ( 5.257080573758899256, 1517.151704408390060, 218.9984329930441618 ) ) ;
#90047=DIRECTION ( 'NONE',  ( 1.755985294532469921E-16, -1.000000000000000000, 1.338183447452831989E-16 ) ) ;
#90055=EDGE_LOOP ( 'NONE', ( #56011, #41058, #71129, #59897 ) ) ;
#90068=VECTOR ( 'NONE', #93978, 1000.000000000000000 ) ;
#90069=DIRECTION ( 'NONE',  ( -0.9455185755993178454, 0.000000000000000000, 0.3255681544571539243 ) ) ;
#90079=ORIENTED_EDGE ( 'NONE', *, *, #52242, .T. ) ;
#90092=VECTOR ( 'NONE', #105158, 1000.000000000000000 ) ;
#90107=EDGE_CURVE ( 'NONE', #104584, #105548, #62816, .T. ) ;
#90130=DIRECTION ( 'NONE',  ( 0.9455185755993178454, 0.000000000000000000, -0.3255681544571537578 ) ) ;
#90181=CARTESIAN_POINT ( 'NONE',  ( -3.968827101022720072, 1521.951704408389787, 229.5396913742049776 ) ) ;
#90227=CARTESIAN_POINT ( 'NONE',  ( 21.62164173326539895, 1517.151704408390060, 208.0273405521070060 ) ) ;
#90239=EDGE_LOOP ( 'NONE', ( #70501, #16160, #105799, #101578, #4156 ) ) ;
#90277=VERTEX_POINT ( 'NONE', #24063 ) ;
#90312=CYLINDRICAL_SURFACE ( 'NONE', #43044, 2.000000000000003553 ) ;
#90323=VECTOR ( 'NONE', #99692, 1000.000000000000000 ) ;
#90336=DIRECTION ( 'NONE',  ( -5.980589973904019347E-17, 1.000000000000000000, -1.736889445713099699E-16 ) ) ;
#90345=CIRCLE ( 'NONE', #88627, 1.999999999999999556 ) ;
#90350=EDGE_CURVE ( 'NONE', #61329, #62788, #53933, .T. ) ;
#90360=CARTESIAN_POINT ( 'NONE',  ( -6.790918657024139549, 1522.051704408389924, 184.0243675267330161 ) ) ;
#90388=VERTEX_POINT ( 'NONE', #7828 ) ;
#90393=FACE_OUTER_BOUND ( 'NONE', #28678, .T. ) ;
#90398=DIRECTION ( 'NONE',  ( -0.6736849260863841948, 0.000000000000000000, 0.7390186874254148774 ) ) ;
#90421=FACE_OUTER_BOUND ( 'NONE', #11594, .T. ) ;
#90468=ORIENTED_EDGE ( 'NONE', *, *, #71913, .F. ) ;
#90488=DIRECTION ( 'NONE',  ( -1.755985294532469921E-16, 1.000000000000000000, -1.338183447452831989E-16 ) ) ;
#90511=ORIENTED_EDGE ( 'NONE', *, *, #4812, .T. ) ;
#90539=EDGE_CURVE ( 'NONE', #18256, #21199, #18065, .T. ) ;
#90598=ORIENTED_EDGE ( 'NONE', *, *, #82087, .F. ) ;
#90636=EDGE_LOOP ( 'NONE', ( #40704, #45566 ) ) ;
#90679=AXIS2_PLACEMENT_3D ( 'NONE', #22506, #63489, #20879 ) ;
#90745=EDGE_CURVE ( 'NONE', #96193, #98249, #109294, .T. ) ;
#90772=ORIENTED_EDGE ( 'NONE', *, *, #44085, .T. ) ;
#90802=VECTOR ( 'NONE', #12036, 1000.000000000000000 ) ;
#90814=ORIENTED_EDGE ( 'NONE', *, *, #1747, .F. ) ;
#90818=ORIENTED_EDGE ( 'NONE', *, *, #2988, .T. ) ;
#90831=ORIENTED_EDGE ( 'NONE', *, *, #89059, .F. ) ;
#90851=ORIENTED_EDGE ( 'NONE', *, *, #77435, .T. ) ;
#90855=EDGE_CURVE ( 'NONE', #52731, #1004, #2045, .T. ) ;
#90869=VECTOR ( 'NONE', #66536, 1000.000000000000000 ) ;
#90876=CIRCLE ( 'NONE', #99816, 2.000000000000003553 ) ;
#90901=CARTESIAN_POINT ( 'NONE',  ( -11.21032122992201785, 1517.151704408390060, 229.8720270527158220 ) ) ;
#90904=CARTESIAN_POINT ( 'NONE',  ( -0.5779273184081722414, 1519.551704408389924, 186.0802614738061607 ) ) ;
#90950=ORIENTED_EDGE ( 'NONE', *, *, #52303, .T. ) ;
#90964=ORIENTED_EDGE ( 'NONE', *, *, #15183, .F. ) ;
#91004=CIRCLE ( 'NONE', #10608, 26.00000000000000711 ) ;
#91012=CIRCLE ( 'NONE', #8756, 1.999999999999999556 ) ;
#91042=CARTESIAN_POINT ( 'NONE',  ( -9.803834995107230554, 1517.151704408390060, 196.6215198571080123 ) ) ;
#91053=CARTESIAN_POINT ( 'NONE',  ( 7.848979634317430509, 1517.051704408389924, 215.9448598632019980 ) ) ;
#91084=CARTESIAN_POINT ( 'NONE',  ( 19.63722818094939981, 1521.951704408389787, 218.2362632588020119 ) ) ;
#91108=CARTESIAN_POINT ( 'NONE',  ( -6.871715297790212063, 1521.804095990991300, 183.7897170437400973 ) ) ;
#91146=AXIS2_PLACEMENT_3D ( 'NONE', #83338, #98482, #21750 ) ;
#91162=CARTESIAN_POINT ( 'NONE',  ( -11.78824854703250047, 1517.051704408389924, 206.8304425649369875 ) ) ;
#91187=CARTESIAN_POINT ( 'NONE',  ( -5.134308048384249940E-13, 1492.051704408390151, 209.1218459616989946 ) ) ;
#91217=EDGE_LOOP ( 'NONE', ( #54171, #38734 ) ) ;
#91234=ORIENTED_EDGE ( 'NONE', *, *, #97083, .T. ) ;
#91238=ORIENTED_EDGE ( 'NONE', *, *, #67827, .T. ) ;
#91251=DIRECTION ( 'NONE',  ( -0.6736849260863841948, 0.000000000000000000, 0.7390186874254148774 ) ) ;
#91253=ORIENTED_EDGE ( 'NONE', *, *, #93511, .F. ) ;
#91285=CARTESIAN_POINT ( 'NONE',  ( 15.72751745975079984, 1517.051704408389924, 206.8816388537309763 ) ) ;
#91311=EDGE_LOOP ( 'NONE', ( #65382, #9887, #32138, #26868, #1044 ) ) ;
#91326=EDGE_LOOP ( 'NONE', ( #108403, #74548, #9419, #23631 ) ) ;
#91364=ORIENTED_EDGE ( 'NONE', *, *, #38006, .T. ) ;
#91394=ADVANCED_FACE ( 'NONE', ( #10336 ), #9787, .F. ) ;
#91405=CARTESIAN_POINT ( 'NONE',  ( 4.517196230222682019, 1522.051704408389924, 227.6318199458918343 ) ) ;
#91488=CIRCLE ( 'NONE', #73687, 2.000000000000011102 ) ;
#91491=ORIENTED_EDGE ( 'NONE', *, *, #42812, .T. ) ;
#91497=VERTEX_POINT ( 'NONE', #29340 ) ;
#91499=LINE ( 'NONE', #81974, #6419 ) ;
#91511=ORIENTED_EDGE ( 'NONE', *, *, #8534, .T. ) ;
#91514=EDGE_LOOP ( 'NONE', ( #45769, #2356, #51821, #89587, #87428 ) ) ;
#91539=CIRCLE ( 'NONE', #32548, 2.000000000000002220 ) ;
#91551=ORIENTED_EDGE ( 'NONE', *, *, #9807, .F. ) ;
#91557=CARTESIAN_POINT ( 'NONE',  ( -3.331783404088239919, 1517.151704408390060, 220.8088060444078451 ) ) ;
#91584=ORIENTED_EDGE ( 'NONE', *, *, #22823, .F. ) ;
#91585=DIRECTION ( 'NONE',  ( 1.755985294532469921E-16, -1.000000000000000000, 1.338183447452831989E-16 ) ) ;
#91608=CARTESIAN_POINT ( 'NONE',  ( -15.69795926856320101, 1521.951704408389787, 195.4758181589010064 ) ) ;
#91641=FACE_OUTER_BOUND ( 'NONE', #65455, .T. ) ;
#91643=AXIS2_PLACEMENT_3D ( 'NONE', #66533, #83850, #74378 ) ;
#91652=CARTESIAN_POINT ( 'NONE',  ( -21.01415622427472485, 1517.151704408390060, 217.3717009491090835 ) ) ;
#91655=ORIENTED_EDGE ( 'NONE', *, *, #104765, .F. ) ;
#91673=EDGE_LOOP ( 'NONE', ( #13010, #51382, #90079, #23433, #67861 ) ) ;
#91717=DIRECTION ( 'NONE',  ( -1.755985294532464991E-16, 1.000000000000000000, -1.338183447452830017E-16 ) ) ;
#91727=EDGE_CURVE ( 'NONE', #21912, #88646, #6349, .T. ) ;
#91730=CYLINDRICAL_SURFACE ( 'NONE', #85351, 1.749999999999997558 ) ;
#91759=DIRECTION ( 'NONE',  ( -1.755985294532469921E-16, 1.000000000000000000, -1.338183447452831989E-16 ) ) ;
#91765=CARTESIAN_POINT ( 'NONE',  ( 7.878537825433329367, 1517.051704408389924, 200.0586249522280013 ) ) ;
#91771=EDGE_LOOP ( 'NONE', ( #8812, #107990 ) ) ;
#91773=DIRECTION ( 'NONE',  ( 0.9455185755993178454, 0.000000000000000000, -0.3255681544571539243 ) ) ;
#91784=EDGE_CURVE ( 'NONE', #37972, #48060, #50390, .T. ) ;
#91812=EDGE_CURVE ( 'NONE', #105548, #8134, #25323, .T. ) ;
#91814=ORIENTED_EDGE ( 'NONE', *, *, #238, .T. ) ;
#91832=CIRCLE ( 'NONE', #48948, 1.999999999999999556 ) ;
#91873=EDGE_CURVE ( 'NONE', #82777, #3107, #47128, .T. ) ;
#91957=CARTESIAN_POINT ( 'NONE',  ( -17.66551557795533611, 1517.051704408389924, 200.3426142980791269 ) ) ;
#92003=CIRCLE ( 'NONE', #22437, 1.999999999999999556 ) ;
#92008=AXIS2_PLACEMENT_3D ( 'NONE', #69298, #87752, #1534 ) ;
#92009=DIRECTION ( 'NONE',  ( -0.9455185755993178454, 0.000000000000000000, 0.3255681544571537578 ) ) ;
#92031=LINE ( 'NONE', #83081, #92904 ) ;
#92059=VERTEX_POINT ( 'NONE', #17335 ) ;
#92071=ORIENTED_EDGE ( 'NONE', *, *, #3648, .T. ) ;
#92082=AXIS2_PLACEMENT_3D ( 'NONE', #106930, #30220, #66070 ) ;
#92104=DIRECTION ( 'NONE',  ( -1.755985294532469921E-16, 1.000000000000000000, -1.338183447452831989E-16 ) ) ;
#92163=FACE_BOUND ( 'NONE', #51858, .T. ) ;
#92186=DIRECTION ( 'NONE',  ( -1.755985294532469921E-16, 1.000000000000000000, -1.338183447452831989E-16 ) ) ;
#92195=CARTESIAN_POINT ( 'NONE',  ( 1.925297170580940076, 1519.551704408389924, 230.6853930747409720 ) ) ;
#92196=ORIENTED_EDGE ( 'NONE', *, *, #39862, .T. ) ;
#92198=CIRCLE ( 'NONE', #43928, 1.999999999999998668 ) ;
#92207=EDGE_LOOP ( 'NONE', ( #62613, #68739, #103301, #76114 ) ) ;
#92237=ORIENTED_EDGE ( 'NONE', *, *, #58517, .F. ) ;
#92251=EDGE_CURVE ( 'NONE', #25680, #5162, #75412, .T. ) ;
#92268=VECTOR ( 'NONE', #63418, 1000.000000000000000 ) ;
#92273=ORIENTED_EDGE ( 'NONE', *, *, #60388, .T. ) ;
#92277=ORIENTED_EDGE ( 'NONE', *, *, #58984, .F. ) ;
#92281=DIRECTION ( 'NONE',  ( -5.980589973904019347E-17, 1.000000000000000000, -1.736889445713099699E-16 ) ) ;
#92298=CARTESIAN_POINT ( 'NONE',  ( -2.562340869413339828, 1517.151704408390060, 196.2891841806521711 ) ) ;
#92320=ORIENTED_EDGE ( 'NONE', *, *, #93379, .F. ) ;
#92326=EDGE_LOOP ( 'NONE', ( #95785, #7697, #31021, #80720 ) ) ;
#92377=CARTESIAN_POINT ( 'NONE',  ( -17.71193100849139768, 1519.551704408389924, 221.5709757781449980 ) ) ;
#92392=CARTESIAN_POINT ( 'NONE',  ( 0.6370436997427018078, 1522.051704408389924, 200.3909606286928238 ) ) ;
#92448=CARTESIAN_POINT ( 'NONE',  ( -5.923682464646780943, 1522.051704408389924, 223.8623791742500089 ) ) ;
#92483=EDGE_CURVE ( 'NONE', #69558, #34577, #43971, .T. ) ;
#92495=AXIS2_PLACEMENT_3D ( 'NONE', #67346, #93063, #25843 ) ;
#92497=ORIENTED_EDGE ( 'NONE', *, *, #25421, .T. ) ;
#92537=ADVANCED_FACE ( 'NONE', ( #110193 ), #50318, .F. ) ;
#92561=CARTESIAN_POINT ( 'NONE',  ( -18.31941652021488665, 1522.051704408389924, 214.4156261991469421 ) ) ;
#92568=DIRECTION ( 'NONE',  ( 5.980589973904019347E-17, -1.000000000000000000, 1.736889445713099699E-16 ) ) ;
#92572=FACE_BOUND ( 'NONE', #101935, .T. ) ;
#92620=VERTEX_POINT ( 'NONE', #3095 ) ;
#92627=CIRCLE ( 'NONE', #49729, 1.999999999999999556 ) ;
#92631=AXIS2_PLACEMENT_3D ( 'NONE', #47804, #90336, #81939 ) ;
#92633=LINE ( 'NONE', #9202, #35665 ) ;
#92649=DIRECTION ( 'NONE',  ( 0.9455185755993178454, 0.000000000000000000, -0.3255681544571537578 ) ) ;
#92667=CARTESIAN_POINT ( 'NONE',  ( 19.05930086383897049, 1517.151704408390060, 195.1946787710221827 ) ) ;
#92691=EDGE_CURVE ( 'NONE', #76035, #32612, #19852, .T. ) ;
#92703=AXIS2_PLACEMENT_3D ( 'NONE', #20006, #63702, #36818 ) ;
#92706=FACE_BOUND ( 'NONE', #61953, .T. ) ;
#92711=CYLINDRICAL_SURFACE ( 'NONE', #85466, 2.000000000000003553 ) ;
#92723=DIRECTION ( 'NONE',  ( -1.755985294532469921E-16, 1.000000000000000000, -1.338183447452831989E-16 ) ) ;
#92742=CARTESIAN_POINT ( 'NONE',  ( 21.62164173326539895, 1517.151704408390060, 208.0273405521070060 ) ) ;
#92766=EDGE_CURVE ( 'NONE', #76507, #22264, #54600, .T. ) ;
#92780=PLANE ( 'NONE',  #471 ) ;
#92783=CIRCLE ( 'NONE', #78497, 1.999999999999999556 ) ;
#92808=DIRECTION ( 'NONE',  ( 5.980589973904019347E-17, -1.000000000000000000, 1.736889445713099699E-16 ) ) ;
#92897=EDGE_CURVE ( 'NONE', #26041, #86132, #95134, .T. ) ;
#92904=VECTOR ( 'NONE', #92568, 1000.000000000000000 ) ;
#92918=DIRECTION ( 'NONE',  ( 1.755985294532464991E-16, -1.000000000000000000, 1.338183447452830017E-16 ) ) ;
#92966=DIRECTION ( 'NONE',  ( -5.980589973904019347E-17, 1.000000000000000000, -1.736889445713099699E-16 ) ) ;
#93030=ORIENTED_EDGE ( 'NONE', *, *, #61058, .T. ) ;
#93063=DIRECTION ( 'NONE',  ( 5.980589973904019347E-17, -1.000000000000000000, 1.736889445713099699E-16 ) ) ;
#93088=EDGE_CURVE ( 'NONE', #84204, #53816, #23707, .T. ) ;
#93107=ADVANCED_FACE ( 'NONE', ( #104294 ), #9128, .F. ) ;
#93110=CARTESIAN_POINT ( 'NONE',  ( 13.16517659032116860, 1522.051704408389924, 194.0489770726361485 ) ) ;
#93127=DIRECTION ( 'NONE',  ( -0.6736849260863839728, 0.000000000000000000, 0.7390186874254150995 ) ) ;
#93130=FACE_BOUND ( 'NONE', #34920, .T. ) ;
#93134=ORIENTED_EDGE ( 'NONE', *, *, #49297, .T. ) ;
#93138=VERTEX_POINT ( 'NONE', #94783 ) ;
#93145=AXIS2_PLACEMENT_3D ( 'NONE', #1956, #20366, #97644 ) ;
#93161=PRODUCT_DEFINITION ( 'UNKNOWN', '', #51243, #51345 ) ;
#93181=( GEOMETRIC_REPRESENTATION_CONTEXT ( 3 ) GLOBAL_UNCERTAINTY_ASSIGNED_CONTEXT ( ( #84931 ) ) GLOBAL_UNIT_ASSIGNED_CONTEXT ( ( #81981, #13658, #108850 ) ) REPRESENTATION_CONTEXT ( 'NONE', 'WORKASPACE' ) );
#93189=AXIS2_PLACEMENT_3D ( 'NONE', #18123, #52319, #86443 ) ;
#93200=AXIS2_PLACEMENT_3D ( 'NONE', #85495, #7160, #8794 ) ;
#93207=EDGE_CURVE ( 'NONE', #21199, #58053, #91539, .T. ) ;
#93212=FACE_OUTER_BOUND ( 'NONE', #62167, .T. ) ;
#93228=DIRECTION ( 'NONE',  ( -0.6736849260863839728, 0.000000000000000000, 0.7390186874254150995 ) ) ;
#93244=FACE_OUTER_BOUND ( 'NONE', #15729, .T. ) ;
#93260=FACE_BOUND ( 'NONE', #12830, .T. ) ;
#93284=ORIENTED_EDGE ( 'NONE', *, *, #77689, .T. ) ;
#93340=DIRECTION ( 'NONE',  ( -1.755985294532469921E-16, 1.000000000000000000, -1.338183447452831989E-16 ) ) ;
#93350=DIRECTION ( 'NONE',  ( 0.9455185755993178454, 0.000000000000000000, -0.3255681544571537578 ) ) ;
#93368=EDGE_LOOP ( 'NONE', ( #62214, #12655, #62058, #101959, #64197 ) ) ;
#93379=EDGE_CURVE ( 'NONE', #46101, #37972, #94084, .T. ) ;
#93387=EDGE_CURVE ( 'NONE', #30117, #75707, #21567, .T. ) ;
#93393=ORIENTED_EDGE ( 'NONE', *, *, #74040, .F. ) ;
#93413=CARTESIAN_POINT ( 'NONE',  ( -19.63722818134010240, 1521.951704408389787, 200.0074286634620364 ) ) ;
#93428=CARTESIAN_POINT ( 'NONE',  ( 4.939530087350459949E-13, 1547.051704408389924, 209.1218459616989946 ) ) ;
#93461=CYLINDRICAL_SURFACE ( 'NONE', #5204, 2.000000000000003109 ) ;
#93493=CYLINDRICAL_SURFACE ( 'NONE', #33571, 1.999999999999999556 ) ;
#93511=EDGE_CURVE ( 'NONE', #97416, #39586, #1961, .T. ) ;
#93541=DIRECTION ( 'NONE',  ( 0.9455185755993178454, 0.000000000000000000, -0.3255681544571537578 ) ) ;
#93577=ORIENTED_EDGE ( 'NONE', *, *, #44085, .F. ) ;
#93584=CARTESIAN_POINT ( 'NONE',  ( -1.317811661047103788, 1517.151704408390060, 194.7136484256038500 ) ) ;
#93593=ORIENTED_EDGE ( 'NONE', *, *, #100899, .F. ) ;
#93641=CARTESIAN_POINT ( 'NONE',  ( -14.35058941781813324, 1519.551704408389924, 193.9977807835901729 ) ) ;
#93662=DIRECTION ( 'NONE',  ( -0.9455185755993178454, 0.000000000000000000, 0.3255681544571539243 ) ) ;
#93665=AXIS2_PLACEMENT_3D ( 'NONE', #63215, #37979, #1633 ) ;
#93668=EDGE_LOOP ( 'NONE', ( #20848, #42603, #27595, #52142, #20162 ) ) ;
#93675=CARTESIAN_POINT ( 'NONE',  ( -7.848979634317430509, 1517.151704408390060, 202.2988320601959913 ) ) ;
#93680=CARTESIAN_POINT ( 'NONE',  ( -3.968827103576990201, 1519.551704408389924, 229.5396913781519856 ) ) ;
#93734=AXIS2_PLACEMENT_3D ( 'NONE', #10441, #25564, #1505 ) ;
#93743=AXIS2_PLACEMENT_3D ( 'NONE', #90227, #20272, #14070 ) ;
#93778=ORIENTED_EDGE ( 'NONE', *, *, #29046, .T. ) ;
#93799=ORIENTED_EDGE ( 'NONE', *, *, #96517, .T. ) ;
#93813=VERTEX_POINT ( 'NONE', #88333 ) ;
#93868=CIRCLE ( 'NONE', #33050, 1.999999999999997780 ) ;
#93879=ORIENTED_EDGE ( 'NONE', *, *, #59650, .T. ) ;
#93894=CARTESIAN_POINT ( 'NONE',  ( 14.38014760757803145, 1522.051704408389924, 208.3596762285818045 ) ) ;
#93901=CARTESIAN_POINT ( 'NONE',  ( 21.62164173114529930, 1521.951704408389787, 208.0273405545509888 ) ) ;
#93928=EDGE_CURVE ( 'NONE', #28739, #52504, #96604, .T. ) ;
#93931=DIRECTION ( 'NONE',  ( -1.755985294532469921E-16, 1.000000000000000000, -1.338183447452831989E-16 ) ) ;
#93968=ORIENTED_EDGE ( 'NONE', *, *, #106382, .F. ) ;
#93976=EDGE_CURVE ( 'NONE', #37540, #61158, #23037, .T. ) ;
#93978=DIRECTION ( 'NONE',  ( -1.755985294532469921E-16, 1.000000000000000000, -1.338183447452831989E-16 ) ) ;
#93986=DIRECTION ( 'NONE',  ( -0.9455185755993178454, 0.000000000000000000, 0.3255681544571537578 ) ) ;
#94034=VECTOR ( 'NONE', #72828, 1000.000000000000000 ) ;
#94084=LINE ( 'NONE', #68373, #64546 ) ;
#94125=EDGE_CURVE ( 'NONE', #37122, #66446, #103974, .T. ) ;
#94235=ORIENTED_EDGE ( 'NONE', *, *, #87682, .F. ) ;
#94244=CARTESIAN_POINT ( 'NONE',  ( -7.878537825433329367, 1522.051704408389924, 218.1850669711710111 ) ) ;
#94258=VECTOR ( 'NONE', #17415, 1000.000000000000000 ) ;
#94287=EDGE_CURVE ( 'NONE', #63901, #31779, #87797, .T. ) ;
#94302=EDGE_LOOP ( 'NONE', ( #98344, #11643 ) ) ;
#94306=CIRCLE ( 'NONE', #42441, 2.000000000000002220 ) ;
#94345=AXIS2_PLACEMENT_3D ( 'NONE', #23260, #75356, #93228 ) ;
#94349=FACE_BOUND ( 'NONE', #52556, .T. ) ;
#94370=DIRECTION ( 'NONE',  ( -0.6736849260863841948, 0.000000000000000000, 0.7390186874254148774 ) ) ;
#94376=ORIENTED_EDGE ( 'NONE', *, *, #87716, .F. ) ;
#94378=CARTESIAN_POINT ( 'NONE',  ( 8.486023334060124768, 1522.051704408389924, 207.2139745301958271 ) ) ;
#94394=ORIENTED_EDGE ( 'NONE', *, *, #91873, .F. ) ;
#94410=EDGE_LOOP ( 'NONE', ( #56663, #39108, #6743, #47163 ) ) ;
#94423=CARTESIAN_POINT ( 'NONE',  ( -3.909710721586120208, 1517.051704408389924, 197.7672215555029993 ) ) ;
#94437=DIRECTION ( 'NONE',  ( 1.755985294532469921E-16, -1.000000000000000000, 1.338183447452831989E-16 ) ) ;
#94457=VECTOR ( 'NONE', #32987, 1000.000000000000000 ) ;
#94466=AXIS2_PLACEMENT_3D ( 'NONE', #40259, #107458, #108008 ) ;
#94482=CIRCLE ( 'NONE', #103431, 1.999999999999998668 ) ;
#94487=DIRECTION ( 'NONE',  ( 1.755985294532469921E-16, -1.000000000000000000, 1.338183447452831989E-16 ) ) ;
#94524=LINE ( 'NONE', #507, #16747 ) ;
#94570=DIRECTION ( 'NONE',  ( -0.6736849260863841948, 0.000000000000000000, 0.7390186874254148774 ) ) ;
#94629=ORIENTED_EDGE ( 'NONE', *, *, #24066, .T. ) ;
#94631=AXIS2_PLACEMENT_3D ( 'NONE', #38987, #22169, #107854 ) ;
#94655=CARTESIAN_POINT ( 'NONE',  ( 21.01415622463857247, 1517.151704408390060, 200.8719909741391803 ) ) ;
#94695=ORIENTED_EDGE ( 'NONE', *, *, #78879, .F. ) ;
#94708=DIRECTION ( 'NONE',  ( -1.755985294532469921E-16, 1.000000000000000000, -1.338183447452831989E-16 ) ) ;
#94710=EDGE_CURVE ( 'NONE', #47910, #35107, #57430, .T. ) ;
#94711=CARTESIAN_POINT ( 'NONE',  ( -17.68237282055029880, 1517.151704408390060, 205.6847408665509818 ) ) ;
#94723=EDGE_CURVE ( 'NONE', #54088, #23279, #52058, .T. ) ;
#94767=DIRECTION ( 'NONE',  ( 1.755985294532464991E-16, -1.000000000000000000, 1.338183447452830017E-16 ) ) ;
#94773=CIRCLE ( 'NONE', #100127, 2.000000000000003553 ) ;
#94783=CARTESIAN_POINT ( 'NONE',  ( 21.63849897547177292, 1517.051704408389924, 202.6852139837136804 ) ) ;
#94847=DIRECTION ( 'NONE',  ( 0.9455185755993178454, 0.000000000000000000, -0.3255681544571537578 ) ) ;
#94897=AXIS2_PLACEMENT_3D ( 'NONE', #51537, #101349, #49339 ) ;
#94938=CARTESIAN_POINT ( 'NONE',  ( 19.05930086383896693, 1519.551704408389924, 195.1946787710221827 ) ) ;
#94940=DIRECTION ( 'NONE',  ( 1.755985294532464991E-16, -1.000000000000000000, 1.338183447452830017E-16 ) ) ;
#94969=AXIS2_PLACEMENT_3D ( 'NONE', #76986, #27132, #87027 ) ;
#94977=AXIS2_PLACEMENT_3D ( 'NONE', #8669, #77557, #68072 ) ;
#95030=FACE_OUTER_BOUND ( 'NONE', #93368, .T. ) ;
#95044=ADVANCED_FACE ( 'NONE', ( #93212 ), #42826, .F. ) ;
#95046=EDGE_LOOP ( 'NONE', ( #99868, #84944, #44658, #88221, #69194 ) ) ;
#95071=CIRCLE ( 'NONE', #73586, 1.999999999999999556 ) ;
#95086=CIRCLE ( 'NONE', #46834, 1.999999999999998668 ) ;
#95087=DIRECTION ( 'NONE',  ( 5.980589973904019347E-17, -1.000000000000000000, 1.736889445713099699E-16 ) ) ;
#95094=CARTESIAN_POINT ( 'NONE',  ( -7.211935934568213469, 1517.051704408389924, 193.5679467272088345 ) ) ;
#95102=ORIENTED_EDGE ( 'NONE', *, *, #17773, .T. ) ;
#95134=CIRCLE ( 'NONE', #80585, 2.000000000000003109 ) ;
#95139=ORIENTED_EDGE ( 'NONE', *, *, #57862, .F. ) ;
#95146=CIRCLE ( 'NONE', #87974, 1.999999999999998668 ) ;
#95176=ORIENTED_EDGE ( 'NONE', *, *, #34939, .F. ) ;
#95185=DIRECTION ( 'NONE',  ( -1.755985294532469921E-16, 1.000000000000000000, -1.338183447452831989E-16 ) ) ;
#95235=LINE ( 'NONE', #28579, #18041 ) ;
#95290=CARTESIAN_POINT ( 'NONE',  ( 7.848979634317430509, 1517.051704408389924, 215.9448598632019980 ) ) ;
#95311=CARTESIAN_POINT ( 'NONE',  ( 3.909710721586129534, 1522.051704408389924, 220.4764703678949900 ) ) ;
#95312=ORIENTED_EDGE ( 'NONE', *, *, #19116, .F. ) ;
#95327=DIRECTION ( 'NONE',  ( 0.3255681544571567554, 0.000000000000000000, 0.9455185755993167351 ) ) ;
#95360=FACE_OUTER_BOUND ( 'NONE', #13524, .T. ) ;
#95379=ORIENTED_EDGE ( 'NONE', *, *, #80268, .F. ) ;
#95397=ORIENTED_EDGE ( 'NONE', *, *, #16504, .T. ) ;
#95421=FACE_OUTER_BOUND ( 'NONE', #107242, .T. ) ;
#95431=VERTEX_POINT ( 'NONE', #13464 ) ;
#95460=DIRECTION ( 'NONE',  ( -5.980589973904019347E-17, 1.000000000000000000, -1.736889445713099699E-16 ) ) ;
#95477=FACE_BOUND ( 'NONE', #53483, .T. ) ;
#95480=CARTESIAN_POINT ( 'NONE',  ( 18.31941652029302858, 1517.151704408390060, 203.8280657238408651 ) ) ;
#95499=EDGE_LOOP ( 'NONE', ( #12047, #92196 ) ) ;
#95510=ADVANCED_FACE ( 'NONE', ( #98591 ), #3471, .F. ) ;
#95527=ADVANCED_FACE ( 'NONE', ( #38141 ), #48214, .F. ) ;
#95567=CARTESIAN_POINT ( 'NONE',  ( -8.301987938657498844, 1517.051704408389924, 185.0111222839169898 ) ) ;
#95578=DIRECTION ( 'NONE',  ( -1.755985294532469921E-16, 1.000000000000000000, -1.338183447452831989E-16 ) ) ;
#95593=EDGE_LOOP ( 'NONE', ( #89046, #28817 ) ) ;
#95599=AXIS2_PLACEMENT_3D ( 'NONE', #28028, #61661, #95787 ) ;
#95603=FACE_OUTER_BOUND ( 'NONE', #33398, .T. ) ;
#95606=CIRCLE ( 'NONE', #109912, 1.999999999999999556 ) ;
#95621=DIRECTION ( 'NONE',  ( -5.980589973904019347E-17, 1.000000000000000000, -1.736889445713099699E-16 ) ) ;
#95641=VECTOR ( 'NONE', #43711, 1000.000000000000000 ) ;
#95647=ORIENTED_EDGE ( 'NONE', *, *, #91784, .F. ) ;
#95655=CARTESIAN_POINT ( 'NONE',  ( -4.576312612474010777, 1517.151704408390060, 222.3843417993991807 ) ) ;
#95681=CIRCLE ( 'NONE', #86724, 1.999999999999999556 ) ;
#95686=LINE ( 'NONE', #77784, #30303 ) ;
#95724=VERTEX_POINT ( 'NONE', #31385 ) ;
#95762=ORIENTED_EDGE ( 'NONE', *, *, #87210, .F. ) ;
#95785=ORIENTED_EDGE ( 'NONE', *, *, #63283, .F. ) ;
#95787=DIRECTION ( 'NONE',  ( 0.9455185755993178454, 0.000000000000000000, -0.3255681544571539243 ) ) ;
#95791=VECTOR ( 'NONE', #105921, 1000.000000000000000 ) ;
#95804=AXIS2_PLACEMENT_3D ( 'NONE', #58368, #43223, #130 ) ;
#95892=DIRECTION ( 'NONE',  ( -1.755985294532469921E-16, 1.000000000000000000, -1.338183447452831989E-16 ) ) ;
#95897=DIRECTION ( 'NONE',  ( 1.755985294532469921E-16, -1.000000000000000000, 1.338183447452831989E-16 ) ) ;
#95926=ORIENTED_EDGE ( 'NONE', *, *, #69911, .F. ) ;
#95953=CARTESIAN_POINT ( 'NONE',  ( -9.803834995107230554, 1517.051704408389924, 196.6215198571080123 ) ) ;
#95958=CARTESIAN_POINT ( 'NONE',  ( 3.897009772517886717, 1517.051704408389924, 231.0205787110200788 ) ) ;
#95969=DIRECTION ( 'NONE',  ( -1.755985294532469921E-16, 1.000000000000000000, -1.338183447452831989E-16 ) ) ;
#96024=FACE_OUTER_BOUND ( 'NONE', #91514, .T. ) ;
#96032=CARTESIAN_POINT ( 'NONE',  ( -10.10023367162169983, 1522.051704408389924, 185.1638560673330005 ) ) ;
#96055=AXIS2_PLACEMENT_3D ( 'NONE', #23365, #57555, #83828 ) ;
#96069=VERTEX_POINT ( 'NONE', #4694 ) ;
#96109=DIRECTION ( 'NONE',  ( -1.755985294532469921E-16, 1.000000000000000000, -1.338183447452831989E-16 ) ) ;
#96123=AXIS2_PLACEMENT_3D ( 'NONE', #89381, #12673, #21601 ) ;
#96126=DIRECTION ( 'NONE',  ( -0.6736849260863841948, 0.000000000000000000, 0.7390186874254148774 ) ) ;
#96167=DIRECTION ( 'NONE',  ( -1.755985294532469921E-16, 1.000000000000000000, -1.338183447452831989E-16 ) ) ;
#96171=DIRECTION ( 'NONE',  ( -0.9455185755993177343, 0.000000000000000000, 0.3255681544571540909 ) ) ;
#96182=DIRECTION ( 'NONE',  ( -0.6736849260863839728, 0.000000000000000000, 0.7390186874254150995 ) ) ;
#96185=ORIENTED_EDGE ( 'NONE', *, *, #93976, .T. ) ;
#96188=CIRCLE ( 'NONE', #64076, 1.999999999999999556 ) ;
#96193=VERTEX_POINT ( 'NONE', #82512 ) ;
#96196=DIRECTION ( 'NONE',  ( -0.6736849260863837507, 0.000000000000000000, 0.7390186874254154326 ) ) ;
#96208=ORIENTED_EDGE ( 'NONE', *, *, #65192, .F. ) ;
#96293=VERTEX_POINT ( 'NONE', #33192 ) ;
#96296=DIRECTION ( 'NONE',  ( -0.9455185755993178454, 0.000000000000000000, 0.3255681544571537578 ) ) ;
#96357=ORIENTED_EDGE ( 'NONE', *, *, #27666, .F. ) ;
#96388=CIRCLE ( 'NONE', #60684, 2.000000000000003109 ) ;
#96404=AXIS2_PLACEMENT_3D ( 'NONE', #54263, #80546, #45309 ) ;
#96440=CYLINDRICAL_SURFACE ( 'NONE', #72968, 2.000000000000003109 ) ;
#96441=ADVANCED_FACE ( 'NONE', ( #27015 ), #19704, .F. ) ;
#96469=CIRCLE ( 'NONE', #10621, 1.999999999999999556 ) ;
#96516=CARTESIAN_POINT ( 'NONE',  ( -11.81780673814840021, 1517.151704408390060, 222.7166774759110126 ) ) ;
#96517=EDGE_CURVE ( 'NONE', #65641, #31476, #1269, .T. ) ;
#96550=CARTESIAN_POINT ( 'NONE',  ( 13.73040295794826626, 1517.051704408389924, 227.6346699037790984 ) ) ;
#96556=AXIS2_PLACEMENT_3D ( 'NONE', #77305, #9527, #25207 ) ;
#96559=CARTESIAN_POINT ( 'NONE',  ( 10.44087869485973030, 1522.051704408389924, 212.8912867333128531 ) ) ;
#96604=LINE ( 'NONE', #63043, #70157 ) ;
#96617=EDGE_CURVE ( 'NONE', #49504, #75704, #10161, .T. ) ;
#96621=CARTESIAN_POINT ( 'NONE',  ( -17.71193100849139768, 1517.151704408390060, 221.5709757781449980 ) ) ;
#96629=CYLINDRICAL_SURFACE ( 'NONE', #9670, 2.000000000000003109 ) ;
#96634=CARTESIAN_POINT ( 'NONE',  ( 5.940539708128936169, 1521.951704408389787, 189.0391861795680768 ) ) ;
#96677=VECTOR ( 'NONE', #19368, 1000.000000000000000 ) ;
#96684=CARTESIAN_POINT ( 'NONE',  ( -6.954065720117950100, 1519.551704408389924, 183.5505540514350002 ) ) ;
#96711=EDGE_LOOP ( 'NONE', ( #28100, #95312, #90468, #64691, #73229 ) ) ;
#96724=CARTESIAN_POINT ( 'NONE',  ( 1.925297170580940076, 1519.551704408389924, 230.6853930747409720 ) ) ;
#96729=ORIENTED_EDGE ( 'NONE', *, *, #76798, .T. ) ;
#96786=DIRECTION ( 'NONE',  ( -1.755985294532469921E-16, 1.000000000000000000, -1.338183447452831989E-16 ) ) ;
#96801=ORIENTED_EDGE ( 'NONE', *, *, #44116, .T. ) ;
#96802=DIRECTION ( 'NONE',  ( -0.6736849260863841948, 0.000000000000000000, 0.7390186874254148774 ) ) ;
#96808=CIRCLE ( 'NONE', #34127, 1.999999999999999556 ) ;
#96811=DIRECTION ( 'NONE',  ( -0.6736849260863841948, 0.000000000000000000, 0.7390186874254148774 ) ) ;
#96838=LINE ( 'NONE', #68894, #87817 ) ;
#96845=EDGE_LOOP ( 'NONE', ( #18346, #78161, #87438, #102677, #42215 ) ) ;
#96846=AXIS2_PLACEMENT_3D ( 'NONE', #50273, #83848, #76002 ) ;
#96858=CIRCLE ( 'NONE', #109329, 1.999999999999998668 ) ;
#96899=CARTESIAN_POINT ( 'NONE',  ( -9.833393186232900263, 1522.051704408389924, 212.5077547680540135 ) ) ;
#96911=AXIS2_PLACEMENT_3D ( 'NONE', #7278, #56591, #57711 ) ;
#96926=CYLINDRICAL_SURFACE ( 'NONE', #82303, 1.999999999999999556 ) ;
#96938=ADVANCED_FACE ( 'NONE', ( #57619 ), #19162, .T. ) ;
#96997=LINE ( 'NONE', #20260, #67196 ) ;
#97058=EDGE_LOOP ( 'NONE', ( #41259, #60593 ) ) ;
#97083=EDGE_CURVE ( 'NONE', #61329, #11259, #86099, .T. ) ;
#97092=ORIENTED_EDGE ( 'NONE', *, *, #98012, .F. ) ;
#97194=LINE ( 'NONE', #62540, #28994 ) ;
#97202=ORIENTED_EDGE ( 'NONE', *, *, #102943, .F. ) ;
#97263=ADVANCED_FACE ( 'NONE', ( #95603 ), #34037, .F. ) ;
#97268=EDGE_CURVE ( 'NONE', #95724, #79870, #87128, .T. ) ;
#97288=DIRECTION ( 'NONE',  ( 0.9455185755993177343, 0.000000000000000000, -0.3255681544571540909 ) ) ;
#97305=DIRECTION ( 'NONE',  ( -1.755985294532469921E-16, 1.000000000000000000, -1.338183447452831989E-16 ) ) ;
#97324=DIRECTION ( 'NONE',  ( -1.755985294532469921E-16, 1.000000000000000000, -1.338183447452831989E-16 ) ) ;
#97325=DIRECTION ( 'NONE',  ( -0.6736849260863841948, 0.000000000000000000, 0.7390186874254148774 ) ) ;
#97343=CARTESIAN_POINT ( 'NONE',  ( 11.75869035672759999, 1519.551704408389924, 227.2994842695800060 ) ) ;
#97374=VERTEX_POINT ( 'NONE', #38183 ) ;
#97379=DIRECTION ( 'NONE',  ( 0.9455185755993178454, 0.000000000000000000, -0.3255681544571537578 ) ) ;
#97416=VERTEX_POINT ( 'NONE', #53219 ) ;
#97441=CIRCLE ( 'NONE', #43815, 1.999999999999999556 ) ;
#97456=EDGE_LOOP ( 'NONE', ( #25985, #910 ) ) ;
#97461=DIRECTION ( 'NONE',  ( 0.9455185755993178454, 0.000000000000000000, -0.3255681544571539243 ) ) ;
#97517=CARTESIAN_POINT ( 'NONE',  ( -11.15120484727999894, 1517.051704408389924, 198.0995572319588405 ) ) ;
#97523=DIRECTION ( 'NONE',  ( -1.755985294532469921E-16, 1.000000000000000000, -1.338183447452831989E-16 ) ) ;
#97563=CYLINDRICAL_SURFACE ( 'NONE', #860, 2.000000000000003553 ) ;
#97611=FACE_OUTER_BOUND ( 'NONE', #109463, .T. ) ;
#97621=VECTOR ( 'NONE', #63446, 1000.000000000000000 ) ;
#97644=DIRECTION ( 'NONE',  ( -0.6736849260863841948, 0.000000000000000000, 0.7390186874254148774 ) ) ;
#97682=ORIENTED_EDGE ( 'NONE', *, *, #41452, .T. ) ;
#97741=ORIENTED_EDGE ( 'NONE', *, *, #67238, .T. ) ;
#97743=DIRECTION ( 'NONE',  ( -1.755985294532469921E-16, 1.000000000000000000, -1.338183447452831989E-16 ) ) ;
#97799=VECTOR ( 'NONE', #63344, 1000.000000000000000 ) ;
#97801=DIRECTION ( 'NONE',  ( 1.755985294532464991E-16, -1.000000000000000000, 1.338183447452830017E-16 ) ) ;
#97825=ORIENTED_EDGE ( 'NONE', *, *, #70554, .F. ) ;
#97870=LINE ( 'NONE', #98973, #80163 ) ;
#97884=EDGE_CURVE ( 'NONE', #110100, #84204, #94306, .T. ) ;
#97897=CIRCLE ( 'NONE', #56845, 1.999999999999998668 ) ;
#97910=DIRECTION ( 'NONE',  ( -0.6736849260149578855, 0.000000000000000000, 0.7390186874905266823 ) ) ;
#97914=EDGE_CURVE ( 'NONE', #1585, #70769, #3155, .T. ) ;
#97920=ADVANCED_FACE ( 'NONE', ( #75509 ), #91730, .F. ) ;
#97952=ORIENTED_EDGE ( 'NONE', *, *, #57594, .T. ) ;
#97963=EDGE_LOOP ( 'NONE', ( #14381, #68278 ) ) ;
#97979=CARTESIAN_POINT ( 'NONE',  ( 16.33500296837753041, 1517.151704408390060, 214.0369884316988305 ) ) ;
#98012=EDGE_CURVE ( 'NONE', #60698, #93813, #60366, .T. ) ;
#98037=DIRECTION ( 'NONE',  ( -1.755985294532469921E-16, 1.000000000000000000, -1.338183447452831989E-16 ) ) ;
#98048=VERTEX_POINT ( 'NONE', #53628 ) ;
#98066=CIRCLE ( 'NONE', #8696, 1.999999999999998668 ) ;
#98096=ORIENTED_EDGE ( 'NONE', *, *, #46086, .T. ) ;
#98113=ORIENTED_EDGE ( 'NONE', *, *, #77513, .F. ) ;
#98147=AXIS2_PLACEMENT_3D ( 'NONE', #12161, #88876, #98368 ) ;
#98149=VECTOR ( 'NONE', #86179, 1000.000000000000000 ) ;
#98187=DIRECTION ( 'NONE',  ( 5.980589973904019347E-17, -1.000000000000000000, 1.736889445713099699E-16 ) ) ;
#98200=FACE_OUTER_BOUND ( 'NONE', #51906, .T. ) ;
#98226=VERTEX_POINT ( 'NONE', #31008 ) ;
#98249=VERTEX_POINT ( 'NONE', #84163 ) ;
#98250=ORIENTED_EDGE ( 'NONE', *, *, #76798, .F. ) ;
#98304=VERTEX_POINT ( 'NONE', #92561 ) ;
#98305=AXIS2_PLACEMENT_3D ( 'NONE', #93901, #92808, #110714 ) ;
#98338=DIRECTION ( 'NONE',  ( 1.755985294532464991E-16, -1.000000000000000000, 1.338183447452830017E-16 ) ) ;
#98343=EDGE_LOOP ( 'NONE', ( #62023, #71619, #4344, #26546 ) ) ;
#98344=ORIENTED_EDGE ( 'NONE', *, *, #89185, .T. ) ;
#98368=DIRECTION ( 'NONE',  ( -0.9455185755993178454, 0.000000000000000000, 0.3255681544571537578 ) ) ;
#98440=DIRECTION ( 'NONE',  ( 5.980589973904019347E-17, -1.000000000000000000, 1.736889445713099699E-16 ) ) ;
#98448=DIRECTION ( 'NONE',  ( -0.6736849260863839728, 0.000000000000000000, 0.7390186874254150995 ) ) ;
#98455=CIRCLE ( 'NONE', #100229, 2.000000000000003109 ) ;
#98464=ORIENTED_EDGE ( 'NONE', *, *, #67162, .T. ) ;
#98482=DIRECTION ( 'NONE',  ( -1.755985294532469921E-16, 1.000000000000000000, -1.338183447452831989E-16 ) ) ;
#98488=ORIENTED_EDGE ( 'NONE', *, *, #5665, .T. ) ;
#98573=CYLINDRICAL_SURFACE ( 'NONE', #96911, 2.000000000000003553 ) ;
#98574=EDGE_CURVE ( 'NONE', #98304, #19461, #89031, .T. ) ;
#98582=DIRECTION ( 'NONE',  ( -0.6736849260863841948, 0.000000000000000000, 0.7390186874254148774 ) ) ;
#98591=FACE_OUTER_BOUND ( 'NONE', #55893, .T. ) ;
#98630=CARTESIAN_POINT ( 'NONE',  ( -13.73040295794826626, 1521.951704408389787, 190.6090220196199141 ) ) ;
#98660=EDGE_CURVE ( 'NONE', #102140, #52122, #14625, .T. ) ;
#98668=FACE_OUTER_BOUND ( 'NONE', #29057, .T. ) ;
#98670=ORIENTED_EDGE ( 'NONE', *, *, #62551, .T. ) ;
#98685=CIRCLE ( 'NONE', #77275, 1.999999999999999556 ) ;
#98689=CARTESIAN_POINT ( 'NONE',  ( 7.509485228916700454E-15, 1517.551704408389924, 209.1218459616989946 ) ) ;
#98753=CYLINDRICAL_SURFACE ( 'NONE', #57523, 2.000000000000003553 ) ;
#98761=VERTEX_POINT ( 'NONE', #10087 ) ;
#98830=ADVANCED_FACE ( 'NONE', ( #86953 ), #78563, .F. ) ;
#98845=CARTESIAN_POINT ( 'NONE',  ( -9.786977755216737407, 1519.551704408389924, 191.2793932881676540 ) ) ;
#98909=ORIENTED_EDGE ( 'NONE', *, *, #86424, .T. ) ;
#98919=EDGE_CURVE ( 'NONE', #108026, #64960, #97897, .T. ) ;
#98921=DIRECTION ( 'NONE',  ( -5.980589973904019347E-17, 1.000000000000000000, -1.736889445713099699E-16 ) ) ;
#98928=EDGE_LOOP ( 'NONE', ( #110112, #59705 ) ) ;
#98933=EDGE_CURVE ( 'NONE', #86983, #53037, #53259, .T. ) ;
#98963=EDGE_LOOP ( 'NONE', ( #63775, #2153, #35363, #13343, #56003 ) ) ;
#98973=CARTESIAN_POINT ( 'NONE',  ( -18.28985832939522993, 1517.151704408390060, 198.5293912879491529 ) ) ;
#98985=DIRECTION ( 'NONE',  ( 5.980589973904019347E-17, -1.000000000000000000, 1.736889445713099699E-16 ) ) ;
#99010=ORIENTED_EDGE ( 'NONE', *, *, #37063, .T. ) ;
#99017=CARTESIAN_POINT ( 'NONE',  ( -17.71193100849139768, 1522.051704408389924, 221.5709757781449980 ) ) ;
#99020=LINE ( 'NONE', #81124, #103651 ) ;
#99049=ORIENTED_EDGE ( 'NONE', *, *, #59577, .F. ) ;
#99061=ORIENTED_EDGE ( 'NONE', *, *, #85403, .F. ) ;
#99069=ORIENTED_EDGE ( 'NONE', *, *, #56834, .T. ) ;
#99122=CYLINDRICAL_SURFACE ( 'NONE', #98305, 1.999999999999999556 ) ;
#99143=CARTESIAN_POINT ( 'NONE',  ( 5.923682464646780943, 1517.051704408389924, 194.3813127491490036 ) ) ;
#99156=VERTEX_POINT ( 'NONE', #70751 ) ;
#99171=FACE_OUTER_BOUND ( 'NONE', #78904, .T. ) ;
#99212=CIRCLE ( 'NONE', #81318, 1.999999999999999556 ) ;
#99222=EDGE_LOOP ( 'NONE', ( #62630, #51581, #23805, #43143 ) ) ;
#99239=FACE_OUTER_BOUND ( 'NONE', #86807, .T. ) ;
#99246=EDGE_LOOP ( 'NONE', ( #89595, #104447, #90964, #56947, #28277 ) ) ;
#99254=CARTESIAN_POINT ( 'NONE',  ( 11.81780673814840021, 1517.151704408390060, 195.5270144474869767 ) ) ;
#99363=ADVANCED_FACE ( 'NONE', ( #88895 ), #61512, .F. ) ;
#99370=CIRCLE ( 'NONE', #40396, 1.999999999999998668 ) ;
#99391=ORIENTED_EDGE ( 'NONE', *, *, #8283, .F. ) ;
#99422=AXIS2_PLACEMENT_3D ( 'NONE', #52987, #54105, #87119 ) ;
#99451=ORIENTED_EDGE ( 'NONE', *, *, #70106, .F. ) ;
#99452=ORIENTED_EDGE ( 'NONE', *, *, #88424, .T. ) ;
#99465=VERTEX_POINT ( 'NONE', #43403 ) ;
#99468=ORIENTED_EDGE ( 'NONE', *, *, #106382, .T. ) ;
#99481=CARTESIAN_POINT ( 'NONE',  ( -15.72751745975079984, 1517.051704408389924, 211.3620530696679793 ) ) ;
#99491=CYLINDRICAL_SURFACE ( 'NONE', #65097, 2.000000000000003109 ) ;
#99518=ORIENTED_EDGE ( 'NONE', *, *, #75563, .F. ) ;
#99574=ADVANCED_FACE ( 'NONE', ( #63539 ), #10903, .F. ) ;
#99618=CARTESIAN_POINT ( 'NONE',  ( 19.66678637246580053, 1522.051704408389924, 202.3500283489900085 ) ) ;
#99628=ORIENTED_EDGE ( 'NONE', *, *, #55531, .F. ) ;
#99692=DIRECTION ( 'NONE',  ( -1.755985294532469921E-16, 1.000000000000000000, -1.338183447452831989E-16 ) ) ;
#99734=AXIS2_PLACEMENT_3D ( 'NONE', #104034, #45263, #1596 ) ;
#99771=VERTEX_POINT ( 'NONE', #6887 ) ;
#99780=CARTESIAN_POINT ( 'NONE',  ( -6.790918657024139549, 1517.051704408389924, 184.0243675267330161 ) ) ;
#99784=CARTESIAN_POINT ( 'NONE',  ( -19.05930086066416962, 1517.151704408390060, 223.0490131529958262 ) ) ;
#99794=DIRECTION ( 'NONE',  ( -0.6736849260863841948, 0.000000000000000000, 0.7390186874254148774 ) ) ;
#99809=VECTOR ( 'NONE', #41019, 1000.000000000000000 ) ;
#99816=AXIS2_PLACEMENT_3D ( 'NONE', #5929, #91585, #33312 ) ;
#99829=EDGE_CURVE ( 'NONE', #38215, #104547, #67641, .T. ) ;
#99843=CARTESIAN_POINT ( 'NONE',  ( -17.71193101166619854, 1517.051704408389924, 221.5709757775249784 ) ) ;
#99849=CYLINDRICAL_SURFACE ( 'NONE', #80140, 1.999999999999999556 ) ;
#99852=DIRECTION ( 'NONE',  ( 1.755985294532469921E-16, -1.000000000000000000, 1.338183447452831989E-16 ) ) ;
#99856=DIRECTION ( 'NONE',  ( -0.6736849260863839728, 0.000000000000000000, 0.7390186874254150995 ) ) ;
#99868=ORIENTED_EDGE ( 'NONE', *, *, #67162, .F. ) ;
#99902=AXIS2_PLACEMENT_3D ( 'NONE', #58783, #100754, #94570 ) ;
#99904=ORIENTED_EDGE ( 'NONE', *, *, #96617, .T. ) ;
#99914=ORIENTED_EDGE ( 'NONE', *, *, #85030, .F. ) ;
#99935=DIRECTION ( 'NONE',  ( 0.9455185755993178454, 0.000000000000000000, -0.3255681544571537578 ) ) ;
#99988=EDGE_LOOP ( 'NONE', ( #40002, #45143, #86321, #92071, #107499, #45872 ) ) ;
#100003=FACE_BOUND ( 'NONE', #7660, .T. ) ;
#100060=VECTOR ( 'NONE', #37443, 1000.000000000000000 ) ;
#100070=EDGE_LOOP ( 'NONE', ( #37727, #66341 ) ) ;
#100077=CARTESIAN_POINT ( 'NONE',  ( -3.272667022753710242, 1519.551704408389924, 189.0363362235078171 ) ) ;
#100099=CARTESIAN_POINT ( 'NONE',  ( 21.60894078433416610, 1521.951704408389787, 218.5714488934191309 ) ) ;
#100116=ADVANCED_FACE ( 'NONE', ( #54283 ), #11701, .F. ) ;
#100127=AXIS2_PLACEMENT_3D ( 'NONE', #74191, #108871, #100466 ) ;
#100160=CARTESIAN_POINT ( 'NONE',  ( -2.562340869413346489, 1517.051704408389924, 196.2891841806521711 ) ) ;
#100164=CIRCLE ( 'NONE', #30464, 1.999999999999999556 ) ;
#100175=CYLINDRICAL_SURFACE ( 'NONE', #44465, 2.000000000000003553 ) ;
#100187=ORIENTED_EDGE ( 'NONE', *, *, #57143, .T. ) ;
#100192=ORIENTED_EDGE ( 'NONE', *, *, #45332, .T. ) ;
#100195=EDGE_CURVE ( 'NONE', #3770, #78370, #30137, .T. ) ;
#100229=AXIS2_PLACEMENT_3D ( 'NONE', #92195, #15468, #30438 ) ;
#100241=DIRECTION ( 'NONE',  ( -0.9455185755993178454, 0.000000000000000000, 0.3255681544571537578 ) ) ;
#100323=CARTESIAN_POINT ( 'NONE',  ( -8.486023334060130097, 1522.051704408389924, 211.0297173932031569 ) ) ;
#100344=CIRCLE ( 'NONE', #89545, 1.999999999999998668 ) ;
#100346=VERTEX_POINT ( 'NONE', #87036 ) ;
#100365=DIRECTION ( 'NONE',  ( 1.755985294532469921E-16, -1.000000000000000000, 1.338183447452831989E-16 ) ) ;
#100396=LINE ( 'NONE', #41602, #107360 ) ;
#100466=DIRECTION ( 'NONE',  ( -0.6736849260863841948, 0.000000000000000000, 0.7390186874254148774 ) ) ;
#100544=VERTEX_POINT ( 'NONE', #96550 ) ;
#100556=FACE_BOUND ( 'NONE', #76084, .T. ) ;
#100629=DIRECTION ( 'NONE',  ( 0.9455185755993177343, 0.000000000000000000, -0.3255681544571540909 ) ) ;
#100643=ORIENTED_EDGE ( 'NONE', *, *, #63306, .F. ) ;
#100662=ORIENTED_EDGE ( 'NONE', *, *, #77661, .F. ) ;
#100663=LINE ( 'NONE', #74949, #41360 ) ;
#100709=DIRECTION ( 'NONE',  ( -0.9455185755993178454, 0.000000000000000000, 0.3255681544571539243 ) ) ;
#100711=DIRECTION ( 'NONE',  ( -0.6736849260863841948, 0.000000000000000000, 0.7390186874254148774 ) ) ;
#100731=DIRECTION ( 'NONE',  ( 1.755985294532464991E-16, -1.000000000000000000, 1.338183447452830017E-16 ) ) ;
#100754=DIRECTION ( 'NONE',  ( -1.755985294532469921E-16, 1.000000000000000000, -1.338183447452831989E-16 ) ) ;
#100790=FACE_OUTER_BOUND ( 'NONE', #11379, .T. ) ;
#100853=ORIENTED_EDGE ( 'NONE', *, *, #37161, .F. ) ;
#100876=LINE ( 'NONE', #49409, #74324 ) ;
#100899=EDGE_CURVE ( 'NONE', #86629, #107071, #106932, .T. ) ;
#101016=AXIS2_PLACEMENT_3D ( 'NONE', #11250, #36977, #44300 ) ;
#101027=LINE ( 'NONE', #66372, #68848 ) ;
#101038=LINE ( 'NONE', #57970, #103795 ) ;
#101039=CARTESIAN_POINT ( 'NONE',  ( 17.71193101166619854, 1522.051704408389924, 196.6727161458730109 ) ) ;
#101044=EDGE_LOOP ( 'NONE', ( #24312, #41506 ) ) ;
#101082=EDGE_LOOP ( 'NONE', ( #93393, #13213, #110125, #46269, #51253 ) ) ;
#101094=FACE_BOUND ( 'NONE', #6617, .T. ) ;
#101117=VERTEX_POINT ( 'NONE', #85100 ) ;
#101185=CARTESIAN_POINT ( 'NONE',  ( -1.376928043298436100, 1517.151704408390060, 226.4861182474958525 ) ) ;
#101188=ORIENTED_EDGE ( 'NONE', *, *, #104765, .T. ) ;
#101208=VERTEX_POINT ( 'NONE', #92392 ) ;
#101257=ORIENTED_EDGE ( 'NONE', *, *, #83249, .T. ) ;
#101278=ADVANCED_FACE ( 'NONE', ( #88848 ), #21062, .F. ) ;
#101310=ADVANCED_FACE ( 'NONE', ( #93244 ), #16510, .F. ) ;
#101339=DIRECTION ( 'NONE',  ( -0.9455185755993178454, 0.000000000000000000, 0.3255681544571537578 ) ) ;
#101349=DIRECTION ( 'NONE',  ( 1.755985294532469921E-16, -1.000000000000000000, 1.338183447452831989E-16 ) ) ;
#101409=ORIENTED_EDGE ( 'NONE', *, *, #29046, .F. ) ;
#101444=CARTESIAN_POINT ( 'NONE',  ( 15.69795926444620271, 1519.551704408389924, 222.7678737639049871 ) ) ;
#101474=DIRECTION ( 'NONE',  ( 5.980589973904019347E-17, -1.000000000000000000, 1.736889445713099699E-16 ) ) ;
#101508=AXIS2_PLACEMENT_3D ( 'NONE', #89516, #30710, #46987 ) ;
#101511=FACE_BOUND ( 'NONE', #67296, .T. ) ;
#101541=CIRCLE ( 'NONE', #60495, 1.999999999999999556 ) ;
#101561=VECTOR ( 'NONE', #30678, 1000.000000000000114 ) ;
#101563=DIRECTION ( 'NONE',  ( -0.9455185755993178454, 0.000000000000000000, 0.3255681544571539243 ) ) ;
#101571=AXIS2_PLACEMENT_3D ( 'NONE', #13656, #39445, #48414 ) ;
#101578=ORIENTED_EDGE ( 'NONE', *, *, #25456, .F. ) ;
#101591=CIRCLE ( 'NONE', #46259, 1.999999999999998668 ) ;
#101673=DIRECTION ( 'NONE',  ( -1.755985294532469921E-16, 1.000000000000000000, -1.338183447452831989E-16 ) ) ;
#101686=EDGE_LOOP ( 'NONE', ( #73283, #74156, #26682, #91511, #82836 ) ) ;
#101694=AXIS2_PLACEMENT_3D ( 'NONE', #87693, #53546, #79842 ) ;
#101749=CARTESIAN_POINT ( 'NONE',  ( 17.68237282055029880, 1517.151704408390060, 212.5589510568480023 ) ) ;
#101750=AXIS2_PLACEMENT_3D ( 'NONE', #67096, #91717, #13890 ) ;
#101801=CYLINDRICAL_SURFACE ( 'NONE', #66291, 1.999999999999999556 ) ;
#101804=CIRCLE ( 'NONE', #76819, 2.000000000000002220 ) ;
#101821=DIRECTION ( 'NONE',  ( -5.980589973904019347E-17, 1.000000000000000000, -1.736889445713099699E-16 ) ) ;
#101833=ORIENTED_EDGE ( 'NONE', *, *, #39442, .F. ) ;
#101839=CIRCLE ( 'NONE', #85793, 1.999999999999999556 ) ;
#101863=AXIS2_PLACEMENT_3D ( 'NONE', #55189, #73638, #89314 ) ;
#101875=VECTOR ( 'NONE', #95087, 1000.000000000000000 ) ;
#101887=ORIENTED_EDGE ( 'NONE', *, *, #53555, .T. ) ;
#101935=EDGE_LOOP ( 'NONE', ( #53812, #50210 ) ) ;
#101959=ORIENTED_EDGE ( 'NONE', *, *, #50822, .T. ) ;
#101964=AXIS2_PLACEMENT_3D ( 'NONE', #73571, #57331, #22004 ) ;
#101968=DIRECTION ( 'NONE',  ( -5.980589973904019347E-17, 1.000000000000000000, -1.736889445713099699E-16 ) ) ;
#102043=CIRCLE ( 'NONE', #78906, 1.999999999999997780 ) ;
#102074=DIRECTION ( 'NONE',  ( 0.000000000000000000, -1.338183447452830017E-16, -1.000000000000000000 ) ) ;
#102115=VERTEX_POINT ( 'NONE', #18485 ) ;
#102131=EDGE_CURVE ( 'NONE', #95431, #65868, #98066, .T. ) ;
#102140=VERTEX_POINT ( 'NONE', #27456 ) ;
#102164=ADVANCED_FACE ( 'NONE', ( #77328 ), #53240, .F. ) ;
#102178=DIRECTION ( 'NONE',  ( -1.755985294532469921E-16, 1.000000000000000000, -1.338183447452831989E-16 ) ) ;
#102185=AXIS2_PLACEMENT_3D ( 'NONE', #103276, #26583, #110048 ) ;
#102284=EDGE_LOOP ( 'NONE', ( #92277, #48434, #22606, #19619 ) ) ;
#102307=DIRECTION ( 'NONE',  ( -5.980589973904019347E-17, 1.000000000000000000, -1.736889445713099699E-16 ) ) ;
#102313=CARTESIAN_POINT ( 'NONE',  ( 17.68237282055029880, 1522.051704408389924, 212.5589510568480023 ) ) ;
#102319=ADVANCED_FACE ( 'NONE', ( #7766 ), #100175, .F. ) ;
#102322=EDGE_LOOP ( 'NONE', ( #84124, #20346 ) ) ;
#102334=DIRECTION ( 'NONE',  ( -5.980589973904019347E-17, 1.000000000000000000, -1.736889445713099699E-16 ) ) ;
#102343=ORIENTED_EDGE ( 'NONE', *, *, #42389, .F. ) ;
#102384=CARTESIAN_POINT ( 'NONE',  ( 1.317811661047101568, 1517.051704408389924, 223.5300434977941677 ) ) ;
#102386=ORIENTED_EDGE ( 'NONE', *, *, #62419, .F. ) ;
#102397=ORIENTED_EDGE ( 'NONE', *, *, #63863, .T. ) ;
#102400=CARTESIAN_POINT ( 'NONE',  ( 15.69795926888880189, 1521.951704408389787, 222.7678737654429995 ) ) ;
#102413=CARTESIAN_POINT ( 'NONE',  ( -0.5779273184081697989, 1517.151704408390060, 186.0802614738061607 ) ) ;
#102468=EDGE_CURVE ( 'NONE', #86629, #9574, #14503, .T. ) ;
#102486=DIRECTION ( 'NONE',  ( -1.755985294532469921E-16, 1.000000000000000000, -1.338183447452831989E-16 ) ) ;
#102489=EDGE_LOOP ( 'NONE', ( #83369, #2115, #79483, #43454, #3264 ) ) ;
#102554=DIRECTION ( 'NONE',  ( -5.980589973904019347E-17, 1.000000000000000000, -1.736889445713099699E-16 ) ) ;
#102567=CYLINDRICAL_SURFACE ( 'NONE', #108929, 2.000000000000001332 ) ;
#102589=CARTESIAN_POINT ( 'NONE',  ( 9.803834995107230554, 1522.051704408389924, 221.6221720662910002 ) ) ;
#102610=FACE_BOUND ( 'NONE', #17745, .T. ) ;
#102628=DIRECTION ( 'NONE',  ( -0.6736849260863841948, 0.000000000000000000, 0.7390186874254148774 ) ) ;
#102649=ORIENTED_EDGE ( 'NONE', *, *, #2971, .F. ) ;
#102677=ORIENTED_EDGE ( 'NONE', *, *, #110075, .F. ) ;
#102770=CARTESIAN_POINT ( 'NONE',  ( -1.997114497637953345, 1517.051704408389924, 229.8748770088220965 ) ) ;
#102846=EDGE_CURVE ( 'NONE', #19461, #98304, #10555, .T. ) ;
#102852=FACE_OUTER_BOUND ( 'NONE', #22915, .T. ) ;
#102896=CIRCLE ( 'NONE', #36742, 1.999999999999999556 ) ;
#102929=CARTESIAN_POINT ( 'NONE',  ( 20.98459803409886959, 1519.551704408389924, 216.7582258867871587 ) ) ;
#102937=VERTEX_POINT ( 'NONE', #34117 ) ;
#102943=EDGE_CURVE ( 'NONE', #75707, #21719, #52042, .T. ) ;
#102964=ADVANCED_FACE ( 'NONE', ( #87859 ), #20071, .F. ) ;
#102998=DIRECTION ( 'NONE',  ( -5.980589973904019347E-17, 1.000000000000000000, -1.736889445713099699E-16 ) ) ;
#103034=CARTESIAN_POINT ( 'NONE',  ( -10.10023367162169983, 1522.051704408389924, 185.1638560673330005 ) ) ;
#103134=ORIENTED_EDGE ( 'NONE', *, *, #27274, .F. ) ;
#103149=CARTESIAN_POINT ( 'NONE',  ( -13.16517659032117038, 1517.151704408390060, 224.1947148507618408 ) ) ;
#103191=CARTESIAN_POINT ( 'NONE',  ( 13.10606020890036838, 1519.551704408389924, 225.8214468947291493 ) ) ;
#103193=VERTEX_POINT ( 'NONE', #91405 ) ;
#103201=CIRCLE ( 'NONE', #110323, 1.999999999999999556 ) ;
#103244=DIRECTION ( 'NONE',  ( 1.755985294532464991E-16, -1.000000000000000000, 1.338183447452830017E-16 ) ) ;
#103276=CARTESIAN_POINT ( 'NONE',  ( -5.864566082395439750, 1517.051704408389924, 192.0899093523580063 ) ) ;
#103300=VERTEX_POINT ( 'NONE', #57277 ) ;
#103301=ORIENTED_EDGE ( 'NONE', *, *, #70106, .T. ) ;
#103365=EDGE_CURVE ( 'NONE', #25738, #79870, #66227, .T. ) ;
#103377=CARTESIAN_POINT ( 'NONE',  ( 7.891238774076772877, 1519.551704408389924, 189.5145166091761553 ) ) ;
#103378=CARTESIAN_POINT ( 'NONE',  ( 15.69795926444620271, 1517.151704408390060, 222.7678737639049871 ) ) ;
#103394=VERTEX_POINT ( 'NONE', #68979 ) ;
#103400=CARTESIAN_POINT ( 'NONE',  ( 17.71193101166619854, 1522.051704408389924, 196.6727161458730109 ) ) ;
#103423=CARTESIAN_POINT ( 'NONE',  ( -10.41132050640262996, 1517.151704408390060, 189.4661702785461728 ) ) ;
#103431=AXIS2_PLACEMENT_3D ( 'NONE', #32010, #23603, #7360 ) ;
#103439=CARTESIAN_POINT ( 'NONE',  ( 21.01415622463856891, 1522.051704408389924, 200.8719909741391803 ) ) ;
#103457=LINE ( 'NONE', #26763, #60560 ) ;
#103463=DIRECTION ( 'NONE',  ( -5.980589973904019347E-17, 1.000000000000000000, -1.736889445713099699E-16 ) ) ;
#103491=AXIS2_PLACEMENT_3D ( 'NONE', #71573, #89968, #96171 ) ;
#103525=DIRECTION ( 'NONE',  ( -0.9455185755993178454, 0.000000000000000000, 0.3255681544571537578 ) ) ;
#103543=EDGE_CURVE ( 'NONE', #99156, #96293, #66637, .T. ) ;
#103559=VECTOR ( 'NONE', #57633, 1000.000000000000000 ) ;
#103577=LINE ( 'NONE', #26879, #66939 ) ;
#103584=CARTESIAN_POINT ( 'NONE',  ( -7.848979634317430509, 1517.051704408389924, 202.2988320601959913 ) ) ;
#103589=ADVANCED_FACE ( 'NONE', ( #105181 ), #104622, .F. ) ;
#103613=ORIENTED_EDGE ( 'NONE', *, *, #23746, .T. ) ;
#103646=ORIENTED_EDGE ( 'NONE', *, *, #19379, .F. ) ;
#103651=VECTOR ( 'NONE', #15008, 1000.000000000000000 ) ;
#103678=EDGE_LOOP ( 'NONE', ( #96729, #28501 ) ) ;
#103731=EDGE_CURVE ( 'NONE', #13291, #69131, #73230, .T. ) ;
#103740=AXIS2_PLACEMENT_3D ( 'NONE', #52528, #86660, #36263 ) ;
#103746=SURFACE_STYLE_USAGE ( .BOTH. , #69624 ) ;
#103795=VECTOR ( 'NONE', #16469, 1000.000000000000000 ) ;
#103862=ORIENTED_EDGE ( 'NONE', *, *, #54949, .F. ) ;
#103868=DIRECTION ( 'NONE',  ( -0.6736849260863841948, 0.000000000000000000, 0.7390186874254148774 ) ) ;
#103974=LINE ( 'NONE', #52491, #44881 ) ;
#103983=EDGE_LOOP ( 'NONE', ( #45217, #55091 ) ) ;
#103986=DIRECTION ( 'NONE',  ( -1.755985294532469921E-16, 1.000000000000000000, -1.338183447452831989E-16 ) ) ;
#104013=FACE_OUTER_BOUND ( 'NONE', #50365, .T. ) ;
#104034=CARTESIAN_POINT ( 'NONE',  ( -11.81780673814840021, 1517.151704408390060, 222.7166774759110126 ) ) ;
#104105=AXIS2_PLACEMENT_3D ( 'NONE', #65822, #107251, #55222 ) ;
#104130=DIRECTION ( 'NONE',  ( 0.9858563016923833633, 0.000000000000000000, 0.1675928173085483863 ) ) ;
#104143=ORIENTED_EDGE ( 'NONE', *, *, #104265, .T. ) ;
#104205=DIRECTION ( 'NONE',  ( 5.980589973904019347E-17, -1.000000000000000000, 1.736889445713099699E-16 ) ) ;
#104235=CARTESIAN_POINT ( 'NONE',  ( 0.3255681544576509712, 1547.051704408389924, 210.0673645372983174 ) ) ;
#104265=EDGE_CURVE ( 'NONE', #75704, #71877, #49288, .T. ) ;
#104291=DIRECTION ( 'NONE',  ( 1.755985294532464991E-16, -1.000000000000000000, 1.338183447452830017E-16 ) ) ;
#104294=FACE_OUTER_BOUND ( 'NONE', #82920, .T. ) ;
#104305=ORIENTED_EDGE ( 'NONE', *, *, #93379, .T. ) ;
#104309=DIRECTION ( 'NONE',  ( -1.755985294532469921E-16, 1.000000000000000000, -1.338183447452831989E-16 ) ) ;
#104324=ORIENTED_EDGE ( 'NONE', *, *, #21536, .F. ) ;
#104414=VERTEX_POINT ( 'NONE', #30122 ) ;
#104420=AXIS2_PLACEMENT_3D ( 'NONE', #49121, #65926, #32836 ) ;
#104427=DIRECTION ( 'NONE',  ( -5.980589973904019347E-17, 1.000000000000000000, -1.736889445713099699E-16 ) ) ;
#104447=ORIENTED_EDGE ( 'NONE', *, *, #88720, .F. ) ;
#104451=ORIENTED_EDGE ( 'NONE', *, *, #31807, .T. ) ;
#104462=DIRECTION ( 'NONE',  ( 0.9455185755993177343, 0.000000000000000000, -0.3255681544571540909 ) ) ;
#104468=ORIENTED_EDGE ( 'NONE', *, *, #90745, .F. ) ;
#104529=CARTESIAN_POINT ( 'NONE',  ( -1.925297167936410148, 1517.051704408389924, 187.5582988455250018 ) ) ;
#104547=VERTEX_POINT ( 'NONE', #54805 ) ;
#104572=CYLINDRICAL_SURFACE ( 'NONE', #68036, 2.000000000000003109 ) ;
#104582=VERTEX_POINT ( 'NONE', #29045 ) ;
#104584=VERTEX_POINT ( 'NONE', #72705 ) ;
#104622=CYLINDRICAL_SURFACE ( 'NONE', #33806, 1.999999999999999556 ) ;
#104652=ORIENTED_EDGE ( 'NONE', *, *, #9699, .F. ) ;
#104717=EDGE_CURVE ( 'NONE', #48781, #64960, #55911, .T. ) ;
#104765=EDGE_CURVE ( 'NONE', #58053, #50989, #101804, .T. ) ;
#104786=CARTESIAN_POINT ( 'NONE',  ( -11.75869035857540013, 1519.551704408389924, 190.9442076533970010 ) ) ;
#104829=AXIS2_PLACEMENT_3D ( 'NONE', #81195, #45973, #97461 ) ;
#104836=ADVANCED_FACE ( 'NONE', ( #42955 ), #45178, .F. ) ;
#104875=EDGE_LOOP ( 'NONE', ( #17597, #59586, #52627, #45405, #60694 ) ) ;
#104892=DIRECTION ( 'NONE',  ( -1.755985294532469921E-16, 1.000000000000000000, -1.338183447452831989E-16 ) ) ;
#104915=DIRECTION ( 'NONE',  ( -1.755985294532469921E-16, 1.000000000000000000, -1.338183447452831989E-16 ) ) ;
#104918=FACE_OUTER_BOUND ( 'NONE', #68255, .T. ) ;
#104979=AXIS2_PLACEMENT_3D ( 'NONE', #101444, #18000, #42672 ) ;
#105058=CYLINDRICAL_SURFACE ( 'NONE', #69320, 2.000000000000003109 ) ;
#105060=AXIS2_PLACEMENT_3D ( 'NONE', #81929, #4149, #64064 ) ;
#105099=DIRECTION ( 'NONE',  ( -5.980589973904019347E-17, 1.000000000000000000, -1.736889445713099699E-16 ) ) ;
#105123=DIRECTION ( 'NONE',  ( -0.6736849260863841948, 0.000000000000000000, 0.7390186874254148774 ) ) ;
#105143=CIRCLE ( 'NONE', #85446, 1.999999999999997780 ) ;
#105148=ORIENTED_EDGE ( 'NONE', *, *, #33180, .F. ) ;
#105154=CARTESIAN_POINT ( 'NONE',  ( 8.456465142934460388, 1517.051704408389924, 223.1002094411418284 ) ) ;
#105158=DIRECTION ( 'NONE',  ( -1.755985294532469921E-16, 1.000000000000000000, -1.338183447452831989E-16 ) ) ;
#105161=VERTEX_POINT ( 'NONE', #45057 ) ;
#105162=VERTEX_POINT ( 'NONE', #70271 ) ;
#105181=FACE_OUTER_BOUND ( 'NONE', #96711, .T. ) ;
#105183=DIRECTION ( 'NONE',  ( 0.9455185755993178454, 0.000000000000000000, -0.3255681544571538688 ) ) ;
#105196=EDGE_LOOP ( 'NONE', ( #47747, #31743, #81733, #73628 ) ) ;
#105199=VECTOR ( 'NONE', #64328, 1000.000000000000000 ) ;
#105204=AXIS2_PLACEMENT_3D ( 'NONE', #64934, #91759, #41376 ) ;
#105213=ORIENTED_EDGE ( 'NONE', *, *, #78055, .F. ) ;
#105219=( GEOMETRIC_REPRESENTATION_CONTEXT ( 3 ) GLOBAL_UNCERTAINTY_ASSIGNED_CONTEXT ( ( #16604 ) ) GLOBAL_UNIT_ASSIGNED_CONTEXT ( ( #86941, #35999, #87510 ) ) REPRESENTATION_CONTEXT ( 'NONE', 'WORKASPACE' ) );
#105291=AXIS2_PLACEMENT_3D ( 'NONE', #56692, #38224, #80793 ) ;
#105292=CARTESIAN_POINT ( 'NONE',  ( -1.376928043298434767, 1522.051704408389924, 226.4861182474958525 ) ) ;
#105293=CARTESIAN_POINT ( 'NONE',  ( -0.02955819112566620069, 1517.151704408390060, 225.0080808726450243 ) ) ;
#105360=CARTESIAN_POINT ( 'NONE',  ( 15.69795926888880189, 1521.951704408389787, 222.7678737654429995 ) ) ;
#105379=CIRCLE ( 'NONE', #101750, 3.999999999999997335 ) ;
#105388=DIRECTION ( 'NONE',  ( -1.755985294532469921E-16, 1.000000000000000000, -1.338183447452831989E-16 ) ) ;
#105390=CARTESIAN_POINT ( 'NONE',  ( -8.486023334060128320, 1517.151704408390060, 211.0297173932031569 ) ) ;
#105409=CIRCLE ( 'NONE', #80390, 2.000000000000003553 ) ;
#105412=EDGE_LOOP ( 'NONE', ( #65506, #68006, #62001, #42789 ) ) ;
#105430=CARTESIAN_POINT ( 'NONE',  ( 14.35058941227343254, 1522.051704408389924, 224.2459111387558437 ) ) ;
#105475=DIRECTION ( 'NONE',  ( 0.9455185755993177343, 0.000000000000000000, -0.3255681544571540909 ) ) ;
#105500=DIRECTION ( 'NONE',  ( 5.980589973904019347E-17, -1.000000000000000000, 1.736889445713099699E-16 ) ) ;
#105538=CIRCLE ( 'NONE', #16137, 3.999999999999997335 ) ;
#105548=VERTEX_POINT ( 'NONE', #25588 ) ;
#105557=CIRCLE ( 'NONE', #1822, 1.999999999999998668 ) ;
#105559=DIRECTION ( 'NONE',  ( -0.9455185755993177343, 0.000000000000000000, 0.3255681544571540909 ) ) ;
#105561=( NAMED_UNIT ( * ) PLANE_ANGLE_UNIT ( ) SI_UNIT ( $, .RADIAN. ) );
#105570=ORIENTED_EDGE ( 'NONE', *, *, #88720, .T. ) ;
#105576=EDGE_CURVE ( 'NONE', #33799, #76035, #60779, .T. ) ;
#105611=ADVANCED_FACE ( 'NONE', ( #5646 ), #99122, .F. ) ;
#105613=CARTESIAN_POINT ( 'NONE',  ( 9.225907677606100421, 1517.151704408390060, 198.5805875773771731 ) ) ;
#105626=VERTEX_POINT ( 'NONE', #58672 ) ;
#105629=CARTESIAN_POINT ( 'NONE',  ( -19.68364361186289813, 1519.551704408389924, 221.2357901434498615 ) ) ;
#105646=DIRECTION ( 'NONE',  ( -0.6736849260863837507, 0.000000000000000000, 0.7390186874254154326 ) ) ;
#105649=DIRECTION ( 'NONE',  ( -1.755985294532469921E-16, 1.000000000000000000, -1.338183447452831989E-16 ) ) ;
#105665=AXIS2_PLACEMENT_3D ( 'NONE', #40806, #15030, #23982 ) ;
#105799=ORIENTED_EDGE ( 'NONE', *, *, #12007, .F. ) ;
#105813=VECTOR ( 'NONE', #54126, 1000.000000000000000 ) ;
#105844=ORIENTED_EDGE ( 'NONE', *, *, #93976, .F. ) ;
#105847=CARTESIAN_POINT ( 'NONE',  ( 19.63722818094939981, 1517.051704408389924, 218.2362632588020119 ) ) ;
#105920=CYLINDRICAL_SURFACE ( 'NONE', #9841, 2.000000000000003553 ) ;
#105921=DIRECTION ( 'NONE',  ( 5.980589973904019347E-17, -1.000000000000000000, 1.736889445713099699E-16 ) ) ;
#105958=DIRECTION ( 'NONE',  ( -1.755985294532469921E-16, 1.000000000000000000, -1.338183447452831989E-16 ) ) ;
#105969=CIRCLE ( 'NONE', #91643, 1.999999999999998668 ) ;
#105994=ORIENTED_EDGE ( 'NONE', *, *, #108679, .F. ) ;
#105998=CYLINDRICAL_SURFACE ( 'NONE', #18814, 2.000000000000003553 ) ;
#106032=ORIENTED_EDGE ( 'NONE', *, *, #79455, .F. ) ;
#106040=CARTESIAN_POINT ( 'NONE',  ( -17.04532912216366825, 1522.051704408389924, 196.9538555332918293 ) ) ;
#106055=CARTESIAN_POINT ( 'NONE',  ( 14.35058941227343077, 1517.151704408390060, 224.2459111387558437 ) ) ;
#106077=DIRECTION ( 'NONE',  ( 5.980589973904019347E-17, -1.000000000000000000, 1.736889445713099699E-16 ) ) ;
#106157=AXIS2_PLACEMENT_3D ( 'NONE', #56006, #100731, #90130 ) ;
#106209=CARTESIAN_POINT ( 'NONE',  ( -23.59335433706185015, 1519.551704408389924, 209.8811657366039185 ) ) ;
#106228=EDGE_CURVE ( 'NONE', #47709, #35907, #59004, .T. ) ;
#106237=VECTOR ( 'NONE', #5179, 1000.000000000000000 ) ;
#106265=EDGE_CURVE ( 'NONE', #63893, #20461, #78657, .T. ) ;
#106291=LINE ( 'NONE', #31232, #30197 ) ;
#106306=VERTEX_POINT ( 'NONE', #74959 ) ;
#106323=EDGE_LOOP ( 'NONE', ( #93030, #70302 ) ) ;
#106381=CARTESIAN_POINT ( 'NONE',  ( -17.68237282055029880, 1517.051704408389924, 205.6847408665509818 ) ) ;
#106382=EDGE_CURVE ( 'NONE', #100544, #81391, #107259, .T. ) ;
#106440=CIRCLE ( 'NONE', #47381, 1.999999999999997780 ) ;
#106445=CARTESIAN_POINT ( 'NONE',  ( -11.18076303840566332, 1517.051704408389924, 213.9857921429048417 ) ) ;
#106492=CARTESIAN_POINT ( 'NONE',  ( -7.878537825433329367, 1517.151704408390060, 218.1850669711710111 ) ) ;
#106527=ORIENTED_EDGE ( 'NONE', *, *, #30221, .T. ) ;
#106538=DIRECTION ( 'NONE',  ( -0.6736849260863841948, 0.000000000000000000, 0.7390186874254148774 ) ) ;
#106565=CIRCLE ( 'NONE', #29412, 1.999999999999999556 ) ;
#106576=DIRECTION ( 'NONE',  ( 0.9455185755993178454, 0.000000000000000000, -0.3255681544571539243 ) ) ;
#106642=CARTESIAN_POINT ( 'NONE',  ( -0.04641543311909263059, 1519.551704408389924, 230.3502074419784265 ) ) ;
#106669=VERTEX_POINT ( 'NONE', #16254 ) ;
#106692=DIRECTION ( 'NONE',  ( -5.980589973904019347E-17, 1.000000000000000000, -1.736889445713099699E-16 ) ) ;
#106719=FACE_OUTER_BOUND ( 'NONE', #72123, .T. ) ;
#106800=FACE_OUTER_BOUND ( 'NONE', #104875, .T. ) ;
#106813=CARTESIAN_POINT ( 'NONE',  ( -11.15120484728000072, 1517.151704408390060, 198.0995572319588405 ) ) ;
#106846=CARTESIAN_POINT ( 'NONE',  ( 6.501609782144663896, 1522.051704408389924, 217.4228972380528262 ) ) ;
#106874=DIRECTION ( 'NONE',  ( -0.6736849260863841948, 0.000000000000000000, 0.7390186874254148774 ) ) ;
#106899=EDGE_CURVE ( 'NONE', #75707, #30117, #17867, .T. ) ;
#106921=DIRECTION ( 'NONE',  ( -0.9455185755993178454, 0.000000000000000000, 0.3255681544571537578 ) ) ;
#106930=CARTESIAN_POINT ( 'NONE',  ( 15.72751745975079984, 1517.051704408389924, 206.8816388537309763 ) ) ;
#106932=CIRCLE ( 'NONE', #13967, 2.000000000000003553 ) ;
#106953=CARTESIAN_POINT ( 'NONE',  ( 8.627556093114653990, 1521.551704408389696, 234.1780882150808623 ) ) ;
#106986=CARTESIAN_POINT ( 'NONE',  ( 13.74310390781900004, 1517.151704408390060, 217.0905615615409943 ) ) ;
#107012=EDGE_CURVE ( 'NONE', #86132, #108494, #40672, .T. ) ;
#107043=CARTESIAN_POINT ( 'NONE',  ( -3.331783404088238143, 1522.051704408389924, 220.8088060444078451 ) ) ;
#107051=LINE ( 'NONE', #79670, #19028 ) ;
#107071=VERTEX_POINT ( 'NONE', #94938 ) ;
#107074=ORIENTED_EDGE ( 'NONE', *, *, #65359, .T. ) ;
#107110=AXIS2_PLACEMENT_3D ( 'NONE', #41295, #109062, #100629 ) ;
#107136=CARTESIAN_POINT ( 'NONE',  ( -2.621457251404220035, 1517.151704408390060, 228.0616540033011574 ) ) ;
#107142=DIRECTION ( 'NONE',  ( 0.9455185755993178454, 0.000000000000000000, -0.3255681544571539243 ) ) ;
#107153=AXIS2_PLACEMENT_3D ( 'NONE', #31047, #65229, #96196 ) ;
#107170=CARTESIAN_POINT ( 'NONE',  ( 1.997114501359404048, 1521.951704408389787, 188.3688149103338958 ) ) ;
#107171=DIRECTION ( 'NONE',  ( -5.980589973904019347E-17, 1.000000000000000000, -1.736889445713099699E-16 ) ) ;
#107177=FACE_BOUND ( 'NONE', #23539, .T. ) ;
#107186=VECTOR ( 'NONE', #108969, 1000.000000000000000 ) ;
#107242=EDGE_LOOP ( 'NONE', ( #73636, #73492, #44374, #46207 ) ) ;
#107248=VECTOR ( 'NONE', #86540, 1000.000000000000000 ) ;
#107251=DIRECTION ( 'NONE',  ( -1.755985294532469921E-16, 1.000000000000000000, -1.338183447452831989E-16 ) ) ;
#107259=CIRCLE ( 'NONE', #10726, 1.999999999999997780 ) ;
#107298=EDGE_CURVE ( 'NONE', #77569, #17947, #71592, .T. ) ;
#107360=VECTOR ( 'NONE', #58956, 1000.000000000000000 ) ;
#107361=CARTESIAN_POINT ( 'NONE',  ( 3.968827103902559550, 1517.151704408390060, 188.7040005461919918 ) ) ;
#107380=DIRECTION ( 'NONE',  ( -5.980589973904019347E-17, 1.000000000000000000, -1.736889445713099699E-16 ) ) ;
#107382=CYLINDRICAL_SURFACE ( 'NONE', #17553, 2.000000000000003553 ) ;
#107384=ORIENTED_EDGE ( 'NONE', *, *, #709, .T. ) ;
#107458=DIRECTION ( 'NONE',  ( 1.755985294532464991E-16, -1.000000000000000000, 1.338183447452830017E-16 ) ) ;
#107470=ORIENTED_EDGE ( 'NONE', *, *, #59780, .F. ) ;
#107480=DIRECTION ( 'NONE',  ( 1.755985294532469921E-16, -1.000000000000000000, 1.338183447452831989E-16 ) ) ;
#107484=EDGE_CURVE ( 'NONE', #18655, #80453, #42927, .T. ) ;
#107493=EDGE_LOOP ( 'NONE', ( #39607, #44447, #54320, #31064 ) ) ;
#107498=ORIENTED_EDGE ( 'NONE', *, *, #68263, .T. ) ;
#107499=ORIENTED_EDGE ( 'NONE', *, *, #24066, .F. ) ;
#107534=CIRCLE ( 'NONE', #96846, 1.999999999999999556 ) ;
#107535=CARTESIAN_POINT ( 'NONE',  ( 9.862951377358559313, 1519.551704408389924, 189.8497022443989977 ) ) ;
#107539=DIRECTION ( 'NONE',  ( -0.9455185755993178454, 0.000000000000000000, 0.3255681544571539243 ) ) ;
#107551=CARTESIAN_POINT ( 'NONE',  ( -19.64992912988063267, 1521.951704408389787, 210.5515370059081022 ) ) ;
#107590=DIRECTION ( 'NONE',  ( -5.980589973904019347E-17, 1.000000000000000000, -1.736889445713099699E-16 ) ) ;
#107614=CIRCLE ( 'NONE', #41519, 2.000000000000003553 ) ;
#107664=ADVANCED_FACE ( 'NONE', ( #373 ), #50743, .F. ) ;
#107680=DIRECTION ( 'NONE',  ( -1.755985294532469921E-16, 1.000000000000000000, -1.338183447452831989E-16 ) ) ;
#107681=EDGE_CURVE ( 'NONE', #23279, #54088, #19736, .T. ) ;
#107732=FACE_BOUND ( 'NONE', #68359, .T. ) ;
#107746=EDGE_CURVE ( 'NONE', #58393, #36440, #98455, .T. ) ;
#107827=CARTESIAN_POINT ( 'NONE',  ( -2.694739704345536335, 1522.051704408389924, 212.0779207114006510 ) ) ;
#107854=DIRECTION ( 'NONE',  ( 0.3255681544571546460, 0.000000000000000000, 0.9455185755993176233 ) ) ;
#107894=EDGE_CURVE ( 'NONE', #81601, #52122, #35895, .T. ) ;
#107901=EDGE_LOOP ( 'NONE', ( #15916, #13901 ) ) ;
#107931=DIRECTION ( 'NONE',  ( -1.755985294532469921E-16, 1.000000000000000000, -1.338183447452831989E-16 ) ) ;
#107949=DIRECTION ( 'NONE',  ( 0.9455185755993178454, 0.000000000000000000, -0.3255681544571539243 ) ) ;
#107979=CARTESIAN_POINT ( 'NONE',  ( 1.925297169133120212, 1517.051704408389924, 230.6853930764029883 ) ) ;
#107985=DIRECTION ( 'NONE',  ( -0.6736849260863841948, 0.000000000000000000, 0.7390186874254148774 ) ) ;
#107990=ORIENTED_EDGE ( 'NONE', *, *, #88303, .T. ) ;
#108008=DIRECTION ( 'NONE',  ( 0.9455185755993178454, 0.000000000000000000, -0.3255681544571537578 ) ) ;
#108026=VERTEX_POINT ( 'NONE', #25321 ) ;
#108071=ORIENTED_EDGE ( 'NONE', *, *, #93387, .F. ) ;
#108083=DIRECTION ( 'NONE',  ( -0.6736849260863841948, 0.000000000000000000, 0.7390186874254148774 ) ) ;
#108089=CARTESIAN_POINT ( 'NONE',  ( -0.6370436997427022519, 1517.051704408389924, 217.8527312947061603 ) ) ;
#108145=AXIS2_PLACEMENT_3D ( 'NONE', #65523, #12493, #91251 ) ;
#108154=DIRECTION ( 'NONE',  ( 1.755985294532464991E-16, -1.000000000000000000, 1.338183447452830017E-16 ) ) ;
#108168=DIRECTION ( 'NONE',  ( 1.755985294532464991E-16, -1.000000000000000000, 1.338183447452830017E-16 ) ) ;
#108185=ORIENTED_EDGE ( 'NONE', *, *, #32610, .T. ) ;
#108203=CARTESIAN_POINT ( 'NONE',  ( 5.316196956075327051, 1522.051704408389924, 187.2259631713411636 ) ) ;
#108206=ORIENTED_EDGE ( 'NONE', *, *, #24196, .T. ) ;
#108253=DIRECTION ( 'NONE',  ( 1.755985294532464991E-16, -1.000000000000000000, 1.338183447452830017E-16 ) ) ;
#108261=EDGE_CURVE ( 'NONE', #56930, #55445, #75227, .T. ) ;
#108285=ADVANCED_FACE ( 'NONE', ( #67693 ), #101801, .F. ) ;
#108348=ADVANCED_FACE ( 'NONE', ( #2707 ), #45810, .F. ) ;
#108377=FACE_OUTER_BOUND ( 'NONE', #72269, .T. ) ;
#108395=CARTESIAN_POINT ( 'NONE',  ( -2.694739704345535891, 1517.051704408389924, 212.0779207114006510 ) ) ;
#108403=ORIENTED_EDGE ( 'NONE', *, *, #13079, .F. ) ;
#108406=CARTESIAN_POINT ( 'NONE',  ( -9.196349486490200675, 1517.051704408389924, 203.7768694350468195 ) ) ;
#108412=FACE_OUTER_BOUND ( 'NONE', #45125, .T. ) ;
#108416=FACE_BOUND ( 'NONE', #63257, .T. ) ;
#108433=CARTESIAN_POINT ( 'NONE',  ( -0.6370436997426996983, 1517.151704408390060, 217.8527312947061603 ) ) ;
#108456=DIRECTION ( 'NONE',  ( -0.3255681544571569219, -1.836970198721028948E-16, -0.9455185755993167351 ) ) ;
#108494=VERTEX_POINT ( 'NONE', #102770 ) ;
#108504=CARTESIAN_POINT ( 'NONE',  ( 2.359533070475779804E-16, 1517.051704408389924, 209.1218459616989946 ) ) ;
#108540=APPLICATION_CONTEXT ( 'automotive_design' ) ;
#108595=DIRECTION ( 'NONE',  ( 1.755985294532464991E-16, -1.000000000000000000, 1.338183447452830017E-16 ) ) ;
#108603=EDGE_LOOP ( 'NONE', ( #62589, #98464, #40770, #82487, #43049 ) ) ;
#108637=DIRECTION ( 'NONE',  ( -1.755985294532469921E-16, 1.000000000000000000, -1.338183447452831989E-16 ) ) ;
#108641=DIRECTION ( 'NONE',  ( -1.755985294532469921E-16, 1.000000000000000000, -1.338183447452831989E-16 ) ) ;
#108643=DIRECTION ( 'NONE',  ( -0.9455185755993177343, 0.000000000000000000, 0.3255681544571540909 ) ) ;
#108655=CARTESIAN_POINT ( 'NONE',  ( 9.862951377130659836, 1521.951704408389787, 189.8497022437369708 ) ) ;
#108656=ORIENTED_EDGE ( 'NONE', *, *, #45365, .T. ) ;
#108666=CYLINDRICAL_SURFACE ( 'NONE', #78552, 2.000000000000003109 ) ;
#108679=EDGE_CURVE ( 'NONE', #59011, #86431, #14368, .T. ) ;
#108681=ORIENTED_EDGE ( 'NONE', *, *, #39442, .T. ) ;
#108769=ORIENTED_EDGE ( 'NONE', *, *, #105576, .T. ) ;
#108790=AXIS2_PLACEMENT_3D ( 'NONE', #79179, #104915, #36064 ) ;
#108806=AXIS2_PLACEMENT_3D ( 'NONE', #25489, #104427, #45102 ) ;
#108818=ORIENTED_EDGE ( 'NONE', *, *, #59893, .F. ) ;
#108832=FACE_BOUND ( 'NONE', #81603, .T. ) ;
#108837=ORIENTED_EDGE ( 'NONE', *, *, #28233, .T. ) ;
#108850=( NAMED_UNIT ( * ) SI_UNIT ( $, .STERADIAN. ) SOLID_ANGLE_UNIT ( ) );
#108856=VERTEX_POINT ( 'NONE', #37809 ) ;
#108863=CIRCLE ( 'NONE', #98147, 1.999999999999999556 ) ;
#108867=AXIS2_PLACEMENT_3D ( 'NONE', #10675, #2299, #28010 ) ;
#108871=DIRECTION ( 'NONE',  ( 1.755985294532469921E-16, -1.000000000000000000, 1.338183447452831989E-16 ) ) ;
#108873=VECTOR ( 'NONE', #70523, 1000.000000000000000 ) ;
#108911=DIRECTION ( 'NONE',  ( -0.9455185755993178454, 0.000000000000000000, 0.3255681544571537578 ) ) ;
#108921=AXIS2_PLACEMENT_3D ( 'NONE', #99143, #5668, #39815 ) ;
#108925=EDGE_CURVE ( 'NONE', #21199, #81391, #73630, .T. ) ;
#108929=AXIS2_PLACEMENT_3D ( 'NONE', #86339, #43793, #109357 ) ;
#108935=DIRECTION ( 'NONE',  ( 0.9455185755993178454, 0.000000000000000000, -0.3255681544571537578 ) ) ;
#108939=EDGE_LOOP ( 'NONE', ( #106032, #78630, #109351, #9009 ) ) ;
#108953=CIRCLE ( 'NONE', #32056, 1.999999999999997780 ) ;
#108969=DIRECTION ( 'NONE',  ( 5.980589973904019347E-17, -1.000000000000000000, 1.736889445713099699E-16 ) ) ;
#108970=AXIS2_PLACEMENT_3D ( 'NONE', #8905, #27371, #10020 ) ;
#108971=CARTESIAN_POINT ( 'NONE',  ( 15.74021840827733598, 1519.551704408389924, 196.3375305112799936 ) ) ;
#108974=FACE_BOUND ( 'NONE', #90636, .T. ) ;
#108989=AXIS2_PLACEMENT_3D ( 'NONE', #53635, #28408, #45229 ) ;
#108996=ORIENTED_EDGE ( 'NONE', *, *, #77689, .F. ) ;
#108999=EDGE_LOOP ( 'NONE', ( #47090, #47181 ) ) ;
#109000=ORIENTED_EDGE ( 'NONE', *, *, #13707, .F. ) ;
#109014=VECTOR ( 'NONE', #65853, 1000.000000000000000 ) ;
#109025=EDGE_LOOP ( 'NONE', ( #16509, #65471 ) ) ;
#109062=DIRECTION ( 'NONE',  ( 1.755985294532464991E-16, -1.000000000000000000, 1.338183447452830017E-16 ) ) ;
#109078=ORIENTED_EDGE ( 'NONE', *, *, #110075, .T. ) ;
#109091=CARTESIAN_POINT ( 'NONE',  ( 5.940539708128937058, 1517.051704408389924, 189.0391861795680768 ) ) ;
#109097=AXIS2_PLACEMENT_3D ( 'NONE', #79536, #2301, #89015 ) ;
#109102=ORIENTED_EDGE ( 'NONE', *, *, #45994, .F. ) ;
#109148=EDGE_CURVE ( 'NONE', #8406, #70030, #95235, .T. ) ;
#109156=EDGE_LOOP ( 'NONE', ( #90598, #90818, #46227, #53187 ) ) ;
#109204=CARTESIAN_POINT ( 'NONE',  ( -12.39573405564623165, 1522.051704408389924, 199.6750929870061668 ) ) ;
#109229=CARTESIAN_POINT ( 'NONE',  ( 17.68237282055029880, 1517.051704408389924, 212.5589510568480023 ) ) ;
#109232=ORIENTED_EDGE ( 'NONE', *, *, #66618, .F. ) ;
#109267=AXIS2_PLACEMENT_3D ( 'NONE', #23853, #98921, #65901 ) ;
#109294=CIRCLE ( 'NONE', #37753, 1.999999999999999556 ) ;
#109309=DIRECTION ( 'NONE',  ( -1.755985294532469921E-16, 1.000000000000000000, -1.338183447452831989E-16 ) ) ;
#109317=AXIS2_PLACEMENT_3D ( 'NONE', #68054, #57450, #75346 ) ;
#109329=AXIS2_PLACEMENT_3D ( 'NONE', #78894, #79437, #86720 ) ;
#109338=ORIENTED_EDGE ( 'NONE', *, *, #29311, .T. ) ;
#109343=CARTESIAN_POINT ( 'NONE',  ( 1.984413551915469975, 1522.051704408389924, 198.9129232538419956 ) ) ;
#109351=ORIENTED_EDGE ( 'NONE', *, *, #65192, .T. ) ;
#109357=DIRECTION ( 'NONE',  ( 0.9858563016761853204, 0.000000000000000000, 0.1675928174038331386 ) ) ;
#109362=DIRECTION ( 'NONE',  ( -0.9455185755993178454, 0.000000000000000000, 0.3255681544571537578 ) ) ;
#109369=FACE_OUTER_BOUND ( 'NONE', #16658, .T. ) ;
#109380=CARTESIAN_POINT ( 'NONE',  ( 19.63722818192610120, 1519.551704408389924, 218.2362632616380154 ) ) ;
#109463=EDGE_LOOP ( 'NONE', ( #89904, #49541, #12275, #31168 ) ) ;
#109497=DIRECTION ( 'NONE',  ( 0.9455185755993178454, 0.000000000000000000, -0.3255681544571537578 ) ) ;
#109523=FACE_BOUND ( 'NONE', #45126, .T. ) ;
#109549=ORIENTED_EDGE ( 'NONE', *, *, #37214, .T. ) ;
#109601=EDGE_LOOP ( 'NONE', ( #24183, #27739, #23167, #51451, #84296 ) ) ;
#109640=ORIENTED_EDGE ( 'NONE', *, *, #12765, .F. ) ;
#109651=EDGE_CURVE ( 'NONE', #49504, #67084, #65528, .T. ) ;
#109670=DIRECTION ( 'NONE',  ( -1.755985294532469921E-16, 1.000000000000000000, -1.338183447452831989E-16 ) ) ;
#109714=DIRECTION ( 'NONE',  ( -1.755985294532469921E-16, 1.000000000000000000, -1.338183447452831989E-16 ) ) ;
#109746=EDGE_CURVE ( 'NONE', #72223, #41356, #66365, .T. ) ;
#109765=CARTESIAN_POINT ( 'NONE',  ( -17.71193100849139768, 1517.151704408390060, 221.5709757781449980 ) ) ;
#109777=CARTESIAN_POINT ( 'NONE',  ( -13.74310390781900004, 1517.051704408389924, 201.1531303618569950 ) ) ;
#109826=VERTEX_POINT ( 'NONE', #100077 ) ;
#109857=DIRECTION ( 'NONE',  ( 0.9455185755993178454, 0.000000000000000000, -0.3255681544571537578 ) ) ;
#109861=LINE ( 'NONE', #93584, #94258 ) ;
#109882=DIRECTION ( 'NONE',  ( 0.9455185755993178454, 0.000000000000000000, -0.3255681544571539243 ) ) ;
#109898=DIRECTION ( 'NONE',  ( 0.9455185755993177343, 0.000000000000000000, -0.3255681544571540909 ) ) ;
#109908=LINE ( 'NONE', #34296, #39970 ) ;
#109912=AXIS2_PLACEMENT_3D ( 'NONE', #35655, #60893, #87169 ) ;
#109920=DIRECTION ( 'NONE',  ( -1.755985294532469921E-16, 1.000000000000000000, -1.338183447452831989E-16 ) ) ;
#109924=EDGE_CURVE ( 'NONE', #48151, #68701, #102043, .T. ) ;
#109937=CARTESIAN_POINT ( 'NONE',  ( -4.517196230222677578, 1517.051704408389924, 190.6118719775071781 ) ) ;
#109941=FACE_OUTER_BOUND ( 'NONE', #30534, .T. ) ;
#109944=FACE_BOUND ( 'NONE', #85673, .T. ) ;
#109982=ADVANCED_FACE ( 'NONE', ( #7217 ), #5562, .F. ) ;
#110034=AXIS2_PLACEMENT_3D ( 'NONE', #51594, #66762, #74600 ) ;
#110038=LINE ( 'NONE', #24895, #1447 ) ;
#110048=DIRECTION ( 'NONE',  ( -0.9455185755993178454, 0.000000000000000000, 0.3255681544571539243 ) ) ;
#110072=DIRECTION ( 'NONE',  ( -1.755985294532469921E-16, 1.000000000000000000, -1.338183447452831989E-16 ) ) ;
#110075=EDGE_CURVE ( 'NONE', #41356, #22976, #31855, .T. ) ;
#110077=DIRECTION ( 'NONE',  ( -1.755985294532469921E-16, 1.000000000000000000, -1.338183447452831989E-16 ) ) ;
#110085=CARTESIAN_POINT ( 'NONE',  ( 0.000000000000000000, 0.000000000000000000, 0.000000000000000000 ) ) ;
#110096=CARTESIAN_POINT ( 'NONE',  ( 9.862951377358559313, 1522.051704408389924, 189.8497022443989977 ) ) ;
#110100=VERTEX_POINT ( 'NONE', #24259 ) ;
#110112=ORIENTED_EDGE ( 'NONE', *, *, #81848, .T. ) ;
#110113=LINE ( 'NONE', #34508, #15343 ) ;
#110125=ORIENTED_EDGE ( 'NONE', *, *, #106228, .F. ) ;
#110161=DIRECTION ( 'NONE',  ( 1.755985294532464991E-16, -1.000000000000000000, 1.338183447452830017E-16 ) ) ;
#110167=CYLINDRICAL_SURFACE ( 'NONE', #36630, 2.000000000000003553 ) ;
#110182=ORIENTED_EDGE ( 'NONE', *, *, #59709, .T. ) ;
#110193=FACE_OUTER_BOUND ( 'NONE', #41790, .T. ) ;
#110229=DIRECTION ( 'NONE',  ( -0.6736849260863841948, 0.000000000000000000, 0.7390186874254148774 ) ) ;
#110234=DIRECTION ( 'NONE',  ( -5.980589973904019347E-17, 1.000000000000000000, -1.736889445713099699E-16 ) ) ;
#110251=DIRECTION ( 'NONE',  ( 5.980589973904019347E-17, -1.000000000000000000, 1.736889445713099699E-16 ) ) ;
#110313=EDGE_LOOP ( 'NONE', ( #47835, #93799, #89739, #33906 ) ) ;
#110323=AXIS2_PLACEMENT_3D ( 'NONE', #6971, #41125, #75305 ) ;
#110377=ADVANCED_FACE ( 'NONE', ( #10092 ), #78408, .F. ) ;
#110436=VERTEX_POINT ( 'NONE', #12722 ) ;
#110461=EDGE_CURVE ( 'NONE', #43348, #93138, #75309, .T. ) ;
#110513=EDGE_LOOP ( 'NONE', ( #70669, #2052, #65675, #68212 ) ) ;
#110538=DIRECTION ( 'NONE',  ( 0.9858563016761853204, 0.000000000000000000, 0.1675928174038331386 ) ) ;
#110581=DIRECTION ( 'NONE',  ( 1.755985294532464991E-16, -1.000000000000000000, 1.338183447452830017E-16 ) ) ;
#110585=CARTESIAN_POINT ( 'NONE',  ( -10.10023367162169983, 1517.051704408389924, 185.1638560673330005 ) ) ;
#110594=EDGE_CURVE ( 'NONE', #55445, #95431, #57504, .T. ) ;
#110607=VERTEX_POINT ( 'NONE', #15999 ) ;
#110648=ORIENTED_EDGE ( 'NONE', *, *, #49297, .F. ) ;
#110692=DIRECTION ( 'NONE',  ( -0.6736849260863839728, 0.000000000000000000, 0.7390186874254150995 ) ) ;
#110694=VERTEX_POINT ( 'NONE', #66462 ) ;
#110714=DIRECTION ( 'NONE',  ( 0.9858563016923833633, 0.000000000000000000, 0.1675928173085483863 ) ) ;
#110735=ORIENTED_EDGE ( 'NONE', *, *, #99829, .F. ) ;
#110739=DIRECTION ( 'NONE',  ( 1.755985294532464991E-16, -1.000000000000000000, 1.338183447452830017E-16 ) ) ;
#110743=CARTESIAN_POINT ( 'NONE',  ( 7.211935934568218798, 1517.051704408389924, 224.6757451961901495 ) ) ;
#110772=EDGE_LOOP ( 'NONE', ( #44834, #35516 ) ) ;
#110808=DIRECTION ( 'NONE',  ( -0.9455185755993178454, 0.000000000000000000, 0.3255681544571539243 ) ) ;
ENDSEC;
END-ISO-10303-21;
